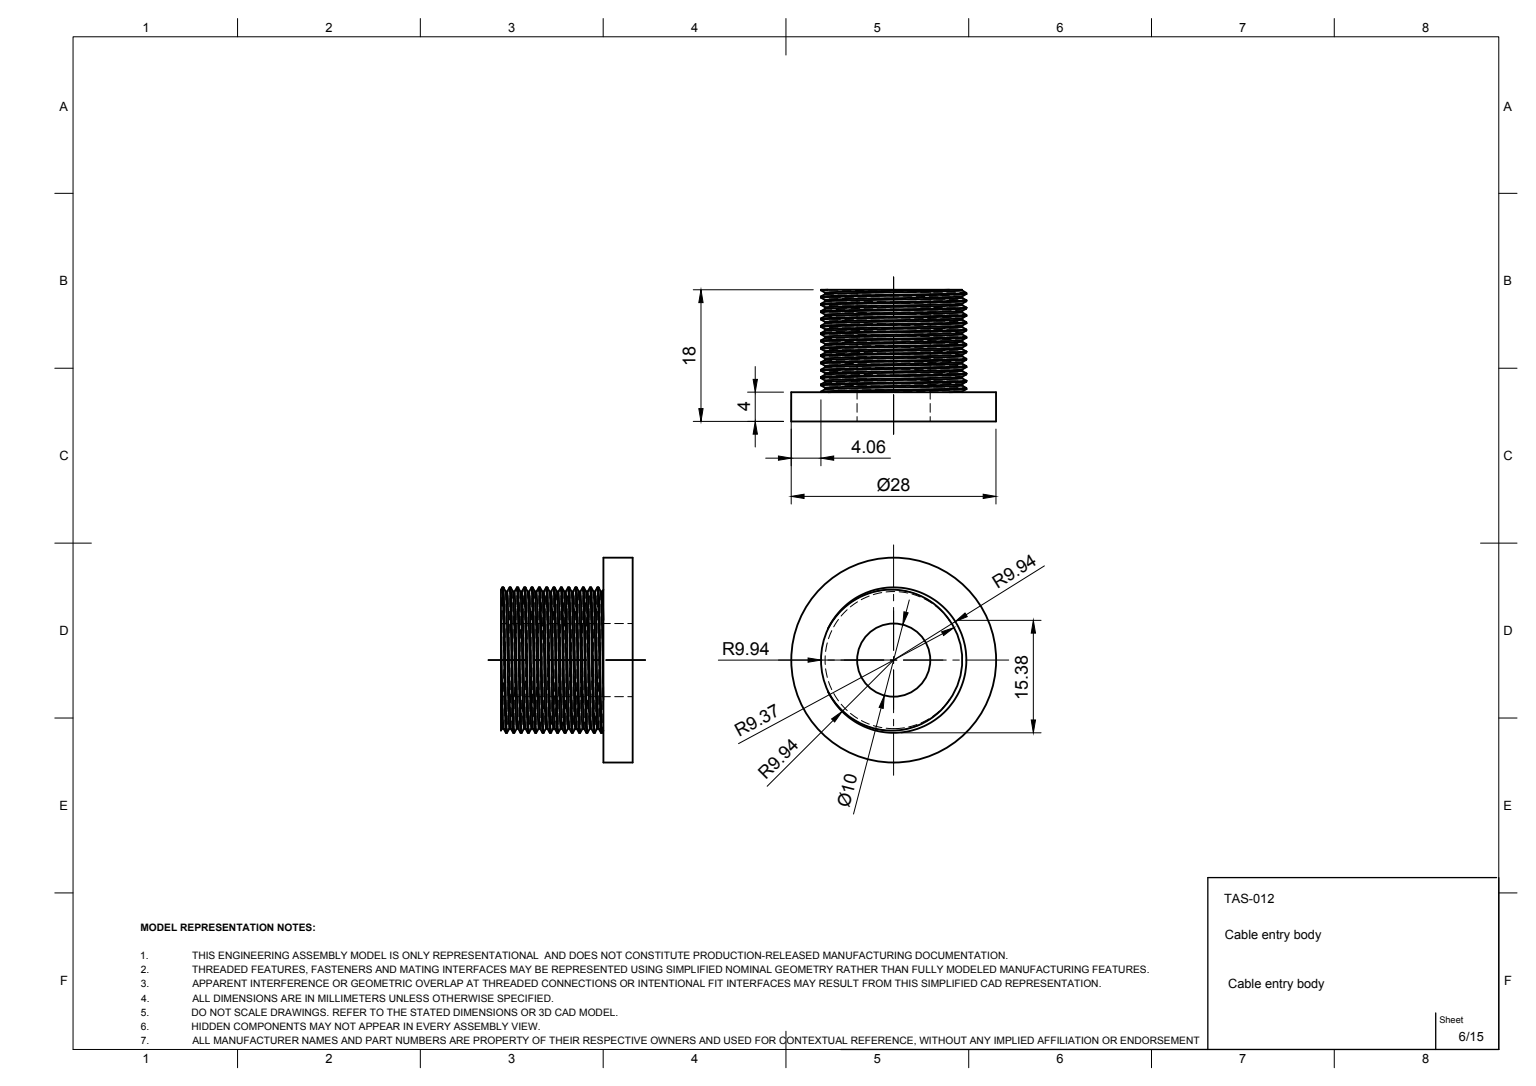
ISO-10303-21;
HEADER;
/* Generated by software containing ST-Developer
 * from STEP Tools, Inc. (www.steptools.com) 
 */

FILE_DESCRIPTION(
/* description */ (
'Independent welded steel electronics enclosure with removable sealed 
lid, internal mounting tray and two threaded cable entries. 300 x 220 
mm body. No ingress or electrical safety rating assigned.'),
/* implementation_level */ '2;1');

FILE_NAME(
/* name */ 'Cable entry body.step',
/* time_stamp */ '2026-11-14T09:13:27-08:00',
/* author */ (''),
/* organization */ (''),
/* preprocessor_version */ 'ST-DEVELOPER v20.2',
/* originating_system */ 'Autodesk Translation Framework v15.17.0.0',
/* authorisation */ '');

FILE_SCHEMA (('AUTOMOTIVE_DESIGN { 1 0 10303 214 3 1 1 }'));
ENDSEC;

DATA;
#10=MECHANICAL_DESIGN_GEOMETRIC_PRESENTATION_REPRESENTATION('',(#978),#94412);
#166=B_SPLINE_SURFACE_WITH_KNOTS('',3,3,((#89566,#89567,#89568,#89569,#89570,
#89571,#89572,#89573,#89574,#89575,#89576,#89577,#89578,#89579,#89580,#89581,
#89582,#89583,#89584,#89585,#89586,#89587,#89588,#89589,#89590,#89591,#89592,
#89593,#89594,#89595,#89596,#89597,#89598,#89599,#89600,#89601,#89602,#89603,
#89604,#89605,#89606,#89607,#89608,#89609,#89610,#89611,#89612,#89613,#89614,
#89615,#89616,#89617,#89618,#89619,#89620,#89621,#89622,#89623,#89624,#89625,
#89626,#89627,#89628,#89629,#89630,#89631,#89632,#89633,#89634,#89635,#89636,
#89637,#89638,#89639,#89640,#89641,#89642,#89643,#89644,#89645,#89646,#89647,
#89648,#89649,#89650,#89651,#89652,#89653,#89654,#89655,#89656,#89657,#89658,
#89659,#89660,#89661,#89662,#89663,#89664,#89665,#89666,#89667,#89668,#89669,
#89670,#89671,#89672,#89673,#89674,#89675,#89676,#89677,#89678,#89679,#89680,
#89681,#89682,#89683,#89684,#89685,#89686,#89687,#89688,#89689,#89690,#89691,
#89692,#89693,#89694,#89695,#89696,#89697,#89698,#89699,#89700,#89701,#89702,
#89703,#89704,#89705,#89706,#89707,#89708,#89709,#89710,#89711,#89712,#89713,
#89714,#89715,#89716,#89717,#89718,#89719,#89720,#89721,#89722,#89723,#89724,
#89725,#89726,#89727,#89728,#89729,#89730,#89731,#89732,#89733,#89734,#89735,
#89736,#89737,#89738,#89739,#89740,#89741,#89742,#89743,#89744,#89745,#89746,
#89747,#89748,#89749,#89750),(#89751,#89752,#89753,#89754,#89755,#89756,
#89757,#89758,#89759,#89760,#89761,#89762,#89763,#89764,#89765,#89766,#89767,
#89768,#89769,#89770,#89771,#89772,#89773,#89774,#89775,#89776,#89777,#89778,
#89779,#89780,#89781,#89782,#89783,#89784,#89785,#89786,#89787,#89788,#89789,
#89790,#89791,#89792,#89793,#89794,#89795,#89796,#89797,#89798,#89799,#89800,
#89801,#89802,#89803,#89804,#89805,#89806,#89807,#89808,#89809,#89810,#89811,
#89812,#89813,#89814,#89815,#89816,#89817,#89818,#89819,#89820,#89821,#89822,
#89823,#89824,#89825,#89826,#89827,#89828,#89829,#89830,#89831,#89832,#89833,
#89834,#89835,#89836,#89837,#89838,#89839,#89840,#89841,#89842,#89843,#89844,
#89845,#89846,#89847,#89848,#89849,#89850,#89851,#89852,#89853,#89854,#89855,
#89856,#89857,#89858,#89859,#89860,#89861,#89862,#89863,#89864,#89865,#89866,
#89867,#89868,#89869,#89870,#89871,#89872,#89873,#89874,#89875,#89876,#89877,
#89878,#89879,#89880,#89881,#89882,#89883,#89884,#89885,#89886,#89887,#89888,
#89889,#89890,#89891,#89892,#89893,#89894,#89895,#89896,#89897,#89898,#89899,
#89900,#89901,#89902,#89903,#89904,#89905,#89906,#89907,#89908,#89909,#89910,
#89911,#89912,#89913,#89914,#89915,#89916,#89917,#89918,#89919,#89920,#89921,
#89922,#89923,#89924,#89925,#89926,#89927,#89928,#89929,#89930,#89931,#89932,
#89933,#89934,#89935),(#89936,#89937,#89938,#89939,#89940,#89941,#89942,
#89943,#89944,#89945,#89946,#89947,#89948,#89949,#89950,#89951,#89952,#89953,
#89954,#89955,#89956,#89957,#89958,#89959,#89960,#89961,#89962,#89963,#89964,
#89965,#89966,#89967,#89968,#89969,#89970,#89971,#89972,#89973,#89974,#89975,
#89976,#89977,#89978,#89979,#89980,#89981,#89982,#89983,#89984,#89985,#89986,
#89987,#89988,#89989,#89990,#89991,#89992,#89993,#89994,#89995,#89996,#89997,
#89998,#89999,#90000,#90001,#90002,#90003,#90004,#90005,#90006,#90007,#90008,
#90009,#90010,#90011,#90012,#90013,#90014,#90015,#90016,#90017,#90018,#90019,
#90020,#90021,#90022,#90023,#90024,#90025,#90026,#90027,#90028,#90029,#90030,
#90031,#90032,#90033,#90034,#90035,#90036,#90037,#90038,#90039,#90040,#90041,
#90042,#90043,#90044,#90045,#90046,#90047,#90048,#90049,#90050,#90051,#90052,
#90053,#90054,#90055,#90056,#90057,#90058,#90059,#90060,#90061,#90062,#90063,
#90064,#90065,#90066,#90067,#90068,#90069,#90070,#90071,#90072,#90073,#90074,
#90075,#90076,#90077,#90078,#90079,#90080,#90081,#90082,#90083,#90084,#90085,
#90086,#90087,#90088,#90089,#90090,#90091,#90092,#90093,#90094,#90095,#90096,
#90097,#90098,#90099,#90100,#90101,#90102,#90103,#90104,#90105,#90106,#90107,
#90108,#90109,#90110,#90111,#90112,#90113,#90114,#90115,#90116,#90117,#90118,
#90119,#90120),(#90121,#90122,#90123,#90124,#90125,#90126,#90127,#90128,
#90129,#90130,#90131,#90132,#90133,#90134,#90135,#90136,#90137,#90138,#90139,
#90140,#90141,#90142,#90143,#90144,#90145,#90146,#90147,#90148,#90149,#90150,
#90151,#90152,#90153,#90154,#90155,#90156,#90157,#90158,#90159,#90160,#90161,
#90162,#90163,#90164,#90165,#90166,#90167,#90168,#90169,#90170,#90171,#90172,
#90173,#90174,#90175,#90176,#90177,#90178,#90179,#90180,#90181,#90182,#90183,
#90184,#90185,#90186,#90187,#90188,#90189,#90190,#90191,#90192,#90193,#90194,
#90195,#90196,#90197,#90198,#90199,#90200,#90201,#90202,#90203,#90204,#90205,
#90206,#90207,#90208,#90209,#90210,#90211,#90212,#90213,#90214,#90215,#90216,
#90217,#90218,#90219,#90220,#90221,#90222,#90223,#90224,#90225,#90226,#90227,
#90228,#90229,#90230,#90231,#90232,#90233,#90234,#90235,#90236,#90237,#90238,
#90239,#90240,#90241,#90242,#90243,#90244,#90245,#90246,#90247,#90248,#90249,
#90250,#90251,#90252,#90253,#90254,#90255,#90256,#90257,#90258,#90259,#90260,
#90261,#90262,#90263,#90264,#90265,#90266,#90267,#90268,#90269,#90270,#90271,
#90272,#90273,#90274,#90275,#90276,#90277,#90278,#90279,#90280,#90281,#90282,
#90283,#90284,#90285,#90286,#90287,#90288,#90289,#90290,#90291,#90292,#90293,
#90294,#90295,#90296,#90297,#90298,#90299,#90300,#90301,#90302,#90303,#90304,
#90305)),.UNSPECIFIED.,.F.,.F.,.F.,(4,4),(4,1,1,1,1,1,1,1,1,1,1,1,1,1,1,
1,1,1,1,1,1,1,1,1,1,1,1,1,1,1,1,1,1,1,1,1,1,1,1,1,1,1,1,1,1,1,1,1,1,1,1,
1,1,1,1,1,1,1,1,1,1,1,1,1,1,1,1,1,1,1,1,1,1,1,1,1,1,1,1,1,1,1,1,1,1,1,1,
1,1,1,1,1,1,1,1,1,1,1,1,1,1,1,1,1,1,1,1,1,1,1,1,1,1,1,1,1,1,1,1,1,1,1,1,
1,1,1,1,1,1,1,1,1,1,1,1,1,1,1,1,1,1,1,1,1,1,1,1,1,1,1,1,1,1,1,1,1,1,1,1,
1,1,1,1,1,1,1,1,1,1,1,1,1,1,1,1,1,1,1,1,1,1,1,4),(-0.000109569828534403,
0.0660914630517642),(8.30203615430833,8.79675414262435,9.29147213094037,
9.78619011925639,10.2809081075724,10.7756260958884,11.2703440842045,11.7650620725205,
12.2597800608365,12.7544980491525,13.2492160374685,13.7439340257846,14.2386520141006,
14.7333700024166,15.2280879907326,15.7228059790487,16.2175239673647,16.7122419556807,
17.2069599439967,17.7016779323128,18.1963959206288,18.6911139089448,19.1858318972608,
19.6805498855768,20.1752678738929,20.6699858622089,21.1647038505249,21.6594218388409,
22.1541398271569,22.648857815473,23.143575803789,23.638293792105,24.133011780421,
24.6277297687371,25.1224477570531,25.6171657453691,26.1118837336851,26.6066017220011,
27.1013197103172,27.5960376986332,28.0907556869492,28.5854736752652,29.0801916635813,
29.5749096518973,30.0696276402133,30.5643456285293,31.0590636168453,31.5537816051614,
32.0484995934774,32.5432175817934,33.0379355701094,33.5326535584255,34.0273715467415,
34.5220895350575,35.0168075233735,35.5115255116895,36.0062435000056,36.5009614883216,
36.9956794766376,37.4903974649536,37.9851154532697,38.4798334415857,38.9745514299017,
39.4692694182177,39.9639874065337,40.4587053948498,40.9534233831658,41.4481413714818,
41.9428593597978,42.4375773481139,42.9322953364299,43.4270133247459,43.9217313130619,
44.416449301378,44.911167289694,45.40588527801,45.900603266326,46.395321254642,
46.8900392429581,47.3847572312741,47.8794752195901,48.3741932079061,48.8689111962221,
49.3636291845382,49.8583471728542,50.3530651611702,50.8477831494862,51.3425011378023,
51.8372191261183,52.3319371144343,52.8266551027503,53.3213730910663,53.8160910793824,
54.3108090676984,54.8055270560144,55.3002450443304,55.7949630326465,56.2896810209625,
56.7843990092785,57.2791169975945,57.7738349859105,58.2685529742266,58.7632709625426,
59.2579889508586,59.7527069391746,60.2474249274907,60.7421429158067,61.2368609041227,
61.7315788924387,62.2262968807547,62.7210148690708,63.2157328573868,63.7104508457028,
64.2051688340188,64.6998868223349,65.1946048106509,65.6893227989669,66.1840407872829,
66.678758775599,67.173476763915,67.668194752231,68.162912740547,68.657630728863,
69.1523487171791,69.6470667054951,70.1417846938111,70.6365026821271,71.1312206704432,
71.6259386587592,72.1206566470752,72.6153746353912,73.1100926237072,73.6048106120233,
74.0995286003393,74.5942465886553,75.0889645769713,75.5836825652873,76.0784005536034,
76.5731185419194,77.0678365302354,77.5625545185514,78.0572725068675,78.5519904951835,
79.0467084834995,79.5414264718155,80.0361444601315,80.5308624484476,81.0255804367636,
81.5202984250796,82.0150164133956,82.5097344017117,83.0044523900277,83.4991703783437,
83.9938883666597,84.4886063549757,84.9833243432918,85.4780423316078,85.9727603199238,
86.4674783082398,86.9621962965559,87.4569142848719,87.9516322731879,88.4463502615039,
88.9410682498199,89.435786238136,89.930504226452,90.425222214768,90.919940203084,
91.4146581914001,91.9093761797161,92.4040941680321,92.8988121563481,93.3935301446641,
93.8882481329802,94.3829661212962,94.8776841096122,95.3724020979282,95.8671200862443,
96.3618380745603,96.8565560628763,97.3512740511923,97.8459920395083,98.3408195976529),
 .UNSPECIFIED.);
#167=B_SPLINE_SURFACE_WITH_KNOTS('',3,3,((#90545,#90546,#90547,#90548,#90549,
#90550,#90551,#90552,#90553,#90554,#90555,#90556,#90557,#90558,#90559,#90560,
#90561,#90562,#90563,#90564,#90565,#90566,#90567,#90568,#90569,#90570,#90571,
#90572,#90573,#90574,#90575,#90576,#90577,#90578,#90579,#90580,#90581,#90582,
#90583,#90584,#90585,#90586,#90587,#90588,#90589,#90590,#90591,#90592,#90593,
#90594,#90595,#90596,#90597,#90598,#90599,#90600,#90601,#90602,#90603,#90604,
#90605,#90606,#90607,#90608,#90609,#90610,#90611,#90612,#90613,#90614,#90615,
#90616,#90617,#90618,#90619,#90620,#90621,#90622,#90623,#90624,#90625,#90626,
#90627,#90628,#90629,#90630,#90631,#90632,#90633,#90634,#90635,#90636,#90637,
#90638,#90639,#90640,#90641,#90642,#90643,#90644,#90645,#90646,#90647,#90648,
#90649,#90650,#90651,#90652,#90653,#90654,#90655,#90656,#90657,#90658,#90659,
#90660,#90661,#90662,#90663,#90664,#90665,#90666,#90667,#90668,#90669,#90670,
#90671,#90672,#90673,#90674,#90675,#90676,#90677,#90678,#90679,#90680,#90681,
#90682,#90683,#90684,#90685,#90686,#90687,#90688,#90689,#90690,#90691,#90692,
#90693,#90694,#90695,#90696,#90697,#90698,#90699,#90700,#90701,#90702,#90703,
#90704,#90705,#90706,#90707,#90708,#90709,#90710,#90711,#90712,#90713,#90714,
#90715,#90716,#90717,#90718,#90719,#90720,#90721,#90722,#90723,#90724,#90725,
#90726,#90727,#90728,#90729),(#90730,#90731,#90732,#90733,#90734,#90735,
#90736,#90737,#90738,#90739,#90740,#90741,#90742,#90743,#90744,#90745,#90746,
#90747,#90748,#90749,#90750,#90751,#90752,#90753,#90754,#90755,#90756,#90757,
#90758,#90759,#90760,#90761,#90762,#90763,#90764,#90765,#90766,#90767,#90768,
#90769,#90770,#90771,#90772,#90773,#90774,#90775,#90776,#90777,#90778,#90779,
#90780,#90781,#90782,#90783,#90784,#90785,#90786,#90787,#90788,#90789,#90790,
#90791,#90792,#90793,#90794,#90795,#90796,#90797,#90798,#90799,#90800,#90801,
#90802,#90803,#90804,#90805,#90806,#90807,#90808,#90809,#90810,#90811,#90812,
#90813,#90814,#90815,#90816,#90817,#90818,#90819,#90820,#90821,#90822,#90823,
#90824,#90825,#90826,#90827,#90828,#90829,#90830,#90831,#90832,#90833,#90834,
#90835,#90836,#90837,#90838,#90839,#90840,#90841,#90842,#90843,#90844,#90845,
#90846,#90847,#90848,#90849,#90850,#90851,#90852,#90853,#90854,#90855,#90856,
#90857,#90858,#90859,#90860,#90861,#90862,#90863,#90864,#90865,#90866,#90867,
#90868,#90869,#90870,#90871,#90872,#90873,#90874,#90875,#90876,#90877,#90878,
#90879,#90880,#90881,#90882,#90883,#90884,#90885,#90886,#90887,#90888,#90889,
#90890,#90891,#90892,#90893,#90894,#90895,#90896,#90897,#90898,#90899,#90900,
#90901,#90902,#90903,#90904,#90905,#90906,#90907,#90908,#90909,#90910,#90911,
#90912,#90913,#90914),(#90915,#90916,#90917,#90918,#90919,#90920,#90921,
#90922,#90923,#90924,#90925,#90926,#90927,#90928,#90929,#90930,#90931,#90932,
#90933,#90934,#90935,#90936,#90937,#90938,#90939,#90940,#90941,#90942,#90943,
#90944,#90945,#90946,#90947,#90948,#90949,#90950,#90951,#90952,#90953,#90954,
#90955,#90956,#90957,#90958,#90959,#90960,#90961,#90962,#90963,#90964,#90965,
#90966,#90967,#90968,#90969,#90970,#90971,#90972,#90973,#90974,#90975,#90976,
#90977,#90978,#90979,#90980,#90981,#90982,#90983,#90984,#90985,#90986,#90987,
#90988,#90989,#90990,#90991,#90992,#90993,#90994,#90995,#90996,#90997,#90998,
#90999,#91000,#91001,#91002,#91003,#91004,#91005,#91006,#91007,#91008,#91009,
#91010,#91011,#91012,#91013,#91014,#91015,#91016,#91017,#91018,#91019,#91020,
#91021,#91022,#91023,#91024,#91025,#91026,#91027,#91028,#91029,#91030,#91031,
#91032,#91033,#91034,#91035,#91036,#91037,#91038,#91039,#91040,#91041,#91042,
#91043,#91044,#91045,#91046,#91047,#91048,#91049,#91050,#91051,#91052,#91053,
#91054,#91055,#91056,#91057,#91058,#91059,#91060,#91061,#91062,#91063,#91064,
#91065,#91066,#91067,#91068,#91069,#91070,#91071,#91072,#91073,#91074,#91075,
#91076,#91077,#91078,#91079,#91080,#91081,#91082,#91083,#91084,#91085,#91086,
#91087,#91088,#91089,#91090,#91091,#91092,#91093,#91094,#91095,#91096,#91097,
#91098,#91099),(#91100,#91101,#91102,#91103,#91104,#91105,#91106,#91107,
#91108,#91109,#91110,#91111,#91112,#91113,#91114,#91115,#91116,#91117,#91118,
#91119,#91120,#91121,#91122,#91123,#91124,#91125,#91126,#91127,#91128,#91129,
#91130,#91131,#91132,#91133,#91134,#91135,#91136,#91137,#91138,#91139,#91140,
#91141,#91142,#91143,#91144,#91145,#91146,#91147,#91148,#91149,#91150,#91151,
#91152,#91153,#91154,#91155,#91156,#91157,#91158,#91159,#91160,#91161,#91162,
#91163,#91164,#91165,#91166,#91167,#91168,#91169,#91170,#91171,#91172,#91173,
#91174,#91175,#91176,#91177,#91178,#91179,#91180,#91181,#91182,#91183,#91184,
#91185,#91186,#91187,#91188,#91189,#91190,#91191,#91192,#91193,#91194,#91195,
#91196,#91197,#91198,#91199,#91200,#91201,#91202,#91203,#91204,#91205,#91206,
#91207,#91208,#91209,#91210,#91211,#91212,#91213,#91214,#91215,#91216,#91217,
#91218,#91219,#91220,#91221,#91222,#91223,#91224,#91225,#91226,#91227,#91228,
#91229,#91230,#91231,#91232,#91233,#91234,#91235,#91236,#91237,#91238,#91239,
#91240,#91241,#91242,#91243,#91244,#91245,#91246,#91247,#91248,#91249,#91250,
#91251,#91252,#91253,#91254,#91255,#91256,#91257,#91258,#91259,#91260,#91261,
#91262,#91263,#91264,#91265,#91266,#91267,#91268,#91269,#91270,#91271,#91272,
#91273,#91274,#91275,#91276,#91277,#91278,#91279,#91280,#91281,#91282,#91283,
#91284)),.UNSPECIFIED.,.F.,.F.,.F.,(4,4),(4,1,1,1,1,1,1,1,1,1,1,1,1,1,1,
1,1,1,1,1,1,1,1,1,1,1,1,1,1,1,1,1,1,1,1,1,1,1,1,1,1,1,1,1,1,1,1,1,1,1,1,
1,1,1,1,1,1,1,1,1,1,1,1,1,1,1,1,1,1,1,1,1,1,1,1,1,1,1,1,1,1,1,1,1,1,1,1,
1,1,1,1,1,1,1,1,1,1,1,1,1,1,1,1,1,1,1,1,1,1,1,1,1,1,1,1,1,1,1,1,1,1,1,1,
1,1,1,1,1,1,1,1,1,1,1,1,1,1,1,1,1,1,1,1,1,1,1,1,1,1,1,1,1,1,1,1,1,1,1,1,
1,1,1,1,1,1,1,1,1,1,1,1,1,1,1,1,1,1,1,1,1,1,1,4),(-7.16819172715052E-5,
0.0661295621106345),(11.6149232889894,12.1097508361343,12.6044688244503,
13.0991868127663,13.5939048010823,14.0886227893984,14.5833407777144,15.0780587660304,
15.5727767543464,16.0674947426624,16.5622127309785,17.0569307192945,17.5516487076105,
18.0463666959265,18.5410846842426,19.0358026725586,19.5305206608746,20.0252386491906,
20.5199566375066,21.0146746258227,21.5093926141387,22.0041106024547,22.4988285907707,
22.9935465790868,23.4882645674028,23.9829825557188,24.4777005440348,24.9724185323508,
25.4671365206669,25.9618545089829,26.4565724972989,26.9512904856149,27.446008473931,
27.940726462247,28.435444450563,28.930162438879,29.424880427195,29.9195984155111,
30.4143164038271,30.9090343921431,31.4037523804591,31.8984703687752,32.3931883570912,
32.8879063454072,33.3826243337232,33.8773423220393,34.3720603103553,34.8667782986713,
35.3614962869873,35.8562142753033,36.3509322636194,36.8456502519354,37.3403682402514,
37.8350862285674,38.3298042168834,38.8245222051995,39.3192401935155,39.8139581818315,
40.3086761701475,40.8033941584636,41.2981121467796,41.7928301350956,42.2875481234116,
42.7822661117277,43.2769841000437,43.7717020883597,44.2664200766757,44.7611380649917,
45.2558560533078,45.7505740416238,46.2452920299398,46.7400100182558,47.2347280065719,
47.7294459948879,48.2241639832039,48.7188819715199,49.2135999598359,49.708317948152,
50.203035936468,50.697753924784,51.1924719131,51.6871899014161,52.1819078897321,
52.6766258780481,53.1713438663641,53.6660618546801,54.1607798429962,54.6554978313122,
55.1502158196282,55.6449338079442,56.1396517962603,56.6343697845763,57.1290877728923,
57.6238057612083,58.1185237495243,58.6132417378404,59.1079597261564,59.6026777144724,
60.0973957027884,60.5921136911045,61.0868316794205,61.5815496677365,62.0762676560525,
62.5709856443685,63.0657036326846,63.5604216210006,64.0551396093166,64.5498575976326,
65.0445755859486,65.5392935742647,66.0340115625807,66.5287295508967,67.0234475392127,
67.5181655275288,68.0128835158448,68.5076015041608,69.0023194924768,69.4970374807929,
69.9917554691089,70.4864734574249,70.9811914457409,71.4759094340569,71.970627422373,
72.465345410689,72.960063399005,73.454781387321,73.9494993756371,74.4442173639531,
74.9389353522691,75.4336533405851,75.9283713289011,76.4230893172172,76.9178073055332,
77.4125252938492,77.9072432821652,78.4019612704813,78.8966792587973,79.3913972471133,
79.8861152354293,80.3808332237453,80.8755512120614,81.3702692003774,81.8649871886934,
82.3597051770094,82.8544231653255,83.3491411536415,83.8438591419575,84.3385771302735,
84.8332951185895,85.3280131069056,85.8227310952216,86.3174490835376,86.8121670718536,
87.3068850601697,87.8016030484857,88.2963210368017,88.7910390251177,89.2857570134337,
89.7804750017498,90.2751929900658,90.7699109783818,91.2646289666978,91.7593469550139,
92.2540649433299,92.7487829316459,93.2435009199619,93.7382189082779,94.232936896594,
94.72765488491,95.222372873226,95.717090861542,96.2118088498581,96.7065268381741,
97.2012448264901,97.6959628148061,98.1906808031221,98.6853987914382,99.1801167797542,
99.6748347680702,100.169552756386,100.664270744702,101.158988733018,101.653706721334),
 .UNSPECIFIED.);
#820=B_SPLINE_CURVE_WITH_KNOTS('',3,(#79159,#79160,#79161,#79162,#79163,
#79164,#79165,#79166,#79167,#79168,#79169,#79170,#79171,#79172,#79173,#79174,
#79175,#79176,#79177,#79178,#79179,#79180,#79181,#79182,#79183,#79184,#79185,
#79186,#79187,#79188,#79189,#79190,#79191,#79192,#79193,#79194,#79195,#79196,
#79197,#79198,#79199,#79200,#79201,#79202,#79203,#79204,#79205,#79206,#79207,
#79208,#79209,#79210,#79211,#79212,#79213,#79214,#79215,#79216,#79217,#79218,
#79219,#79220,#79221,#79222,#79223,#79224,#79225,#79226,#79227,#79228,#79229,
#79230,#79231,#79232,#79233,#79234,#79235,#79236,#79237,#79238,#79239,#79240,
#79241,#79242,#79243,#79244,#79245,#79246,#79247,#79248,#79249,#79250,#79251,
#79252,#79253,#79254,#79255,#79256,#79257,#79258,#79259,#79260,#79261,#79262,
#79263,#79264,#79265,#79266,#79267,#79268,#79269,#79270,#79271,#79272,#79273,
#79274,#79275,#79276,#79277,#79278,#79279,#79280,#79281,#79282,#79283,#79284,
#79285,#79286,#79287,#79288,#79289,#79290,#79291,#79292,#79293,#79294,#79295,
#79296,#79297,#79298,#79299,#79300),.UNSPECIFIED.,.F.,.F.,(4,3,3,3,3,3,
3,3,3,3,3,3,3,3,3,3,3,3,3,3,3,3,3,3,3,3,3,3,3,3,3,3,3,3,3,3,3,3,3,3,3,3,
3,3,3,3,3,4),(10.3761157660455,10.4506267934108,10.5251285903801,10.5996351081557,
10.6741416414348,10.7486637991409,10.7756260958884,10.8504232250368,10.9252072529087,
10.9999831359438,11.074764867993,11.1495458255052,11.224342920955,11.2703440842045,
11.345139615213,11.4199219903501,11.494696171193,11.5694761383234,11.6442552982486,
11.719050557087,11.7650620725205,11.8398643668488,11.9146536010829,11.9894347157191,
12.064221679377,12.1390078597512,12.2138101295199,12.2597800608365,12.3345766451278,
12.409360096945,12.4841353745425,12.5589164609149,12.6336967509814,12.7084931494411,
12.7544980491525,12.8292980165575,12.9040848916852,12.9788636222862,13.0536481814959,
13.1284319498564,13.2032318119081,13.2492160374685,13.3240137948197,13.3987981794526,
13.4735800434188,13.5483567240136,13.6231416482335,13.6614849715988),
 .UNSPECIFIED.);
#821=B_SPLINE_CURVE_WITH_KNOTS('',3,(#79303,#79304,#79305,#79306,#79307,
#79308,#79309,#79310,#79311,#79312,#79313,#79314,#79315,#79316,#79317,#79318,
#79319,#79320,#79321,#79322,#79323,#79324,#79325,#79326,#79327,#79328,#79329,
#79330,#79331,#79332,#79333,#79334,#79335,#79336,#79337,#79338,#79339,#79340,
#79341,#79342,#79343,#79344,#79345,#79346,#79347,#79348,#79349,#79350,#79351,
#79352,#79353,#79354,#79355,#79356,#79357,#79358,#79359,#79360,#79361,#79362,
#79363,#79364,#79365,#79366,#79367,#79368,#79369,#79370,#79371,#79372,#79373,
#79374,#79375,#79376,#79377,#79378,#79379,#79380,#79381,#79382,#79383,#79384,
#79385,#79386,#79387,#79388,#79389,#79390),.UNSPECIFIED.,.F.,.F.,(4,3,3,
3,3,3,3,3,3,3,3,3,3,3,3,3,3,3,3,3,3,3,3,3,3,3,3,3,3,4),(11.6150328478182,
11.6902644851111,11.765490800086,11.8407152603781,11.915951572411,11.9911896602386,
12.0664446325848,12.1097508361343,12.1843206348914,12.2588742437492,12.3334173056347,
12.4079642286108,12.4825096216488,12.5570715231469,12.6044688244503,12.6793948372725,
12.7543093202956,12.8292168206913,12.9041309543681,12.9790445298975,13.0539736854477,
13.0991868127663,13.1739291377348,13.2486577313256,13.3233777185475,13.3981032598866,
13.4728279518355,13.5475690389764,13.5939048010823,13.6615138258512),
 .UNSPECIFIED.);
#822=B_SPLINE_CURVE_WITH_KNOTS('',3,(#79396,#79397,#79398,#79399,#79400,
#79401,#79402,#79403,#79404,#79405,#79406,#79407,#79408,#79409,#79410,#79411,
#79412,#79413,#79414,#79415,#79416,#79417,#79418,#79419,#79420,#79421,#79422,
#79423,#79424,#79425,#79426,#79427,#79428,#79429,#79430,#79431,#79432,#79433,
#79434,#79435,#79436,#79437,#79438,#79439,#79440,#79441,#79442,#79443,#79444,
#79445,#79446,#79447,#79448,#79449,#79450,#79451,#79452,#79453,#79454,#79455,
#79456,#79457,#79458,#79459,#79460,#79461,#79462,#79463,#79464,#79465,#79466,
#79467,#79468,#79469,#79470,#79471,#79472,#79473,#79474,#79475,#79476,#79477,
#79478,#79479,#79480,#79481,#79482,#79483,#79484,#79485,#79486,#79487,#79488,
#79489,#79490,#79491,#79492,#79493,#79494,#79495,#79496,#79497,#79498,#79499,
#79500,#79501,#79502,#79503,#79504,#79505,#79506,#79507,#79508,#79509,#79510,
#79511,#79512,#79513,#79514,#79515,#79516,#79517,#79518,#79519,#79520,#79521,
#79522,#79523,#79524,#79525,#79526,#79527,#79528,#79529,#79530,#79531,#79532,
#79533,#79534,#79535,#79536,#79537,#79538,#79539,#79540,#79541,#79542,#79543,
#79544,#79545,#79546,#79547,#79548,#79549,#79550,#79551,#79552,#79553,#79554,
#79555,#79556,#79557,#79558,#79559,#79560,#79561,#79562,#79563,#79564,#79565,
#79566,#79567,#79568,#79569,#79570,#79571,#79572,#79573,#79574,#79575,#79576,
#79577,#79578,#79579,#79580,#79581,#79582,#79583,#79584,#79585,#79586,#79587,
#79588,#79589,#79590,#79591,#79592,#79593,#79594,#79595,#79596,#79597),
 .UNSPECIFIED.,.F.,.F.,(4,2,2,2,2,2,2,2,2,2,2,2,2,2,2,2,2,2,2,2,2,2,2,2,
2,2,2,2,2,2,2,2,2,2,2,2,2,2,2,2,2,2,2,2,2,2,2,2,2,2,2,2,2,2,2,2,2,2,2,2,
2,2,2,2,2,2,2,2,2,2,2,2,2,2,2,2,2,2,2,2,2,2,2,2,2,2,2,2,2,2,2,2,2,2,2,2,
2,2,2,2,4),(-3.97109063192392,-3.9649584214025,-3.94125537962466,-3.91058322495257,
-3.89203316749827,-3.84035677009342,-3.74824131557227,-3.73197860427002,
-3.71922584434786,-3.7030726518714,-3.65804376908474,-3.52982073441756,
-3.50151446932462,-3.47782076935689,-3.4473215548278,-3.41239070554766,
-3.33572477575311,-3.28181642319089,-3.26520322651505,-3.25253604022651,
-3.23404990159059,-3.16534005368315,-3.07245755536263,-3.04222784660332,
-3.01852003999537,-2.99040223435899,-2.92206615278128,-2.82216886043237,
-2.80355774413339,-2.79088364704611,-2.77406349559966,-2.71944855650011,
-2.60247397040471,-2.57415598977363,-2.55046311454246,-2.51997956828078,
-2.4850754427358,-2.40855380420268,-2.35454076431744,-2.33788289742667,
-2.3252186833505,-2.30679093405412,-2.23683808586572,-2.14563298851787,
-2.11519033019849,-2.09146875015941,-2.0635047653402,-1.99725335964054,
-1.92544579474782,-1.88783821260595,-1.87222481097903,-1.85935818272856,
-1.83875150547172,-1.81194280557731,-1.73607218751607,-1.67481226399478,
-1.64659832981041,-1.62289804626951,-1.5922742192944,-1.57376850668018,
-1.52228771650205,-1.42937494715888,-1.41329236281721,-1.40056336817996,
-1.38425485370735,-1.33736129887648,-1.23960749036547,-1.19865388794307,
-1.17365645574888,-1.14883914487401,-1.10910255959279,-1.05646920957979,
-0.965000054988304,-0.949200763425442,-0.936504180056433,-0.919932085860634,
-0.869443816545504,-0.752738157034909,-0.722675470641795,-0.699000369934617,
-0.673666991491305,-0.664833626055923,-0.649423893463878,-0.601283018334735,
-0.502106716811277,-0.484581341103242,-0.47641641941256,-0.464785993756397,
-0.449891830642469,-0.436902619345004,-0.358101489383389,-0.286795121484024,
-0.257554411525978,-0.233892389125443,-0.211223048857578,-0.156660280482908,
-0.0839224513368464,-0.0354159956040736,-0.0191828792016435,-0.00973861638456724,
-0.000140069715062154),.UNSPECIFIED.);
#823=B_SPLINE_CURVE_WITH_KNOTS('',3,(#79598,#79599,#79600,#79601,#79602,
#79603,#79604,#79605,#79606,#79607,#79608,#79609,#79610,#79611,#79612,#79613,
#79614,#79615,#79616,#79617,#79618,#79619,#79620,#79621,#79622,#79623,#79624,
#79625,#79626,#79627,#79628,#79629,#79630,#79631,#79632,#79633,#79634,#79635,
#79636,#79637,#79638,#79639,#79640,#79641,#79642,#79643,#79644,#79645,#79646,
#79647,#79648,#79649,#79650,#79651,#79652,#79653,#79654,#79655,#79656,#79657,
#79658,#79659,#79660,#79661,#79662,#79663,#79664,#79665,#79666,#79667,#79668,
#79669,#79670,#79671,#79672,#79673,#79674,#79675,#79676,#79677,#79678,#79679,
#79680,#79681,#79682,#79683,#79684,#79685,#79686,#79687,#79688),
 .UNSPECIFIED.,.F.,.F.,(4,3,3,3,3,3,3,3,3,3,3,3,3,3,3,3,3,3,3,3,3,3,3,3,
3,3,3,3,3,3,4),(13.6614849715988,13.7362826754358,13.7439340257846,13.8187329504215,
13.8935187704987,13.9682964370049,14.0430799261714,14.1178626229009,14.1926614179982,
14.2386520141006,14.3134508885949,14.3882366586011,14.4630142752602,14.5377977152858,
14.6125803633574,14.6873791108762,14.7333700024166,14.8081687869976,14.882954465705,
14.9577319899606,15.0325153365808,15.1072978908342,15.1820965445166,15.2280879907326,
15.302789587196,15.3774777760568,15.4521578013161,15.5268433257792,15.6015287495532,
15.6762295160124,15.7079632678645),.UNSPECIFIED.);
#824=B_SPLINE_CURVE_WITH_KNOTS('',3,(#79690,#79691,#79692,#79693,#79694,
#79695,#79696,#79697,#79698,#79699,#79700,#79701,#79702,#79703,#79704,#79705,
#79706,#79707,#79708,#79709,#79710,#79711,#79712,#79713,#79714,#79715,#79716,
#79717,#79718,#79719,#79720,#79721,#79722,#79723,#79724,#79725,#79726,#79727,
#79728,#79729,#79730,#79731,#79732,#79733,#79734,#79735,#79736,#79737,#79738,
#79739,#79740,#79741,#79742,#79743,#79744,#79745,#79746,#79747,#79748,#79749,
#79750,#79751,#79752,#79753,#79754,#79755,#79756,#79757,#79758,#79759,#79760,
#79761,#79762,#79763,#79764,#79765,#79766,#79767,#79768,#79769,#79770,#79771,
#79772,#79773,#79774,#79775,#79776,#79777),.UNSPECIFIED.,.F.,.F.,(4,3,3,
3,3,3,3,3,3,3,3,3,3,3,3,3,3,3,3,3,3,3,3,3,3,3,3,3,3,4),(13.6615138258512,
13.7363191624509,13.8111159963363,13.8859184780869,13.9607196890201,14.0355373534483,
14.0886227893984,14.1634199053517,14.2382039199167,14.3129797895736,14.3877615082347,
14.4625424523753,14.5373395345686,14.5833407777144,14.6581363061753,14.7329186787134,
14.8076928569137,14.8824728213545,14.9572519785678,15.0320472346775,15.0780587660304,
15.1528610671284,15.2276503082195,15.302431429779,15.3772184004102,15.4520045877747,
15.5268068645131,15.5727767543464,15.650970727164,15.7079632679489),
 .UNSPECIFIED.);
#825=B_SPLINE_CURVE_WITH_KNOTS('',3,(#79778,#79779,#79780,#79781,#79782,
#79783,#79784,#79785,#79786,#79787,#79788,#79789),.UNSPECIFIED.,.F.,.F.,
(4,1,1,1,1,1,1,1,1,4),(15.7079632679489,16.0674947426624,16.5622127309785,
17.0569307192945,17.5516487076105,18.0463666959265,18.5410846842426,19.0358026725586,
19.5305206608746,19.9446639604968),.UNSPECIFIED.);
#826=B_SPLINE_CURVE_WITH_KNOTS('',3,(#79794,#79795,#79796,#79797,#79798,
#79799,#79800,#79801,#79802,#79803,#79804,#79805,#79806,#79807,#79808,#79809,
#79810,#79811,#79812,#79813,#79814,#79815,#79816,#79817,#79818,#79819,#79820,
#79821,#79822,#79823,#79824,#79825,#79826,#79827,#79828,#79829,#79830,#79831,
#79832,#79833,#79834,#79835,#79836,#79837,#79838,#79839,#79840,#79841,#79842,
#79843,#79844,#79845,#79846,#79847,#79848,#79849,#79850,#79851,#79852,#79853,
#79854,#79855,#79856,#79857,#79858,#79859,#79860,#79861,#79862,#79863,#79864,
#79865,#79866,#79867,#79868,#79869,#79870,#79871,#79872,#79873,#79874,#79875,
#79876,#79877,#79878,#79879,#79880,#79881,#79882,#79883,#79884,#79885,#79886,
#79887,#79888,#79889,#79890,#79891,#79892,#79893,#79894,#79895,#79896,#79897,
#79898,#79899,#79900,#79901,#79902,#79903,#79904,#79905,#79906,#79907,#79908,
#79909,#79910,#79911,#79912,#79913,#79914,#79915,#79916,#79917,#79918,#79919,
#79920,#79921,#79922,#79923,#79924,#79925,#79926,#79927,#79928,#79929,#79930,
#79931,#79932,#79933,#79934,#79935,#79936,#79937,#79938,#79939,#79940,#79941,
#79942,#79943,#79944,#79945,#79946,#79947,#79948,#79949,#79950,#79951,#79952,
#79953,#79954,#79955,#79956,#79957,#79958,#79959,#79960,#79961,#79962,#79963,
#79964,#79965,#79966,#79967,#79968,#79969,#79970,#79971,#79972,#79973,#79974,
#79975,#79976,#79977,#79978,#79979,#79980,#79981,#79982,#79983,#79984,#79985,
#79986,#79987,#79988,#79989,#79990,#79991,#79992,#79993,#79994,#79995,#79996,
#79997,#79998,#79999,#80000,#80001,#80002,#80003,#80004,#80005,#80006,#80007,
#80008,#80009,#80010,#80011,#80012,#80013,#80014,#80015,#80016,#80017,#80018,
#80019,#80020,#80021,#80022,#80023,#80024,#80025,#80026,#80027,#80028,#80029,
#80030,#80031,#80032,#80033,#80034,#80035,#80036,#80037,#80038,#80039,#80040,
#80041,#80042,#80043,#80044,#80045,#80046,#80047,#80048,#80049,#80050,#80051,
#80052,#80053,#80054,#80055,#80056,#80057,#80058,#80059,#80060,#80061,#80062,
#80063,#80064,#80065,#80066,#80067,#80068,#80069,#80070,#80071,#80072,#80073,
#80074,#80075,#80076,#80077,#80078,#80079,#80080,#80081,#80082,#80083,#80084,
#80085,#80086,#80087,#80088,#80089,#80090,#80091,#80092,#80093,#80094,#80095,
#80096,#80097,#80098,#80099,#80100,#80101),.UNSPECIFIED.,.F.,.F.,(4,2,2,
2,2,2,2,2,2,2,2,2,2,2,2,2,2,2,2,2,2,2,2,2,2,2,2,2,2,2,2,2,2,2,2,2,2,2,2,
2,2,2,2,2,2,2,2,2,2,2,2,2,2,2,2,2,2,2,2,2,2,2,2,2,2,2,2,2,2,2,2,2,2,2,2,
2,2,2,2,2,2,2,2,2,2,2,2,2,2,2,2,2,2,2,2,2,2,2,2,2,2,2,2,2,2,2,2,2,2,2,2,
2,2,2,2,2,2,2,2,2,2,2,2,2,2,2,2,2,2,2,2,2,2,2,2,2,2,2,2,2,2,2,2,2,2,2,2,
2,2,2,2,2,2,4),(-9.86013605182866,-9.85775592310744,-9.80120571927038,-9.78509274360098,
-9.76249470244743,-9.74934425532136,-9.73451575923864,-9.70134415794215,
-9.62845209064997,-9.55767673893976,-9.52939672097626,-9.50570105156311,
-9.47568485969833,-9.38097537979839,-9.33321054321053,-9.31169702354504,
-9.29405595272518,-9.28265001569269,-9.26623359882227,-9.21661344277033,
-9.13666290115609,-9.10114259414212,-9.07029916734766,-9.04658601691335,
-9.01852858927522,-8.89654998353862,-8.84560378324243,-8.8290011938466,
-8.81630761709997,-8.8005391354648,-8.70955394869662,-8.65661582770117,
-8.61674042232065,-8.59190236775481,-8.56692658301866,-8.52612083856455,
-8.42830549826841,-8.38123731803778,-8.3649147337912,-8.35218752366493,
-8.33612032199704,-8.24313778883039,-8.16742303449248,-8.13887189008925,
-8.11519192950506,-8.08500583940029,-7.98521965495371,-7.92449884912506,
-7.90501076512387,-7.8922684876077,-7.87604877900771,-7.83693885180086,
-7.7655751863258,-7.72118503160559,-7.68545871628982,-7.6612173431972,-7.63535576288555,
-7.58841906612945,-7.49441766873105,-7.47359980156074,-7.44683028829438,
-7.43298830831523,-7.41914254335625,-7.39235073028266,-7.28964779422958,
-7.25087949922825,-7.21818171589099,-7.19431121702325,-7.16732570321357,
-7.11144587243985,-7.02819044901947,-6.98844486983763,-6.97280647748618,
-6.95994613294143,-6.93939078254868,-6.88412961052176,-6.85306375000533,
-6.77649597594078,-6.74790554766224,-6.72422736167339,-6.69408941231124,
-6.59384716829753,-6.54927633205444,-6.52053385070342,-6.50636651372026,
-6.49448858324354,-6.47179765676272,-6.36363430158537,-6.32427069852211,
-6.29124106043262,-6.26733515011524,-6.24050357706787,-6.18597660025094,
-6.16949424205874,-6.09754507421765,-6.07916661576279,-6.06729844499258,
-6.0490075016292,-6.03634929855385,-6.01958334460289,-5.96547711678565,
-5.88919331281921,-5.84055104036619,-5.81445688424311,-5.79031754994828,
-5.75535671470574,-5.71242984849447,-5.64152711550889,-5.59920056388999,
-5.58285392158756,-5.5701300056767,-5.55084368472898,-5.53804144574276,
-5.45977517752814,-5.38672804378348,-5.35770365462632,-5.33403881488783,
-5.30440026965166,-5.27092874007404,-5.2016691711656,-5.19262313337488,
-5.13721349899873,-5.12033590631651,-5.10768281194952,-5.08952855945553,
-5.07778672957253,-5.05969028240922,-4.98987066092593,-4.96996673442988,
-4.91648815815063,-4.88953017159539,-4.86565349808146,-4.83289749484037,
-4.75387142711427,-4.67736449371335,-4.65855758971717,-4.64587098151835,
-4.62919627952934,-4.57711505794881,-4.45671660136064,-4.4285728621856,
-4.4048668683294,-4.37414531940268,-4.35554992977496,-4.30367308439143,
-4.28314416449104,-4.26293236475343,-4.21358916027192,-4.19482286021633,
-4.18213903445771,-4.16543487941048,-4.1128678875124,-3.99313738636478,
-3.97109063192392),.UNSPECIFIED.);
#827=B_SPLINE_CURVE_WITH_KNOTS('',3,(#80103,#80104,#80105,#80106,#80107,
#80108,#80109,#80110),.UNSPECIFIED.,.F.,.F.,(4,1,1,1,1,4),(19.9446639604968,
20.0252386491906,20.5199566375066,21.0146746258227,21.5093926141387,21.9911485575199),
 .UNSPECIFIED.);
#828=B_SPLINE_CURVE_WITH_KNOTS('',3,(#80111,#80112,#80113,#80114,#80115,
#80116,#80117,#80118,#80119,#80120,#80121,#80122,#80123,#80124,#80125,#80126,
#80127,#80128,#80129,#80130,#80131,#80132,#80133,#80134,#80135,#80136,#80137,
#80138,#80139,#80140,#80141,#80142,#80143,#80144,#80145,#80146,#80147,#80148,
#80149,#80150,#80151,#80152,#80153,#80154,#80155,#80156,#80157,#80158,#80159,
#80160,#80161,#80162,#80163,#80164,#80165,#80166,#80167,#80168,#80169,#80170,
#80171,#80172,#80173,#80174,#80175,#80176,#80177,#80178,#80179,#80180,#80181,
#80182,#80183,#80184,#80185,#80186,#80187,#80188,#80189,#80190,#80191,#80192,
#80193,#80194,#80195,#80196,#80197,#80198,#80199,#80200,#80201,#80202,#80203,
#80204,#80205,#80206,#80207,#80208,#80209,#80210,#80211,#80212,#80213,#80214,
#80215,#80216,#80217,#80218,#80219,#80220,#80221,#80222,#80223,#80224,#80225,
#80226,#80227,#80228,#80229,#80230,#80231,#80232,#80233,#80234,#80235,#80236,
#80237,#80238,#80239,#80240,#80241,#80242,#80243,#80244,#80245,#80246,#80247,
#80248,#80249,#80250,#80251,#80252,#80253,#80254,#80255,#80256,#80257,#80258,
#80259,#80260,#80261,#80262,#80263,#80264,#80265,#80266,#80267,#80268,#80269,
#80270,#80271,#80272,#80273,#80274,#80275,#80276,#80277,#80278,#80279,#80280,
#80281,#80282,#80283,#80284,#80285,#80286,#80287,#80288,#80289,#80290,#80291,
#80292,#80293,#80294,#80295,#80296,#80297,#80298,#80299,#80300,#80301,#80302,
#80303,#80304,#80305,#80306,#80307,#80308,#80309,#80310),.UNSPECIFIED.,
 .F.,.F.,(4,2,2,2,2,2,2,2,2,2,2,2,2,2,2,2,2,2,2,2,2,2,2,2,2,2,2,2,2,2,2,
2,2,2,2,2,2,2,2,2,2,2,2,2,2,2,2,2,2,2,2,2,2,2,2,2,2,2,2,2,2,2,2,2,2,2,2,
2,2,2,2,2,2,2,2,2,2,2,2,2,2,2,2,2,2,2,2,2,2,2,2,2,2,2,2,2,2,2,2,4),(-11.7781659429298,
-11.7695015011355,-11.7608648717293,-11.7446191234857,-11.6961485739992,
-11.6253310868354,-11.5693010683801,-11.546580909873,-11.5229169989328,
-11.4938896650299,-11.4207905883937,-11.3425572214838,-11.3297661630289,
-11.3149993089201,-11.3033988389499,-11.2945967762062,-11.27631395539,-11.1983463453215,
-11.13949459,-11.1168460665849,-11.1068983920934,-11.0813894076414,-11.0577201330965,
-11.0278361945305,-10.9092863261089,-10.8599661768067,-10.8434748824404,
-10.830769568392,-10.8117030092558,-10.757330661835,-10.6843363809635,-10.6501063763627,
-10.6200191075797,-10.5965648779771,-10.5680452639929,-10.4555779698413,
-10.3974659494186,-10.3804778821854,-10.3678152467337,-10.3494180968824,
-10.2636130824389,-10.1884160541029,-10.1575629366113,-10.1338495789973,
-10.1057997660604,-9.98369695884995,-9.93284204766808,-9.91624569593284,
-9.90355173584416,-9.88463638359643,-9.81037554518269,-9.7497025044728,
-9.7292453368533,-9.6965321207523,-9.6726603626042,-9.64568293025807,-9.58987219510691,
-9.50654307814477,-9.47869354785551,-9.45753575641754,-9.44459690261661,
-9.42923247726541,-9.39657756671605,-9.3238580101053,-9.2537602354624,-9.22552374854818,
-9.20182540347174,-9.17175387252392,-9.07754270399396,-9.00960384726125,
-8.99118342280821,-8.97851965180629,-8.96185630990279,-8.90783600130185,
-8.83133154849194,-8.79643098946603,-8.76594954274167,-8.74225692517295,
-8.71393769160619,-8.59699032178751,-8.54235438486408,-8.52553317220681,
-8.51285924140121,-8.49424976045908,-8.39900512355604,-8.3496835568728,
-8.31149720599506,-8.28690780339787,-8.26465669098099,-8.22564678861382,
-8.12025152888348,-8.07671557608262,-8.06069651088904,-8.04792037962756,
-8.03149393709917,-7.92656790738476,-7.86153813609482,-7.83367099818519,
-7.80993962364222,-7.80726529325742),.UNSPECIFIED.);
#829=B_SPLINE_CURVE_WITH_KNOTS('',3,(#80316,#80317,#80318,#80319,#80320,
#80321,#80322,#80323,#80324,#80325,#80326,#80327),.UNSPECIFIED.,.F.,.F.,
(4,1,1,1,1,1,1,1,1,4),(28.2743338823081,28.5854736752652,29.0801916635813,
29.5749096518973,30.0696276402133,30.5643456285293,31.0590636168453,31.5537816051614,
32.0484995934774,32.5110459440461),.UNSPECIFIED.);
#830=B_SPLINE_CURVE_WITH_KNOTS('',3,(#80328,#80329,#80330,#80331,#80332,
#80333,#80334,#80335,#80336,#80337,#80338,#80339,#80340,#80341,#80342,#80343,
#80344,#80345,#80346,#80347,#80348,#80349,#80350,#80351,#80352,#80353,#80354,
#80355,#80356,#80357,#80358,#80359,#80360,#80361,#80362,#80363,#80364,#80365,
#80366,#80367,#80368,#80369,#80370,#80371,#80372,#80373,#80374,#80375,#80376,
#80377,#80378,#80379,#80380,#80381,#80382,#80383,#80384,#80385,#80386,#80387,
#80388,#80389,#80390,#80391,#80392,#80393,#80394,#80395,#80396,#80397,#80398,
#80399,#80400,#80401,#80402,#80403,#80404,#80405,#80406,#80407,#80408,#80409,
#80410,#80411,#80412,#80413,#80414,#80415,#80416,#80417,#80418,#80419,#80420,
#80421,#80422,#80423,#80424,#80425,#80426,#80427,#80428,#80429,#80430,#80431,
#80432,#80433,#80434,#80435),.UNSPECIFIED.,.F.,.F.,(4,2,2,2,2,2,2,2,2,2,
2,2,2,2,2,2,2,2,2,2,2,2,2,2,2,2,2,2,2,2,2,2,2,2,2,2,2,2,2,2,2,2,2,2,2,2,
2,2,2,2,2,2,2,4),(-11.778252564853,-11.6406709475873,-11.6235349277419,
-11.6112523485181,-11.598568535928,-11.5798024599838,-11.5304636051125,
-11.5206877207964,-11.5075055668975,-11.445472516879,-11.4136118290732,
-11.3858150712362,-11.3629328315184,-11.3338397533264,-11.2579743756513,
-11.1949532381769,-11.1702611569884,-11.152796955343,-11.152515566578,-11.1520536549756,
-11.1513315226703,-11.150268370153,-11.1496141462943,-11.1369542046494,
-11.1202217431636,-11.0691368366197,-10.9907289590674,-10.9554812177169,
-10.924796590793,-10.9010927554962,-10.8729225884066,-10.7530181607851,
-10.7005758873345,-10.6838791394854,-10.6711945775082,-10.6555200921164,
-10.5636129805667,-10.4860973636492,-10.4574659762096,-10.4361630462076,
-10.4073916427012,-10.3366881833582,-10.2569399767523,-10.2293878667224,
-10.2154146117674,-10.2034293258265,-10.1800043676687,-10.0728753989478,
-10.0336200014843,-10.0006505217454,-9.97675121384317,-9.94989254594728,
-9.89513072885096,-9.86013605182866),.UNSPECIFIED.);
#831=B_SPLINE_CURVE_WITH_KNOTS('',3,(#80436,#80437,#80438,#80439,#80440,
#80441,#80442,#80443,#80444,#80445,#80446,#80447,#80448,#80449,#80450,#80451,
#80452,#80453,#80454,#80455,#80456,#80457,#80458,#80459,#80460,#80461,#80462,
#80463,#80464,#80465,#80466,#80467,#80468,#80469,#80470,#80471,#80472,#80473,
#80474,#80475,#80476,#80477,#80478,#80479,#80480,#80481,#80482,#80483,#80484,
#80485,#80486,#80487,#80488,#80489,#80490,#80491,#80492,#80493,#80494,#80495,
#80496,#80497,#80498,#80499,#80500,#80501,#80502,#80503,#80504,#80505,#80506,
#80507,#80508,#80509,#80510,#80511,#80512,#80513,#80514,#80515,#80516,#80517,
#80518,#80519,#80520,#80521,#80522,#80523,#80524,#80525,#80526,#80527,#80528,
#80529,#80530,#80531,#80532,#80533,#80534,#80535,#80536,#80537,#80538,#80539,
#80540,#80541,#80542,#80543,#80544,#80545,#80546,#80547,#80548,#80549,#80550,
#80551,#80552,#80553,#80554,#80555,#80556,#80557,#80558,#80559,#80560,#80561,
#80562,#80563,#80564,#80565,#80566,#80567,#80568,#80569,#80570,#80571,#80572,
#80573,#80574,#80575,#80576,#80577,#80578,#80579,#80580,#80581,#80582,#80583,
#80584,#80585,#80586,#80587,#80588,#80589,#80590,#80591,#80592,#80593,#80594,
#80595,#80596,#80597,#80598,#80599,#80600,#80601,#80602,#80603,#80604,#80605,
#80606,#80607,#80608,#80609,#80610,#80611,#80612,#80613,#80614,#80615,#80616,
#80617,#80618,#80619,#80620,#80621,#80622,#80623,#80624,#80625,#80626,#80627,
#80628,#80629,#80630,#80631,#80632,#80633,#80634,#80635,#80636,#80637,#80638,
#80639,#80640,#80641,#80642,#80643,#80644,#80645,#80646,#80647,#80648,#80649,
#80650,#80651,#80652,#80653,#80654,#80655,#80656,#80657,#80658,#80659,#80660,
#80661,#80662,#80663,#80664,#80665,#80666,#80667,#80668,#80669,#80670,#80671,
#80672,#80673,#80674,#80675,#80676,#80677,#80678,#80679,#80680,#80681,#80682,
#80683,#80684,#80685,#80686,#80687,#80688,#80689,#80690,#80691,#80692,#80693,
#80694,#80695,#80696,#80697,#80698,#80699,#80700,#80701,#80702,#80703,#80704,
#80705,#80706,#80707,#80708,#80709,#80710,#80711,#80712,#80713,#80714,#80715,
#80716,#80717,#80718,#80719,#80720,#80721,#80722,#80723,#80724,#80725,#80726,
#80727,#80728,#80729,#80730,#80731,#80732,#80733,#80734,#80735),
 .UNSPECIFIED.,.F.,.F.,(4,2,2,2,2,2,2,2,2,2,2,2,2,2,2,2,2,2,2,2,2,2,2,2,
2,2,2,2,2,2,2,2,2,2,2,2,2,2,2,2,2,2,2,2,2,2,2,2,2,2,2,2,2,2,2,2,2,2,2,2,
2,2,2,2,2,2,2,2,2,2,2,2,2,2,2,2,2,2,2,2,2,2,2,2,2,2,2,2,2,2,2,2,2,2,2,2,
2,2,2,2,2,2,2,2,2,2,2,2,2,2,2,2,2,2,2,2,2,2,2,2,2,2,2,2,2,2,2,2,2,2,2,2,
2,2,2,2,2,2,2,2,2,2,2,2,2,2,2,2,2,4),(-7.80726529325742,-7.77935749609294,
-7.67305087886337,-7.61532396084259,-7.59835246544215,-7.58568871944003,
-7.56727066738562,-7.47118503282339,-7.42209034280295,-7.38401311193093,
-7.35943952478874,-7.33717305143281,-7.29804852312495,-7.19964982003832,
-7.15047690409958,-7.13399591078041,-7.12128917107599,-7.10220677162885,
-7.04762646706141,-7.01303062849308,-6.96101782570722,-6.94239188993943,
-6.91163719378434,-6.88792947523917,-6.85980982007647,-6.73896706821418,
-6.68720740777731,-6.67055278508652,-6.65786440302101,-6.63903011343649,
-6.56284146877764,-6.48357197730743,-6.45081089598387,-6.42693388028032,
-6.39997866352125,-6.34652087598751,-6.32989519195407,-6.25758324449705,
-6.23131673594426,-6.21100128453345,-6.19817022235686,-6.18241309711473,
-6.14686954960281,-6.11611080039932,-6.04600090885001,-6.02380754583908,
-5.98930233089118,-5.96522178535301,-5.93897523237577,-5.88918110525131,
-5.80898148854834,-5.75967792345171,-5.74327726051686,-5.73187018921226,
-5.71420974715616,-5.6926632020871,-5.64475803048892,-5.55036136288458,
-5.52031075793103,-5.49661326915974,-5.46835998403671,-5.39800749783332,
-5.32522198340407,-5.29281571825591,-5.27749425283985,-5.26454117835684,
-5.24328084015127,-5.21523579186608,-5.13040125871549,-5.0759326908419,
-5.0491080994601,-5.02520070541903,-4.99215618326773,-4.95276549104083,
-4.84434110764955,-4.82183199912996,-4.80998016703858,-4.79576089979521,
-4.76669207336761,-4.6887629815646,-4.65102056503018,-4.60678762499012,
-4.58130911634682,-4.55685806621619,-4.51963156128297,-4.49466563782946,
-4.40554657926642,-4.36686138093599,-4.3510076779813,-4.33949694543313,
-4.32066136354435,-4.29707312666952,-4.23980418042955,-4.1963896853928,
-4.14646511054971,-4.12020136732982,-4.09612672528735,-4.06166971512036,
-4.0395240005844,-3.9696941780766,-3.92927284834963,-3.89911281573639,-3.8847234296745,
-3.87132508166856,-3.84718798128298,-3.723868174573,-3.67950966880563,-3.65401301968522,
-3.62957324258816,-3.59242578765454,-3.56754300871115,-3.47909488615639,
-3.44000695207153,-3.42395354489741,-3.41130481685074,-3.39166051011915,
-3.3295062352493,-3.23111223937331,-3.20106004713098,-3.17738496280548,
-3.14872381429807,-3.07048034386312,-2.97957200166355,-2.96382341457031,
-2.95113180129177,-2.93450944732577,-2.88325837040146,-2.76170931335911,
-2.73362826711275,-2.70991711376523,-2.67910727891974,-2.64364459968794,
-2.56402503823103,-2.51397747236937,-2.49754039088955,-2.48613588695837,
-2.46852001598447,-2.44704958953221,-2.3994666130595,-2.30436443440703,
-2.27439122337597,-2.2506977762483,-2.22238404925131,-2.15106455046269,
-2.05533442705832,-2.03644540328393,-2.02375314844008,-2.00713760892109,
-1.95599150686342,-1.91824501396425),.UNSPECIFIED.);
#832=B_SPLINE_CURVE_WITH_KNOTS('',3,(#80741,#80742,#80743,#80744,#80745,
#80746,#80747,#80748,#80749,#80750,#80751,#80752,#80753,#80754,#80755,#80756,
#80757,#80758,#80759,#80760,#80761,#80762,#80763,#80764,#80765,#80766,#80767,
#80768,#80769,#80770,#80771,#80772,#80773,#80774,#80775,#80776,#80777,#80778,
#80779,#80780,#80781,#80782,#80783,#80784,#80785,#80786,#80787,#80788,#80789,
#80790,#80791,#80792,#80793,#80794,#80795,#80796,#80797,#80798,#80799,#80800,
#80801,#80802,#80803,#80804,#80805,#80806,#80807,#80808,#80809,#80810,#80811,
#80812,#80813,#80814,#80815,#80816,#80817,#80818,#80819,#80820,#80821,#80822,
#80823,#80824,#80825,#80826,#80827,#80828,#80829,#80830,#80831,#80832,#80833,
#80834,#80835,#80836,#80837,#80838,#80839,#80840,#80841,#80842,#80843,#80844,
#80845,#80846,#80847,#80848,#80849,#80850,#80851,#80852,#80853,#80854,#80855,
#80856,#80857,#80858,#80859,#80860,#80861,#80862,#80863,#80864,#80865,#80866,
#80867,#80868,#80869,#80870,#80871,#80872,#80873,#80874,#80875,#80876,#80877,
#80878,#80879,#80880,#80881,#80882,#80883,#80884,#80885,#80886,#80887,#80888,
#80889,#80890,#80891,#80892,#80893,#80894,#80895,#80896,#80897,#80898,#80899,
#80900,#80901,#80902,#80903,#80904,#80905,#80906,#80907,#80908,#80909,#80910,
#80911,#80912,#80913,#80914,#80915,#80916,#80917,#80918,#80919,#80920,#80921,
#80922,#80923,#80924,#80925,#80926,#80927,#80928,#80929,#80930,#80931,#80932,
#80933,#80934),.UNSPECIFIED.,.F.,.F.,(4,2,2,2,2,2,2,2,2,2,2,2,2,2,2,2,2,
2,2,2,2,2,2,2,2,2,2,2,2,2,2,2,2,2,2,2,2,2,2,2,2,2,2,2,2,2,2,2,2,2,2,2,2,
2,2,2,2,2,2,2,2,2,2,2,2,2,2,2,2,2,2,2,2,2,2,2,2,2,2,2,2,2,2,2,2,2,2,2,2,
2,2,2,2,2,2,2,4),(-3.97117590885512,-3.94669210599682,-3.91832163603527,
-3.89463165039578,-3.86421585636958,-3.8294276465923,-3.7535305641743,-3.70095786973156,
-3.68480102203414,-3.67206237742609,-3.65581860712673,-3.60972342272422,
-3.48546404062927,-3.45625278551107,-3.43259021326658,-3.40314936400795,
-3.37001008928841,-3.30231304465889,-3.25471306968969,-3.22710654390848,
-3.21312430909366,-3.19941166328336,-3.17340453068049,-3.09590210320283,
-3.02140843908474,-2.99233187439596,-2.96866796824151,-2.93908586509719,
-2.85571691487168,-2.77465612436432,-2.75627897603085,-2.74361703761271,
-2.72661210030565,-2.66810690159166,-2.55612981204258,-2.52758977816173,
-2.50413606401613,-2.47407252071042,-2.38836528380176,-2.3118553058605,
-2.29304889556372,-2.28036241622853,-2.26368760924573,-2.21160285508002,
-2.09121087589847,-2.06306707946917,-2.03936130748535,-2.00864042433467,
-1.99004556608244,-1.93817082040966,-1.91785217331093,-1.89587697902556,
-1.84473820161903,-1.82916976320421,-1.81649459529526,-1.7996884101607,
-1.74533279986831,-1.62801440519616,-1.59971318465083,-1.576019203503,-1.54551343126094,
-1.45913347520987,-1.38469760991913,-1.365779818563,-1.35308564020557,-1.33649089694924,
-1.28566093199827,-1.16352397162026,-1.13547607916695,-1.11176242983227,
-1.08090624861425,-1.00568594923737,-0.919885438748811,-0.901498384786369,
-0.888836175204954,-0.871839799565827,-0.8135330797845,-0.701310851708188,
-0.672781243510081,-0.649327404532392,-0.62189163869072,-0.589287260920047,
-0.524022535056337,-0.457700442076925,-0.438593440647315,-0.426817530209833,
-0.411870657074917,-0.393914572892701,-0.375874474294829,-0.306470523602214,
-0.286747545038346,-0.232123890928064,-0.205281683836191,-0.182245325000184,
-0.158840728001359,-0.126585532836681,-0.000142354813690746),
 .UNSPECIFIED.);
#833=B_SPLINE_CURVE_WITH_KNOTS('',3,(#80935,#80936,#80937,#80938,#80939,
#80940,#80941,#80942,#80943),.UNSPECIFIED.,.F.,.F.,(4,1,1,1,1,1,4),(32.5110459440461,
32.5432175817934,33.0379355701094,33.5326535584255,34.0273715467415,34.5220895350575,
34.5575191894876),.UNSPECIFIED.);
#834=B_SPLINE_CURVE_WITH_KNOTS('',3,(#80945,#80946,#80947,#80948,#80949,
#80950,#80951,#80952,#80953,#80954,#80955,#80956,#80957,#80958,#80959,#80960,
#80961,#80962,#80963,#80964,#80965,#80966,#80967,#80968,#80969,#80970,#80971,
#80972,#80973,#80974,#80975,#80976,#80977,#80978,#80979,#80980,#80981,#80982,
#80983,#80984,#80985,#80986,#80987,#80988,#80989,#80990,#80991,#80992,#80993,
#80994,#80995,#80996,#80997,#80998,#80999,#81000,#81001,#81002,#81003,#81004,
#81005,#81006,#81007,#81008,#81009,#81010,#81011,#81012,#81013,#81014,#81015,
#81016,#81017,#81018,#81019,#81020,#81021,#81022,#81023,#81024,#81025,#81026,
#81027,#81028,#81029,#81030,#81031,#81032,#81033,#81034,#81035,#81036,#81037,
#81038,#81039,#81040,#81041,#81042,#81043,#81044,#81045,#81046,#81047,#81048,
#81049,#81050,#81051,#81052,#81053,#81054),.UNSPECIFIED.,.F.,.F.,(4,2,2,
2,2,2,2,2,2,2,2,2,2,2,2,2,2,2,2,2,2,2,2,2,2,2,2,2,2,2,2,2,2,2,2,2,2,2,2,
2,2,2,2,2,2,2,2,2,2,2,2,2,2,2,4),(-1.91824501396425,-1.8342962072515,-1.8062233370852,
-1.78251154726549,-1.75169024170491,-1.64528869417893,-1.59185174083218,
-1.572850276496,-1.5601497685894,-1.5436131796231,-1.49364886915071,-1.39509152131626,
-1.35654326121122,-1.33435343049951,-1.3096967027995,-1.27105115822649,
-1.24456381956939,-1.14148313179044,-1.11499221548568,-1.1011975431422,
-1.0873036587019,-1.06022641471589,-0.98116527554644,-0.909790542086502,
-0.88076198567875,-0.857097422887064,-0.827463893622975,-0.794000655713836,
-0.724779681140215,-0.716059543688041,-0.660156861263222,-0.64332592836881,
-0.630670960003319,-0.629780525361832,-0.628733844006517,-0.62803050250851,
-0.627587692028264,-0.627323204165017,-0.609917659297998,-0.585254988701595,
-0.522393448448096,-0.446313546842396,-0.417219738677862,-0.394335955943159,
-0.36653663262421,-0.334674406927403,-0.272634956591863,-0.259378025635748,
-0.23422814172291,-0.196144838492948,-0.179462759142269,-0.166799940165386,
-0.153984094128512,-0.135253108926845,-0.000139984804832171),
 .UNSPECIFIED.);
#835=B_SPLINE_CURVE_WITH_KNOTS('',3,(#81055,#81056,#81057,#81058,#81059,
#81060,#81061,#81062,#81063,#81064,#81065,#81066),.UNSPECIFIED.,.F.,.F.,
(4,1,1,1,1,1,1,1,1,4),(34.5575191894876,34.8667782986713,35.3614962869873,
35.8562142753033,36.3509322636194,36.8456502519354,37.3403682402514,37.8350862285674,
38.3298042168834,38.7942318298859),.UNSPECIFIED.);
#836=B_SPLINE_CURVE_WITH_KNOTS('',3,(#81071,#81072,#81073,#81074,#81075,
#81076,#81077,#81078,#81079,#81080,#81081,#81082,#81083,#81084,#81085,#81086,
#81087,#81088,#81089,#81090,#81091,#81092,#81093,#81094,#81095,#81096,#81097,
#81098,#81099,#81100,#81101,#81102,#81103,#81104,#81105,#81106,#81107,#81108,
#81109,#81110,#81111,#81112,#81113,#81114,#81115,#81116,#81117,#81118,#81119,
#81120,#81121,#81122,#81123,#81124,#81125,#81126,#81127,#81128,#81129,#81130,
#81131,#81132,#81133,#81134,#81135,#81136,#81137,#81138,#81139,#81140,#81141,
#81142,#81143,#81144,#81145,#81146,#81147,#81148,#81149,#81150,#81151,#81152,
#81153,#81154,#81155,#81156,#81157,#81158,#81159,#81160,#81161,#81162,#81163,
#81164,#81165,#81166,#81167,#81168,#81169,#81170,#81171,#81172,#81173,#81174,
#81175,#81176,#81177,#81178,#81179,#81180,#81181,#81182,#81183,#81184,#81185,
#81186,#81187,#81188,#81189,#81190,#81191,#81192,#81193,#81194,#81195,#81196,
#81197,#81198,#81199,#81200,#81201,#81202,#81203,#81204,#81205,#81206,#81207,
#81208,#81209,#81210,#81211,#81212,#81213,#81214,#81215,#81216,#81217,#81218,
#81219,#81220,#81221,#81222,#81223,#81224,#81225,#81226,#81227,#81228,#81229,
#81230,#81231,#81232,#81233,#81234,#81235,#81236,#81237,#81238,#81239,#81240,
#81241,#81242,#81243,#81244,#81245,#81246,#81247,#81248,#81249,#81250,#81251,
#81252,#81253,#81254,#81255,#81256,#81257,#81258,#81259,#81260,#81261,#81262,
#81263,#81264,#81265,#81266,#81267,#81268,#81269,#81270,#81271,#81272,#81273,
#81274,#81275,#81276,#81277,#81278,#81279,#81280,#81281,#81282,#81283,#81284,
#81285,#81286,#81287,#81288,#81289,#81290,#81291,#81292,#81293,#81294,#81295,
#81296,#81297,#81298,#81299,#81300,#81301,#81302,#81303,#81304,#81305,#81306,
#81307,#81308,#81309,#81310,#81311,#81312,#81313,#81314,#81315,#81316,#81317,
#81318,#81319,#81320,#81321,#81322,#81323,#81324,#81325,#81326,#81327,#81328,
#81329,#81330,#81331,#81332,#81333,#81334,#81335,#81336,#81337,#81338,#81339,
#81340,#81341,#81342,#81343,#81344,#81345,#81346,#81347,#81348,#81349,#81350,
#81351,#81352,#81353,#81354,#81355,#81356,#81357,#81358,#81359,#81360,#81361,
#81362,#81363,#81364,#81365,#81366,#81367,#81368),.UNSPECIFIED.,.F.,.F.,
(4,2,2,2,2,2,2,2,2,2,2,2,2,2,2,2,2,2,2,2,2,2,2,2,2,2,2,2,2,2,2,2,2,2,2,
2,2,2,2,2,2,2,2,2,2,2,2,2,2,2,2,2,2,2,2,2,2,2,2,2,2,2,2,2,2,2,2,2,2,2,2,
2,2,2,2,2,2,2,2,2,2,2,2,2,2,2,2,2,2,2,2,2,2,2,2,2,2,2,2,2,2,2,2,2,2,2,2,
2,2,2,2,2,2,2,2,2,2,2,2,2,2,2,2,2,2,2,2,2,2,2,2,2,2,2,2,2,2,2,2,2,2,2,2,
2,2,2,2,2,4),(-9.86033244913055,-9.77739253699707,-9.72608805652884,-9.70946221456373,
-9.69677094322151,-9.67789630566169,-9.58370404394948,-9.53411900141677,
-9.4958060569039,-9.47119783710931,-9.44896361531342,-9.41008279524055,
-9.31161175459176,-9.26210699274753,-9.24560223454247,-9.2328980318875,
-9.21384994916835,-9.15973800623508,-9.0865412548556,-9.05227082661466,
-9.02215941597697,-8.99870349725517,-8.97020186124062,-8.91993015267223,
-8.83613964537186,-8.80822929074451,-8.78703944730677,-8.77409598781925,
-8.75874466618789,-8.72616719264965,-8.71460591101003,-8.64361178224165,
-8.58131395590594,-8.55368052872497,-8.52992100104272,-8.49898199278193,
-8.41371278870625,-8.36129776720617,-8.33872740203133,-8.32047261013326,
-8.30781587696831,-8.29102083704401,-8.23690113026724,-8.22576947493894,
-8.15689905032915,-8.12350961599345,-8.09391980192682,-8.07025570510155,
-8.04118613511597,-7.96727658597128,-7.91431314121214,-7.87005969786478,
-7.85397490925657,-7.84121039815357,-7.82486478496651,-7.73961184116769,
-7.66314229947051,-7.63230474640208,-7.60859179350799,-7.58052989993121,
-7.45862679723594,-7.40762576420864,-7.39101949292255,-7.37832618291459,
-7.36256119343595,-7.27146810243856,-7.21858318283746,-7.17873180614436,
-7.15389716371441,-7.12891735908514,-7.08808541847225,-6.99027954696925,
-6.94324135847825,-6.92692105665543,-6.91419341668011,-6.89812340003582,
-6.80515230070911,-6.75368581940515,-6.73518324516962,-6.70456260377428,
-6.6808620763586,-6.65264484757364,-6.53363498250119,-6.48053465728852,
-6.463798708702,-6.45111745010716,-6.4354809092715,-6.34385213485923,-6.27122998973946,
-6.2407010657508,-6.21700532389978,-6.1887201022444,-6.07105406488286,-6.01695397039558,
-6.00016133534451,-5.98748472432999,-5.96883638058315,-5.88932349350522,
-5.85688907718263,-5.7996625413613,-5.77186850167902,-5.74835431386524,
-5.71726481319648,-5.64013499651377,-5.5561899478352,-5.53983783589433,
-5.52707224812301,-5.51099234058698,-5.46679473976078,-5.40816786213515,
-5.39720969879808,-5.33637019363306,-5.30845410012555,-5.28472697569694,
-5.25367452506697,-5.23477430860724,-5.18153367420624,-5.09224079483206,
-5.07600190110426,-5.06325217333186,-5.04707826682177,-5.00181284160679,
-4.87419332313879,-4.84578181499333,-4.82209415948423,-4.79173118246769,
-4.7570330918028,-4.68161596568595,-4.62656862638144,-4.6096571361798,-4.59700524646752,
-4.57889121193606,-4.56718649646222,-4.54917257720713,-4.47996380352212,
-4.46032468063247,-4.40545256047621,-4.37858099181817,-4.35468437146394,
-4.3217420755776,-4.30106674047401,-4.23928386116105,-4.22927950101439,
-4.16785287070975,-4.14845555875556,-4.13572163212356,-4.11944533935889,
-4.07295488621113,-3.97117590885512),.UNSPECIFIED.);
#837=B_SPLINE_CURVE_WITH_KNOTS('',3,(#81370,#81371,#81372,#81373,#81374,
#81375,#81376,#81377,#81378),.UNSPECIFIED.,.F.,.F.,(4,1,1,1,1,1,4),(38.7942318298859,
38.8245222051995,39.3192401935155,39.8139581818315,40.3086761701475,40.8033941584636,
40.8407044966672),.UNSPECIFIED.);
#838=B_SPLINE_CURVE_WITH_KNOTS('',3,(#81379,#81380,#81381,#81382,#81383,
#81384,#81385,#81386,#81387,#81388,#81389,#81390,#81391,#81392,#81393,#81394,
#81395,#81396,#81397,#81398,#81399,#81400,#81401,#81402,#81403,#81404,#81405,
#81406,#81407,#81408,#81409,#81410,#81411,#81412,#81413,#81414,#81415,#81416,
#81417,#81418,#81419,#81420,#81421,#81422,#81423,#81424,#81425,#81426,#81427,
#81428,#81429,#81430,#81431,#81432,#81433,#81434,#81435,#81436,#81437,#81438,
#81439,#81440,#81441,#81442,#81443,#81444,#81445,#81446,#81447,#81448,#81449,
#81450,#81451,#81452,#81453,#81454,#81455,#81456,#81457,#81458,#81459,#81460,
#81461,#81462,#81463,#81464,#81465,#81466,#81467,#81468,#81469,#81470,#81471,
#81472,#81473,#81474,#81475,#81476,#81477,#81478,#81479,#81480,#81481,#81482,
#81483,#81484,#81485,#81486,#81487,#81488,#81489,#81490,#81491,#81492,#81493,
#81494,#81495,#81496,#81497,#81498,#81499,#81500,#81501,#81502,#81503,#81504,
#81505,#81506,#81507,#81508,#81509,#81510,#81511,#81512,#81513,#81514,#81515,
#81516,#81517,#81518,#81519,#81520,#81521,#81522,#81523,#81524,#81525,#81526,
#81527,#81528,#81529,#81530,#81531,#81532,#81533,#81534,#81535,#81536,#81537,
#81538,#81539,#81540,#81541,#81542,#81543,#81544,#81545,#81546,#81547,#81548,
#81549,#81550,#81551,#81552,#81553,#81554,#81555,#81556,#81557,#81558,#81559,
#81560,#81561,#81562,#81563,#81564,#81565,#81566,#81567,#81568,#81569,#81570,
#81571,#81572,#81573,#81574,#81575,#81576,#81577,#81578,#81579,#81580,#81581,
#81582,#81583,#81584),.UNSPECIFIED.,.F.,.F.,(4,2,2,2,2,2,2,2,2,2,2,2,2,
2,2,2,2,2,2,2,2,2,2,2,2,2,2,2,2,2,2,2,2,2,2,2,2,2,2,2,2,2,2,2,2,2,2,2,2,
2,2,2,2,2,2,2,2,2,2,2,2,2,2,2,2,2,2,2,2,2,2,2,2,2,2,2,2,2,2,2,2,2,2,2,2,
2,2,2,2,2,2,2,2,2,2,2,2,2,2,2,2,2,4),(-11.7781831743828,-11.6260661591714,
-11.6017687512626,-11.5793373662868,-11.5539682497423,-11.5104874491002,
-11.4117913943339,-11.3821460219622,-11.365635591246,-11.3568105796511,
-11.3448291022619,-11.3284934608432,-11.2832616135781,-11.2097913377315,
-11.1693775682343,-11.1378568324822,-11.1343972580855,-11.1114130120227,
-11.0846875885037,-11.0310599347158,-11.0142787233368,-10.9415863014961,
-10.9152604997613,-10.8949131518813,-10.8820784311998,-10.8663378351426,
-10.8303263626715,-10.7390074721489,-10.7137762171665,-10.6762987149449,
-10.6518120688465,-10.6294573281325,-10.5896720157373,-10.4914848761713,
-10.4431744763155,-10.4267566561111,-10.4140423728019,-10.3948660301994,
-10.3303755979629,-10.2640571819278,-10.2312187377213,-10.2019574387005,
-10.1782955211556,-10.1489069072841,-10.025056066204,-9.97904025569186,
-9.96280326709271,-9.9500638566959,-9.93389977234738,-9.84134158836594,
-9.78977879127754,-9.77125454352334,-9.74061054432852,-9.71690924558964,
-9.68871022344481,-9.56202468271073,-9.51544944811176,-9.49916648734847,
-9.48643380623231,-9.47032222349466,-9.37754625099469,-9.32603165477186,
-9.30751829735652,-9.27688610265486,-9.25318533589026,-9.22497743715288,
-9.16377067687952,-9.08784253829277,-9.06102515672551,-9.04041388539968,
-9.02754667261904,-9.0119354141544,-8.97443421784928,-8.90261099926778,
-8.83628479849076,-8.80831510907377,-8.78459403637256,-8.75415933515382,
-8.66289066274043,-8.59341019005958,-8.57477704409865,-8.56328836775181,
-8.54730785134841,-8.5062499668104,-8.43507091744583,-8.39124270955568,
-8.35580860507305,-8.33160692971632,-8.30566037143869,-8.25810507985645,
-8.21190747541639,-8.15402958371029,-8.13031948200305,-8.11141517262278,
-8.09989680431939,-8.08408519176954,-8.04553184658872,-7.97394355569426,
-7.90868877073898,-7.88080345692803,-7.85707400606071,-7.8265184254936,
-7.80724139219308),.UNSPECIFIED.);
#839=B_SPLINE_CURVE_WITH_KNOTS('',3,(#81590,#81591,#81592,#81593,#81594,
#81595,#81596,#81597,#81598,#81599,#81600,#81601,#81602),.UNSPECIFIED.,
 .F.,.F.,(4,1,1,1,1,1,1,1,1,1,4),(47.1238898038468,47.3847572312741,47.8794752195901,
48.3741932079061,48.8689111962221,49.3636291845382,49.8583471728542,50.3530651611702,
50.8477831494862,51.3425011378023,51.3606186663471),.UNSPECIFIED.);
#840=B_SPLINE_CURVE_WITH_KNOTS('',3,(#81603,#81604,#81605,#81606,#81607,
#81608,#81609,#81610,#81611,#81612,#81613,#81614,#81615,#81616,#81617,#81618,
#81619,#81620,#81621,#81622,#81623,#81624,#81625,#81626,#81627,#81628,#81629,
#81630,#81631,#81632,#81633,#81634,#81635,#81636,#81637,#81638,#81639,#81640,
#81641,#81642,#81643,#81644,#81645,#81646,#81647,#81648,#81649,#81650,#81651,
#81652,#81653,#81654,#81655,#81656,#81657,#81658,#81659,#81660,#81661,#81662,
#81663,#81664,#81665,#81666,#81667,#81668,#81669,#81670,#81671,#81672,#81673,
#81674,#81675,#81676,#81677,#81678,#81679,#81680,#81681,#81682,#81683,#81684,
#81685,#81686,#81687,#81688,#81689,#81690,#81691,#81692,#81693,#81694,#81695,
#81696,#81697,#81698,#81699,#81700,#81701,#81702),.UNSPECIFIED.,.F.,.F.,
(4,2,2,2,2,2,2,2,2,2,2,2,2,2,2,2,2,2,2,2,2,2,2,2,2,2,2,2,2,2,2,2,2,2,2,
2,2,2,2,2,2,2,2,2,2,2,2,2,2,4),(-11.7784366611071,-11.7628329720818,-11.7438991398111,
-11.6731931297632,-11.5857198879355,-11.5712330140719,-11.5596933549217,
-11.5477413454121,-11.5245409275816,-11.429055081479,-11.3974403810343,
-11.3770429577357,-11.3465365156196,-11.3239349171576,-11.2987398156749,
-11.2552837584844,-11.157740113712,-11.1282150063576,-11.1117428477294,
-11.0996706976597,-11.0868939480905,-11.0704638980195,-10.9731801343212,
-10.9019065435147,-10.8735957935129,-10.8499022671194,-10.8199255897818,
-10.724853489267,-10.6772553015051,-10.6557812424994,-10.6381633068063,
-10.6267587391384,-10.6103235151704,-10.5603129861121,-10.4806667080049,
-10.4451996306652,-10.4143872066649,-10.3906759963909,-10.362597003124,
-10.2410084683321,-10.1897840972919,-10.1731634678615,-10.1604717404985,
-10.1415899762254,-10.0660389719386,-9.98146986987404,-9.95066607423389,
-9.92695529116087,-9.89887002508965,-9.86033244913055),.UNSPECIFIED.);
#841=B_SPLINE_CURVE_WITH_KNOTS('',3,(#81703,#81704,#81705,#81706,#81707,
#81708,#81709,#81710,#81711,#81712,#81713,#81714,#81715,#81716,#81717,#81718,
#81719,#81720,#81721,#81722,#81723,#81724,#81725,#81726,#81727,#81728,#81729,
#81730,#81731,#81732,#81733,#81734,#81735,#81736,#81737,#81738,#81739,#81740,
#81741,#81742,#81743,#81744,#81745,#81746,#81747,#81748,#81749,#81750,#81751,
#81752,#81753,#81754,#81755,#81756,#81757,#81758,#81759,#81760,#81761,#81762,
#81763,#81764,#81765,#81766,#81767,#81768,#81769,#81770,#81771,#81772,#81773,
#81774,#81775,#81776,#81777,#81778,#81779,#81780,#81781,#81782,#81783,#81784,
#81785,#81786,#81787,#81788,#81789,#81790,#81791,#81792,#81793,#81794,#81795,
#81796,#81797,#81798,#81799,#81800,#81801,#81802,#81803,#81804,#81805,#81806,
#81807,#81808,#81809,#81810,#81811,#81812,#81813,#81814,#81815,#81816,#81817,
#81818,#81819,#81820,#81821,#81822,#81823,#81824,#81825,#81826,#81827,#81828,
#81829,#81830,#81831,#81832,#81833,#81834,#81835,#81836,#81837,#81838,#81839,
#81840,#81841,#81842,#81843,#81844,#81845,#81846,#81847,#81848,#81849,#81850,
#81851,#81852,#81853,#81854,#81855,#81856,#81857,#81858,#81859,#81860,#81861,
#81862,#81863,#81864,#81865,#81866,#81867,#81868,#81869,#81870,#81871,#81872,
#81873,#81874,#81875,#81876,#81877,#81878,#81879,#81880,#81881,#81882,#81883,
#81884,#81885,#81886,#81887,#81888,#81889,#81890,#81891,#81892,#81893,#81894,
#81895,#81896,#81897,#81898,#81899,#81900,#81901,#81902,#81903,#81904,#81905,
#81906,#81907,#81908,#81909,#81910,#81911,#81912,#81913,#81914,#81915,#81916,
#81917,#81918,#81919,#81920,#81921,#81922,#81923,#81924,#81925,#81926,#81927,
#81928,#81929,#81930,#81931,#81932,#81933,#81934,#81935,#81936,#81937,#81938,
#81939,#81940,#81941,#81942,#81943,#81944,#81945,#81946,#81947,#81948,#81949,
#81950,#81951,#81952,#81953,#81954,#81955,#81956,#81957,#81958,#81959,#81960,
#81961,#81962,#81963,#81964,#81965,#81966,#81967,#81968,#81969,#81970,#81971,
#81972,#81973,#81974,#81975,#81976,#81977,#81978,#81979,#81980,#81981,#81982,
#81983,#81984,#81985,#81986,#81987,#81988,#81989,#81990,#81991,#81992,#81993,
#81994),.UNSPECIFIED.,.F.,.F.,(4,2,2,2,2,2,2,2,2,2,2,2,2,2,2,2,2,2,2,2,
2,2,2,2,2,2,2,2,2,2,2,2,2,2,2,2,2,2,2,2,2,2,2,2,2,2,2,2,2,2,2,2,2,2,2,2,
2,2,2,2,2,2,2,2,2,2,2,2,2,2,2,2,2,2,2,2,2,2,2,2,2,2,2,2,2,2,2,2,2,2,2,2,
2,2,2,2,2,2,2,2,2,2,2,2,2,2,2,2,2,2,2,2,2,2,2,2,2,2,2,2,2,2,2,2,2,2,2,2,
2,2,2,2,2,2,2,2,2,2,2,2,2,2,2,2,2,4),(-7.80724139219308,-7.71981411584434,
-7.66238540670509,-7.64542715140195,-7.63276260216355,-7.61432806879973,
-7.51902370635884,-7.46954082116731,-7.43127702730007,-7.40667626901852,
-7.38443574036619,-7.34550564743403,-7.24705048558355,-7.19761483203255,
-7.18111515690178,-7.16841058865532,-7.14935567740324,-7.09514549910357,
-7.06013174301192,-7.00811444826017,-6.98948750202281,-6.95873170878801,
-6.93502392881301,-6.90690505996573,-6.78604788650302,-6.73429865586456,
-6.71764468902357,-6.7049562462725,-6.68612105310803,-6.60994322166724,
-6.52663647899754,-6.49554504837585,-6.4718157252893,-6.44392648958552,
-6.38310357438839,-6.30610461156731,-6.28709356693267,-6.26185675755588,
-6.248274504511,-6.23413839171721,-6.20558963652288,-6.08739629825127,-6.06691649875384,
-6.03417942648747,-6.01030504049926,-5.9833386803844,-5.92762805862817,
-5.9085270784957,-5.88912162087633,-5.8114649031761,-5.79277306680576,-5.78009411540398,
-5.76333503166283,-5.70982622853529,-5.59289502256792,-5.56414726593092,
-5.54284402610689,-5.51418991434288,-5.43611253566099,-5.34507201881703,
-5.32930315830641,-5.31660970274705,-5.30000788713656,-5.24906994341387,
-5.12708537128809,-5.09902902657562,-5.07531612920752,-5.04447208400203,
-5.02576378834927,-4.97338409018216,-4.88079830608383,-4.86525974655114,
-4.85258707442919,-4.83574942302132,-4.78080134286866,-4.66426854438349,
-4.63592963200015,-4.61223831586623,-4.58178290849773,-4.54692666753449,
-4.47066198081675,-4.41655177900153,-4.39977664938611,-4.38711922061191,
-4.36884058323063,-4.34622863933131,-4.29362138147143,-4.20868051162857,
-4.17772831554607,-4.153968166327,-4.12634409390635,-4.06414485520939,-3.99316939908279,
-3.9512880072954,-3.9350046218929,-3.9222721619858,-3.90288743283804,-3.82514334413091,
-3.79455919053801,-3.73524112807164,-3.70744511817718,-3.68393208073028,
-3.65284815981533,-3.57575833230207,-3.49175970537597,-3.47541175515693,
-3.46264712666091,-3.44656482193475,-3.40233582021728,-3.34944051758646,
-3.27544666702614,-3.24637554499574,-3.22271196292625,-3.1931250345579,
-3.0666442707149,-3.02358198437376,-3.00743616719612,-2.99468229505708,
-2.97507273668637,-2.9619614306192,-2.92136634805748,-2.81027466971957,
-2.7817001388985,-2.75824833629441,-2.7282273842617,-2.64473239184088,-2.56664748201972,
-2.54747680819553,-2.53476292974152,-2.51834114956905,-2.46997835697277,
-2.37177799286476,-2.33203424036561,-2.30968496589827,-2.28519289835624,
-2.24767871416892,-2.22240866395265,-2.13076386697722,-2.09522623310789,
-2.07946916398594,-2.06663819593896,-2.0463229812227,-2.0200569220251,-1.94774618660062,
-1.93112068746492,-1.91819499630147),.UNSPECIFIED.);
#842=B_SPLINE_CURVE_WITH_KNOTS('',3,(#82000,#82001,#82002,#82003,#82004,
#82005,#82006,#82007,#82008,#82009,#82010,#82011,#82012,#82013,#82014,#82015,
#82016,#82017,#82018,#82019,#82020,#82021,#82022,#82023,#82024,#82025,#82026,
#82027,#82028,#82029,#82030,#82031,#82032,#82033,#82034,#82035,#82036,#82037,
#82038,#82039,#82040,#82041,#82042,#82043,#82044,#82045,#82046,#82047,#82048,
#82049,#82050,#82051,#82052,#82053,#82054,#82055,#82056,#82057,#82058,#82059,
#82060,#82061,#82062,#82063,#82064,#82065,#82066,#82067,#82068,#82069,#82070,
#82071,#82072,#82073,#82074,#82075,#82076,#82077,#82078,#82079,#82080,#82081,
#82082,#82083,#82084,#82085,#82086,#82087,#82088,#82089,#82090,#82091,#82092,
#82093,#82094,#82095,#82096,#82097,#82098,#82099,#82100,#82101,#82102,#82103,
#82104,#82105,#82106,#82107,#82108,#82109,#82110,#82111,#82112,#82113,#82114,
#82115,#82116,#82117,#82118,#82119,#82120,#82121,#82122,#82123,#82124,#82125,
#82126,#82127,#82128,#82129,#82130,#82131,#82132,#82133,#82134,#82135,#82136,
#82137,#82138,#82139,#82140,#82141,#82142,#82143,#82144,#82145,#82146,#82147,
#82148,#82149,#82150,#82151,#82152,#82153,#82154,#82155,#82156,#82157,#82158,
#82159,#82160,#82161,#82162,#82163,#82164,#82165,#82166,#82167,#82168,#82169,
#82170,#82171,#82172,#82173,#82174,#82175,#82176,#82177,#82178,#82179,#82180,
#82181,#82182,#82183,#82184,#82185,#82186,#82187,#82188,#82189,#82190,#82191,
#82192,#82193,#82194,#82195,#82196,#82197,#82198,#82199,#82200,#82201,#82202,
#82203,#82204,#82205,#82206,#82207,#82208,#82209,#82210,#82211,#82212,#82213,
#82214,#82215,#82216,#82217,#82218,#82219,#82220,#82221,#82222,#82223,#82224,
#82225,#82226,#82227,#82228,#82229,#82230,#82231,#82232,#82233,#82234,#82235,
#82236,#82237,#82238,#82239,#82240,#82241,#82242,#82243,#82244,#82245,#82246,
#82247,#82248,#82249,#82250,#82251,#82252,#82253,#82254,#82255,#82256,#82257,
#82258,#82259,#82260,#82261),.UNSPECIFIED.,.F.,.F.,(4,2,2,2,2,2,2,2,2,2,
2,2,2,2,2,2,2,2,2,2,2,2,2,2,2,2,2,2,2,2,2,2,2,2,2,2,2,2,2,2,2,2,2,2,2,2,
2,2,2,2,2,2,2,2,2,2,2,2,2,2,2,2,2,2,2,2,2,2,2,2,2,2,2,2,2,2,2,2,2,2,2,2,
2,2,2,2,2,2,2,2,2,2,2,2,2,2,2,2,2,2,2,2,2,2,2,2,2,2,2,2,2,2,2,2,2,2,2,2,
2,2,2,2,2,2,2,2,2,2,2,2,4),(-3.97106902784548,-3.92763702759207,-3.88658726948169,
-3.86157564296453,-3.83677143377912,-3.79712325142066,-3.74468343813467,
-3.71930870986453,-3.67855003444377,-3.64596163986994,-3.63121485673307,
-3.61802438814193,-3.59516984522404,-3.57878598034135,-3.52057697670576,
-3.47447712698077,-3.42716169972195,-3.40124808422559,-3.3770314632448,
-3.34148628585702,-3.29655584204512,-3.22516500407385,-3.18603234543882,
-3.16989907684228,-3.15714308560228,-3.13751237530974,-3.07548303671522,
-2.97699289886706,-2.94692082160117,-2.92324532436927,-2.89460137822684,
-2.81677771574109,-2.72646537129329,-2.71028098076275,-2.69753885782243,
-2.68131928490212,-2.63551235245105,-2.51274633614994,-2.48287398686597,
-2.45920466084796,-2.43039101748281,-2.34751381213038,-2.26309873669759,
-2.2467721866917,-2.23401058227639,-2.21791067086075,-2.17348570310189,
-2.1200220147858,-2.04674442946513,-2.0177048269426,-1.99404069618889,-1.96441975132728,
-1.93097753686296,-1.86185582314895,-1.85352372285057,-1.79693737035706,
-1.78016703054182,-1.76750929180927,-1.74922452449514,-1.68025602220506,
-1.58712567071024,-1.55692645471647,-1.53322060704891,-1.50508041606367,
-1.4364223163488,-1.36405595990008,-1.32992978739223,-1.31433086946165,
-1.3014604671143,-1.28082355616448,-1.2539582281551,-1.17770366320611,-1.11698099230666,
-1.08875463234774,-1.06505534980239,-1.03444869698213,-1.01595871852822,
-0.964547150835598,-0.871350335210757,-0.855331785850333,-0.842610685524731,
-0.841971808595246,-0.841598533267113,-0.841016873017116,-0.840476030622721,
-0.839967576677204,-0.839484904299374,-0.839022702077622,-0.838576597640662,
-0.838142908864513,-0.837718465167538,-0.837300475579303,-0.836886428710489,
-0.83647401478626,-0.83606106307723,-0.835645490086229,-0.835225255142268,
-0.8347983209602,-0.834362617250619,-0.833916005886004,-0.83345624637869,
-0.83298096054626,-0.832487595370593,-0.831973383073842,-0.831435297421812,
-0.830870005246937,-0.830273812123175,-0.829642601008122,-0.828971762612169,
-0.811325756352297,-0.778014452110565,-0.656225603591129,-0.627005057000953,
-0.60526296837011,-0.578223232538482,-0.513942971878402,-0.408329105522501,
-0.392024514695536,-0.37945768711879,-0.372205583438089,-0.368508017567174,
-0.364538771885888,-0.35870535677802,-0.336516659750203,-0.28582242840502,
-0.19456591449315,-0.164613128014372,-0.140941586881161,-0.118416890036587,
-0.0893764328265369,-0.000139981276188635),.UNSPECIFIED.);
#843=B_SPLINE_CURVE_WITH_KNOTS('',3,(#82262,#82263,#82264,#82265,#82266,
#82267,#82268,#82269),.UNSPECIFIED.,.F.,.F.,(4,1,1,1,1,4),(51.3606186663471,
51.8372191261183,52.3319371144343,52.8266551027503,53.3213730910663,53.4070751110264),
 .UNSPECIFIED.);
#844=B_SPLINE_CURVE_WITH_KNOTS('',3,(#82271,#82272,#82273,#82274,#82275,
#82276,#82277,#82278,#82279,#82280,#82281,#82282,#82283,#82284,#82285,#82286,
#82287,#82288,#82289,#82290,#82291,#82292,#82293,#82294,#82295,#82296,#82297,
#82298,#82299,#82300,#82301,#82302,#82303,#82304,#82305,#82306,#82307,#82308,
#82309,#82310,#82311,#82312,#82313,#82314,#82315,#82316,#82317,#82318,#82319,
#82320,#82321,#82322,#82323,#82324,#82325,#82326,#82327,#82328,#82329,#82330,
#82331,#82332,#82333,#82334,#82335,#82336,#82337,#82338,#82339,#82340,#82341,
#82342,#82343,#82344,#82345,#82346,#82347,#82348,#82349,#82350,#82351,#82352,
#82353,#82354,#82355,#82356,#82357,#82358,#82359,#82360,#82361,#82362,#82363,
#82364,#82365,#82366,#82367,#82368,#82369,#82370,#82371,#82372,#82373,#82374,
#82375,#82376),.UNSPECIFIED.,.F.,.F.,(4,2,2,2,2,2,2,2,2,2,2,2,2,2,2,2,2,
2,2,2,2,2,2,2,2,2,2,2,2,2,2,2,2,2,2,2,2,2,2,2,2,2,2,2,2,2,2,2,2,2,2,2,4),
(-1.91819499630147,-1.87766457283462,-1.85070973980333,-1.82683283538219,
-1.79407155318896,-1.71482950507396,-1.63860667925558,-1.61977518415059,
-1.6070870775522,-1.59043063343498,-1.53863980797281,-1.41784389016388,
-1.38972214811814,-1.36601476848303,-1.33526346641363,-1.31664055887158,
-1.26464110781738,-1.23166413753118,-1.22234416155914,-1.17083002724642,
-1.15404420940821,-1.1413872571699,-1.12312171934314,-1.10053258824019,
-1.0480302443296,-0.96291390268036,-0.931969030139395,-0.908209396563523,
-0.880580497888131,-0.818328981072665,-0.747343504341567,-0.740218637105036,
-0.70416063323493,-0.688422966350614,-0.675998044370477,-0.662701351071325,
-0.642577968887252,-0.600420092881105,-0.493624541301765,-0.464976406255507,
-0.443133510839089,-0.420702987473508,-0.368555841706777,-0.279372293480822,
-0.24073541960509,-0.224897825626572,-0.212422821125956,-0.199161181862277,
-0.179138713400343,-0.100949134524616,-0.0341860253130483,-0.0155898498183682,
-0.000147296708047949),.UNSPECIFIED.);
#845=B_SPLINE_CURVE_WITH_KNOTS('',3,(#82377,#82378,#82379,#82380,#82381,
#82382,#82383,#82384,#82385,#82386,#82387,#82388,#82389),.UNSPECIFIED.,
 .F.,.F.,(4,1,1,1,1,1,1,1,1,1,4),(53.4070751110264,53.6660618546801,54.1607798429962,
54.6554978313122,55.1502158196282,55.6449338079442,56.1396517962603,56.6343697845763,
57.1290877728923,57.6238057612083,57.6438045939519),.UNSPECIFIED.);
#846=B_SPLINE_CURVE_WITH_KNOTS('',3,(#82394,#82395,#82396,#82397,#82398,
#82399,#82400,#82401,#82402,#82403,#82404,#82405,#82406,#82407,#82408,#82409,
#82410,#82411,#82412,#82413,#82414,#82415,#82416,#82417,#82418,#82419,#82420,
#82421,#82422,#82423,#82424,#82425,#82426,#82427,#82428,#82429,#82430,#82431,
#82432,#82433,#82434,#82435,#82436,#82437,#82438,#82439,#82440,#82441,#82442,
#82443,#82444,#82445,#82446,#82447,#82448,#82449,#82450,#82451,#82452,#82453,
#82454,#82455,#82456,#82457,#82458,#82459,#82460,#82461,#82462,#82463,#82464,
#82465,#82466,#82467,#82468,#82469,#82470,#82471,#82472,#82473,#82474,#82475,
#82476,#82477,#82478,#82479,#82480,#82481,#82482,#82483,#82484,#82485,#82486,
#82487,#82488,#82489,#82490,#82491,#82492,#82493,#82494,#82495,#82496,#82497,
#82498,#82499,#82500,#82501,#82502,#82503,#82504,#82505,#82506,#82507,#82508,
#82509,#82510,#82511,#82512,#82513,#82514,#82515,#82516,#82517,#82518,#82519,
#82520,#82521,#82522,#82523,#82524,#82525,#82526,#82527,#82528,#82529,#82530,
#82531,#82532,#82533,#82534,#82535,#82536,#82537,#82538,#82539,#82540,#82541,
#82542,#82543,#82544,#82545,#82546,#82547,#82548,#82549,#82550,#82551,#82552,
#82553,#82554,#82555,#82556,#82557,#82558,#82559,#82560,#82561,#82562,#82563,
#82564,#82565,#82566,#82567,#82568,#82569,#82570,#82571,#82572,#82573,#82574,
#82575,#82576,#82577,#82578,#82579,#82580,#82581,#82582,#82583,#82584,#82585,
#82586,#82587,#82588,#82589,#82590,#82591,#82592,#82593,#82594,#82595,#82596,
#82597,#82598,#82599,#82600,#82601,#82602,#82603,#82604,#82605,#82606,#82607,
#82608,#82609,#82610,#82611,#82612,#82613,#82614,#82615,#82616,#82617,#82618,
#82619,#82620,#82621,#82622,#82623,#82624,#82625,#82626,#82627,#82628,#82629,
#82630,#82631,#82632,#82633,#82634,#82635,#82636,#82637,#82638,#82639,#82640,
#82641,#82642,#82643,#82644,#82645,#82646,#82647,#82648,#82649,#82650,#82651,
#82652,#82653,#82654,#82655,#82656,#82657,#82658,#82659,#82660,#82661,#82662,
#82663,#82664,#82665,#82666,#82667,#82668,#82669,#82670,#82671,#82672,#82673,
#82674,#82675,#82676,#82677,#82678,#82679,#82680,#82681,#82682,#82683,#82684,
#82685),.UNSPECIFIED.,.F.,.F.,(4,2,2,2,2,2,2,2,2,2,2,2,2,2,2,2,2,2,2,2,
2,2,2,2,2,2,2,2,2,2,2,2,2,2,2,2,2,2,2,2,2,2,2,2,2,2,2,2,2,2,2,2,2,2,2,2,
2,2,2,2,2,2,2,2,2,2,2,2,2,2,2,2,2,2,2,2,2,2,2,2,2,2,2,2,2,2,2,2,2,2,2,2,
2,2,2,2,2,2,2,2,2,2,2,2,2,2,2,2,2,2,2,2,2,2,2,2,2,2,2,2,2,2,2,2,2,2,2,2,
2,2,2,2,2,2,2,2,2,2,2,2,2,2,2,2,2,4),(-9.86015336115856,-9.85112107665557,
-9.73234097774461,-9.67907491002362,-9.66232973585665,-9.64964966553001,
-9.63093939286098,-9.55346161428105,-9.46848977915582,-9.43844076773081,
-9.41498789206796,-9.38643655715724,-9.2747466562768,-9.21601068168618,
-9.19899630765461,-9.18633504712259,-9.16796991697759,-9.11662958873329,
-9.04061738726003,-9.00580818792979,-8.97538018470112,-8.95168998360197,
-8.92332970768221,-8.80723506060394,-8.75194962552062,-8.73509428103419,
-8.7224227714209,-8.70385735242706,-8.62502559433194,-8.54105198095022,
-8.51102185785259,-8.48756957904827,-8.45900234775354,-8.3477111488377,
-8.3072202899935,-8.28012563495795,-8.26622884022644,-8.25243701797931,
-8.22596286234655,-8.12286278334457,-8.09637382329746,-8.05772678593365,
-8.03306987492616,-8.01088026991953,-7.97233364650726,-7.87377414164528,
-7.82380622701391,-7.80726935678347,-7.79456889389346,-7.77556793543447,
-7.72280811588031,-7.6863040883554,-7.63424773593838,-7.59477525556185,
-7.56999679569308,-7.54790772441784,-7.51012282186554,-7.40273633132772,
-7.35891725706706,-7.34287192003409,-7.33010040689837,-7.31370626843554,
-7.2282247323264,-7.22215939427984,-7.170348323014,-7.13098885485114,-7.10622698907692,
-7.0811671137208,-7.03979329316824,-7.00574600627153,-6.93141886167929,
-6.90484124158917,-6.88435831391051,-6.87150695686912,-6.85583337717617,
-6.82117650596712,-6.72870682155704,-6.70334030097632,-6.66573504471784,
-6.64122963123573,-6.61889390092359,-6.57925290940474,-6.48101497679801,
-6.43251820348115,-6.41608627558843,-6.40337347458836,-6.38421758849865,
-6.31915745810591,-6.25316707945606,-6.23169953994733,-6.19793527587825,
-6.17394561104494,-6.147424039819,-6.0954754239936,-6.0546002044583,-5.99766332840923,
-5.97414202140216,-5.9553443672419,-5.9438378775019,-5.92796091797475,-5.88921018058492,
-5.80738331403327,-5.751789343871,-5.72419275012434,-5.702808400446,-5.67277371661147,
-5.58763036529654,-5.5103155132909,-5.49158776523044,-5.47890645502993,
-5.46217389855026,-5.409127062288,-5.29005024509407,-5.26183725705596,-5.23813683574541,
-5.20751153712327,-5.18900449860782,-5.13751794380597,-5.04462723108378,
-5.02853972464975,-5.01581007563393,-4.99950581333244,-4.95266601441447,
-4.85493067453439,-4.81393048047088,-4.78892608679856,-4.76411500771177,
-4.72442103281901,-4.67188119314957,-4.57984323469745,-4.56420311164501,
-4.55152179124098,-4.53479024155588,-4.48175935887976,-4.36266193486768,
-4.33445019780762,-4.31074982326731,-4.28012318965012,-4.26161487334029,
-4.21012252237014,-4.1172562378652,-4.10116362116595,-4.0884333873929,-4.0721338186792,
-4.02535174248445,-3.97106902784548),.UNSPECIFIED.);
#847=B_SPLINE_CURVE_WITH_KNOTS('',3,(#82687,#82688,#82689,#82690,#82691,
#82692,#82693,#82694),.UNSPECIFIED.,.F.,.F.,(4,1,1,1,1,4),(57.6438045939519,
58.1185237495243,58.6132417378404,59.1079597261564,59.6026777144724,59.690260418206),
 .UNSPECIFIED.);
#848=B_SPLINE_CURVE_WITH_KNOTS('',3,(#82695,#82696,#82697,#82698,#82699,
#82700,#82701,#82702,#82703,#82704,#82705,#82706,#82707,#82708,#82709,#82710,
#82711,#82712,#82713,#82714,#82715,#82716,#82717,#82718,#82719,#82720,#82721,
#82722,#82723,#82724,#82725,#82726,#82727,#82728,#82729,#82730,#82731,#82732,
#82733,#82734,#82735,#82736,#82737,#82738,#82739,#82740,#82741,#82742,#82743,
#82744,#82745,#82746,#82747,#82748,#82749,#82750,#82751,#82752,#82753,#82754,
#82755,#82756,#82757,#82758,#82759,#82760,#82761,#82762,#82763,#82764,#82765,
#82766,#82767,#82768,#82769,#82770,#82771,#82772,#82773,#82774,#82775,#82776,
#82777,#82778,#82779,#82780,#82781,#82782,#82783,#82784,#82785,#82786,#82787,
#82788,#82789,#82790,#82791,#82792,#82793,#82794,#82795,#82796,#82797,#82798,
#82799,#82800,#82801,#82802,#82803,#82804,#82805,#82806,#82807,#82808,#82809,
#82810,#82811,#82812,#82813,#82814,#82815,#82816,#82817,#82818,#82819,#82820,
#82821,#82822,#82823,#82824,#82825,#82826,#82827,#82828,#82829,#82830,#82831,
#82832,#82833,#82834,#82835,#82836,#82837,#82838,#82839,#82840,#82841,#82842,
#82843,#82844,#82845,#82846,#82847,#82848,#82849,#82850,#82851,#82852,#82853,
#82854,#82855,#82856,#82857,#82858,#82859,#82860,#82861,#82862,#82863,#82864,
#82865,#82866,#82867,#82868,#82869,#82870,#82871,#82872,#82873,#82874,#82875,
#82876,#82877,#82878,#82879,#82880,#82881,#82882,#82883,#82884,#82885,#82886,
#82887,#82888,#82889,#82890,#82891,#82892,#82893,#82894,#82895,#82896,#82897,
#82898,#82899,#82900,#82901,#82902,#82903,#82904,#82905,#82906,#82907,#82908,
#82909,#82910,#82911,#82912,#82913,#82914,#82915,#82916,#82917,#82918,#82919,
#82920,#82921,#82922,#82923,#82924,#82925,#82926,#82927,#82928,#82929,#82930,
#82931,#82932,#82933,#82934,#82935,#82936,#82937,#82938),.UNSPECIFIED.,
 .F.,.F.,(4,2,2,2,2,2,2,2,2,2,2,2,2,2,2,2,2,2,2,2,2,2,2,2,2,2,2,2,2,2,2,
2,2,2,2,2,2,2,2,2,2,2,2,2,2,2,2,2,2,2,2,2,2,2,2,2,2,2,2,2,2,2,2,2,2,2,2,
2,2,2,2,2,2,2,2,2,2,2,2,2,2,2,2,2,2,2,2,2,2,2,2,2,2,2,2,2,2,2,2,2,2,2,2,
2,2,2,2,2,2,2,2,2,2,2,2,2,2,2,2,2,2,4),(-11.7782433813122,-11.671195119626,
-11.6473056010272,-11.6246665597352,-11.598752315003,-11.5514323970964,
-11.5051023112653,-11.4470576971769,-11.4233144249748,-11.4167649936174,
-11.412514330664,-11.408934675872,-11.4013304508867,-11.3888355709107,-11.3698816668961,
-11.2712794337868,-11.2029058896194,-11.1753604768282,-11.1537618919276,
-11.1248693547153,-11.0009641587299,-10.9682950672716,-10.9508432664319,
-10.9501945134906,-10.9495829148123,-10.9490041309768,-10.9484542778668,
-10.9479298614948,-10.9474277204746,-10.946944974927,-10.9464789807197,
-10.9460272879692,-10.9455876028475,-10.9451577517098,-10.9447356465859,
-10.9443192509673,-10.9439065447685,-10.9434954871308,-10.9430839754008,
-10.9426697982165,-10.942250579915,-10.9293947922388,-10.9137394347937,
-10.876819551278,-10.8455121371138,-10.7764745552988,-10.7430501617321,
-10.7134397120378,-10.6897756517681,-10.6607260850306,-10.550848274455,
-10.5103612654862,-10.4972729434807,-10.4776873479655,-10.4649358198072,
-10.4487756267148,-10.4096435430698,-10.3214283543408,-10.2965750221025,
-10.2594557512361,-10.2350202376197,-10.2126083449402,-10.1723981475647,
-10.0688810548932,-10.0256192830561,-10.0096257475398,-9.99684474971968,
-9.98038599542834,-9.8835911299728,-9.82680570880455,-9.79262003133798,
-9.76857950739939,-9.7422188362255,-9.69154298124339,-9.60225585210072,
-9.56134555490115,-9.54558388244023,-9.53275390079849,-9.5124474570374,
-9.45661100564261,-9.38619139679131,-9.36394538057102,-9.329386850422,-9.30529951752727,
-9.27907138823502,-9.22941808939449,-9.18566307231222,-9.12834348619326,
-9.10474506181329,-9.08590380981178,-9.07439252219019,-9.05854250537307,
-9.01986837505997,-8.94831148201065,-8.88320511691128,-8.85533163827514,
-8.83160077915512,-8.80102750444044,-8.69458410696588,-8.63695913221868,
-8.61999204731709,-8.60732795400351,-8.5889041838377,-8.49284378594965,
-8.44374158551736,-8.40566064934577,-8.38108641082387,-8.35579106529998,
-8.31281680921966,-8.21339842953975,-8.17076238758113,-8.15482828655533,
-8.1420355796061,-8.12550048789552,-8.04370013019104,-7.96980156264351,
-7.936648225396,-7.91272887766949,-7.88595269996078,-7.83189839505448,-7.81526137055862,
-7.8073037175468),.UNSPECIFIED.);
#849=B_SPLINE_CURVE_WITH_KNOTS('',3,(#82944,#82945,#82946,#82947,#82948,
#82949,#82950,#82951,#82952,#82953,#82954,#82955,#82956,#82957,#82958,#82959,
#82960,#82961,#82962,#82963,#82964,#82965,#82966,#82967,#82968,#82969,#82970,
#82971,#82972,#82973,#82974,#82975,#82976,#82977,#82978,#82979,#82980,#82981,
#82982,#82983,#82984,#82985,#82986,#82987,#82988,#82989,#82990,#82991,#82992,
#82993,#82994,#82995,#82996,#82997,#82998,#82999,#83000,#83001,#83002,#83003,
#83004,#83005,#83006,#83007,#83008,#83009,#83010,#83011,#83012,#83013,#83014,
#83015,#83016,#83017,#83018,#83019,#83020,#83021,#83022,#83023,#83024,#83025,
#83026,#83027,#83028,#83029,#83030,#83031,#83032,#83033,#83034,#83035,#83036,
#83037,#83038,#83039,#83040,#83041,#83042,#83043,#83044,#83045,#83046,#83047,
#83048,#83049,#83050,#83051,#83052,#83053,#83054,#83055,#83056,#83057,#83058,
#83059,#83060,#83061,#83062,#83063,#83064,#83065,#83066,#83067,#83068,#83069,
#83070,#83071,#83072,#83073,#83074,#83075,#83076,#83077,#83078,#83079,#83080,
#83081,#83082,#83083,#83084,#83085,#83086,#83087,#83088,#83089,#83090,#83091,
#83092,#83093,#83094,#83095,#83096,#83097,#83098,#83099,#83100,#83101,#83102,
#83103,#83104,#83105,#83106,#83107,#83108,#83109,#83110,#83111,#83112,#83113,
#83114,#83115,#83116,#83117,#83118,#83119,#83120,#83121,#83122,#83123,#83124,
#83125,#83126,#83127,#83128,#83129,#83130,#83131,#83132,#83133,#83134,#83135,
#83136,#83137,#83138,#83139,#83140,#83141,#83142,#83143,#83144,#83145,#83146,
#83147,#83148,#83149),.UNSPECIFIED.,.F.,.F.,(4,2,2,2,2,2,2,2,2,2,2,2,2,
2,2,2,2,2,2,2,2,2,2,2,2,2,2,2,2,2,2,2,2,2,2,2,2,2,2,2,2,2,2,2,2,2,2,2,2,
2,2,2,2,2,2,2,2,2,2,2,2,2,2,2,2,2,2,2,2,2,2,2,2,2,2,2,2,2,2,2,2,2,2,2,2,
2,2,2,2,2,2,2,2,2,2,2,2,2,2,2,2,2,4),(-3.97106360210015,-3.93154941246759,
-3.91534326741906,-3.90259826317977,-3.88639738128753,-3.84081185867932,
-3.71951182690687,-3.68931028839893,-3.66560431106409,-3.63746587323261,
-3.56883288056332,-3.49647260530372,-3.46232003672252,-3.44671727956274,
-3.4338479046664,-3.41321909845903,-3.38636894111882,-3.31021733843855,
-3.24969937392289,-3.22136309713559,-3.19767141447138,-3.16721203280993,
-3.13234915561305,-3.05604983167387,-3.00194770542473,-2.98518978414246,
-2.97253136466594,-2.95423098475025,-2.93158130477272,-2.87880094740292,
-2.7941439040794,-2.76318007271603,-2.73941878842122,-2.71180168845739,
-2.6496813948042,-2.57872010813792,-2.53681247685938,-2.52049133638009,
-2.50776412338351,-2.48843866028749,-2.47559908004031,-2.39722618196737,
-2.3243639623351,-2.29535416049886,-2.27168940342283,-2.24203587860026,
-2.22441494897889,-2.19927707050256,-2.1087441126888,-2.07134810063568,
-2.05573238847377,-2.04286631347507,-2.02226430252417,-1.99546437139115,
-1.9196533220304,-1.85833069935911,-1.83011171892852,-1.80641172640206,
-1.77579456936414,-1.7572950110357,-1.70584144049654,-1.6128177573806,-1.59675964194115,
-1.58403364622509,-1.56770317870616,-1.52053350097482,-1.42268634605136,
-1.38196842104908,-1.35700580281315,-1.33215568560653,-1.29219779257155,
-1.23907726405921,-1.14832949305187,-1.13259936320152,-1.11990966706137,
-1.10326930029612,-1.05173452906981,-0.936637390580611,-0.906425310718271,
-0.882744613850218,-0.854215098157555,-0.778946988843379,-0.684767816069046,
-0.668980502577175,-0.656285143818308,-0.644039947635034,-0.627019610541083,
-0.59575401550241,-0.479312122330603,-0.447076554926775,-0.423615884180066,
-0.399483243967795,-0.372125365902695,-0.34827155072839,-0.267531186387864,
-0.218913608109173,-0.202548666952636,-0.191138962330041,-0.178542598726127,
-0.160457842190778,-0.125671030034368,-0.025411561791965,-0.000144225401985139),
 .UNSPECIFIED.);
#850=B_SPLINE_CURVE_WITH_KNOTS('',3,(#83150,#83151,#83152,#83153,#83154,
#83155,#83156,#83157,#83158,#83159,#83160,#83161,#83162,#83163,#83164,#83165,
#83166,#83167,#83168,#83169,#83170,#83171,#83172,#83173,#83174,#83175,#83176,
#83177,#83178,#83179,#83180,#83181,#83182,#83183,#83184,#83185,#83186,#83187,
#83188,#83189,#83190,#83191,#83192,#83193,#83194,#83195,#83196,#83197,#83198,
#83199,#83200,#83201,#83202,#83203,#83204,#83205,#83206,#83207,#83208,#83209,
#83210,#83211,#83212,#83213,#83214,#83215,#83216,#83217,#83218,#83219,#83220,
#83221,#83222,#83223,#83224,#83225,#83226,#83227,#83228,#83229,#83230,#83231,
#83232,#83233,#83234,#83235,#83236,#83237,#83238,#83239,#83240,#83241,#83242,
#83243,#83244,#83245,#83246,#83247,#83248,#83249,#83250,#83251,#83252,#83253,
#83254,#83255,#83256,#83257,#83258,#83259,#83260,#83261,#83262,#83263,#83264,
#83265,#83266,#83267,#83268,#83269,#83270,#83271,#83272,#83273,#83274,#83275,
#83276,#83277,#83278,#83279,#83280,#83281,#83282,#83283),.UNSPECIFIED.,
 .F.,.F.,(4,2,2,2,2,2,2,2,2,2,2,2,2,2,2,2,2,2,2,2,2,2,2,2,2,2,2,2,2,2,2,
2,2,2,2,2,2,2,2,2,2,2,2,2,2,2,2,2,2,2,2,2,2,2,2,2,2,2,2,2,2,2,2,2,2,2,4),
(-11.7782575909705,-11.7575540749702,-11.7369611070762,-11.7099771235911,
-11.6568567564943,-11.5552551067953,-11.5282812880275,-11.516182296382,
-11.5034219449728,-11.4871032548703,-11.4023154228092,-11.3197716048351,
-11.2964182480323,-11.2787602779056,-11.2535336455908,-11.212763532941,
-11.1112177793469,-11.0812833824136,-11.0776916759057,-11.0756434608909,
-11.073407044803,-11.071605746434,-11.0701524098604,-11.0689762136385,-11.0680206179461,
-11.0672409400877,-11.0666020329901,-11.0660762717131,-11.0656419014181,
-11.0652817257151,-11.0649820852044,-11.0647320703852,-11.0645229180375,
-11.0637768884411,-11.0630779539183,-11.0624209159605,-11.0618010465555,
-11.0533233711773,-11.0406372792275,-11.0249428765762,-10.9303725641988,
-10.8792717018237,-10.8608525571439,-10.8303232403025,-10.8066283466347,
-10.7783454237913,-10.6606599979269,-10.6065800181202,-10.5897890331692,
-10.5771128407755,-10.5584639193114,-10.4804095028337,-10.3930812579989,
-10.3640423659618,-10.3403784154605,-10.3107571883045,-10.1896140519374,
-10.1418789080586,-10.1255045955927,-10.1127846910637,-10.0967756194634,
-10.0035404674789,-9.95213954384135,-9.93365204672542,-9.90304812855436,
-9.87934913223944,-9.86015336115856),.UNSPECIFIED.);
#851=B_SPLINE_CURVE_WITH_KNOTS('',3,(#83284,#83285,#83286,#83287,#83288,
#83289,#83290,#83291,#83292,#83293,#83294,#83295,#83296,#83297,#83298,#83299,
#83300,#83301,#83302,#83303,#83304,#83305,#83306,#83307,#83308,#83309,#83310,
#83311,#83312,#83313,#83314,#83315,#83316,#83317,#83318,#83319,#83320,#83321,
#83322,#83323,#83324,#83325,#83326,#83327,#83328,#83329,#83330,#83331,#83332,
#83333,#83334,#83335,#83336,#83337,#83338,#83339,#83340,#83341,#83342,#83343,
#83344,#83345,#83346,#83347,#83348,#83349,#83350,#83351,#83352,#83353,#83354,
#83355,#83356,#83357,#83358,#83359,#83360,#83361,#83362,#83363,#83364,#83365,
#83366,#83367,#83368,#83369,#83370,#83371,#83372,#83373,#83374,#83375,#83376,
#83377,#83378,#83379,#83380,#83381,#83382,#83383,#83384,#83385,#83386,#83387,
#83388,#83389,#83390,#83391,#83392,#83393,#83394,#83395,#83396,#83397,#83398,
#83399,#83400,#83401,#83402,#83403,#83404,#83405,#83406,#83407,#83408,#83409,
#83410,#83411,#83412,#83413,#83414,#83415,#83416,#83417,#83418,#83419,#83420,
#83421,#83422,#83423,#83424,#83425,#83426,#83427,#83428,#83429,#83430,#83431,
#83432,#83433,#83434,#83435,#83436,#83437,#83438,#83439,#83440,#83441,#83442,
#83443,#83444,#83445,#83446,#83447,#83448,#83449,#83450,#83451,#83452,#83453,
#83454,#83455,#83456,#83457,#83458,#83459,#83460,#83461,#83462,#83463,#83464,
#83465,#83466,#83467,#83468,#83469,#83470,#83471,#83472,#83473,#83474,#83475,
#83476,#83477,#83478,#83479,#83480,#83481,#83482,#83483,#83484,#83485,#83486,
#83487,#83488,#83489,#83490,#83491,#83492,#83493,#83494,#83495,#83496,#83497,
#83498,#83499,#83500,#83501,#83502,#83503,#83504,#83505,#83506,#83507,#83508,
#83509,#83510,#83511,#83512,#83513,#83514,#83515,#83516,#83517,#83518,#83519,
#83520,#83521,#83522,#83523,#83524,#83525,#83526,#83527,#83528,#83529,#83530,
#83531,#83532,#83533,#83534,#83535,#83536,#83537,#83538,#83539,#83540,#83541,
#83542,#83543,#83544,#83545,#83546,#83547,#83548,#83549,#83550,#83551,#83552,
#83553,#83554,#83555,#83556,#83557,#83558,#83559,#83560,#83561,#83562,#83563,
#83564,#83565,#83566,#83567,#83568,#83569,#83570,#83571,#83572,#83573,#83574,
#83575),.UNSPECIFIED.,.F.,.F.,(4,2,2,2,2,2,2,2,2,2,2,2,2,2,2,2,2,2,2,2,
2,2,2,2,2,2,2,2,2,2,2,2,2,2,2,2,2,2,2,2,2,2,2,2,2,2,2,2,2,2,2,2,2,2,2,2,
2,2,2,2,2,2,2,2,2,2,2,2,2,2,2,2,2,2,2,2,2,2,2,2,2,2,2,2,2,2,2,2,2,2,2,2,
2,2,2,2,2,2,2,2,2,2,2,2,2,2,2,2,2,2,2,2,2,2,2,2,2,2,2,2,2,2,2,2,2,2,2,2,
2,2,2,2,2,2,2,2,2,2,2,2,2,2,2,2,2,4),(-7.8073037175468,-7.74292118198365,
-7.72449205042442,-7.71260130911684,-7.69428604059757,-7.68162690632006,
-7.66488060267763,-7.61367995023372,-7.59095399533706,-7.52745080722082,
-7.50644536633783,-7.47315903063662,-7.44922483001077,-7.42250653484181,
-7.36894106007636,-7.34884172523891,-7.27858411274764,-7.26042892551343,
-7.24866073428695,-7.23047799738935,-7.21782404205162,-7.20097033190753,
-7.14531212426787,-7.07022069676661,-7.03558484160617,-7.00525851864319,
-6.98157288953722,-6.95313368063236,-6.82423245389675,-6.7800873275622,
-6.76401234746762,-6.75124615385068,-6.73488860646261,-6.64579612220412,
-6.59260484784879,-6.55261484140024,-6.52775983008803,-6.50280191517561,
-6.4621168874173,-6.36425471880772,-6.31704451025778,-6.30071072326953,
-6.28798505209198,-6.27193033623732,-6.17889231185864,-6.12744299971697,
-6.10894438036917,-6.07832812733441,-6.0546279934244,-6.02640789041755,
-5.9648222721677,-5.88921276289147,-5.85155812821751,-5.83593747359763,
-5.82307248216422,-5.80248010435335,-5.7756983179467,-5.70001064467656,
-5.63853809686397,-5.61031499222469,-5.58661499050462,-5.55600259843744,
-5.53750752466101,-5.48607402915805,-5.39296460190005,-5.37692548423314,
-5.36420168938903,-5.34785376741974,-5.30046325973471,-5.20254393802874,
-5.16201099553745,-5.13707554200837,-5.11219868402656,-5.0720616089203,
-5.01854408903397,-4.93091528972588,-4.91241031564853,-4.89974197024353,
-4.88283908428359,-4.82660225763457,-4.71828360346469,-4.68784014166486,
-4.66411818976943,-4.63615403090008,-4.56990446544818,-4.49809651958925,
-4.46048584326041,-4.44487184088536,-4.43200512455116,-4.411398905625,-4.38459121790057,
-4.30872876916115,-4.24745901609728,-4.21924384248143,-4.19554328001026,
-4.16492013479057,-4.14641518012815,-4.09493811802865,-4.00200708452449,
-3.9859280708723,-3.97319935991522,-3.95688717489712,-3.90994985184454,
-3.81218014182191,-3.77126329230043,-3.74627101771131,-3.72144820066655,
-3.68167629419756,-3.62896589164102,-3.53876932865768,-3.52250366458213,
-3.5097504086274,-3.49359941899154,-3.44859693966417,-3.32031140685774,
-3.29201449886223,-3.26831995178768,-3.23780768369129,-3.16531250903986,
-3.07345863005895,-3.05784470727535,-3.04516560990965,-3.02840673795051,
-2.97490384846812,-2.85796307568887,-2.82921547333254,-2.80791202717228,
-2.77925723658052,-2.70116875374401,-2.61014015700233,-2.5943707035695,
-2.58167708720648,-2.56507556253835,-2.51414391047934,-2.39214873923174,
-2.36409266784384,-2.34037950757043,-2.30953442163685,-2.23440519405854,
-2.14857693793214,-2.13014579159411,-2.1174813608415,-2.10052024235325,
-2.04302775384782,-1.9364103796757,-1.91819812389623),.UNSPECIFIED.);
#852=B_SPLINE_CURVE_WITH_KNOTS('',3,(#83580,#83581,#83582,#83583,#83584,
#83585,#83586,#83587,#83588,#83589,#83590,#83591,#83592,#83593,#83594,#83595,
#83596,#83597,#83598,#83599,#83600,#83601,#83602,#83603,#83604,#83605,#83606,
#83607,#83608,#83609,#83610,#83611,#83612,#83613,#83614,#83615,#83616,#83617,
#83618,#83619,#83620,#83621,#83622,#83623,#83624,#83625,#83626,#83627,#83628,
#83629,#83630,#83631,#83632,#83633,#83634,#83635,#83636,#83637,#83638,#83639,
#83640,#83641,#83642,#83643,#83644,#83645,#83646,#83647,#83648,#83649,#83650,
#83651,#83652,#83653,#83654,#83655,#83656,#83657,#83658,#83659,#83660,#83661,
#83662,#83663,#83664,#83665,#83666,#83667,#83668,#83669,#83670,#83671,#83672,
#83673,#83674,#83675,#83676,#83677,#83678,#83679,#83680,#83681,#83682,#83683,
#83684,#83685,#83686,#83687,#83688,#83689,#83690,#83691,#83692,#83693,#83694,
#83695,#83696,#83697,#83698,#83699,#83700,#83701,#83702,#83703,#83704,#83705,
#83706,#83707,#83708,#83709,#83710,#83711,#83712,#83713,#83714,#83715,#83716,
#83717,#83718,#83719,#83720,#83721,#83722,#83723,#83724,#83725,#83726,#83727,
#83728,#83729,#83730,#83731,#83732,#83733,#83734,#83735,#83736,#83737,#83738,
#83739,#83740,#83741,#83742,#83743,#83744,#83745,#83746,#83747,#83748,#83749,
#83750,#83751,#83752,#83753,#83754,#83755,#83756,#83757,#83758,#83759,#83760,
#83761,#83762,#83763,#83764,#83765,#83766,#83767,#83768,#83769,#83770,#83771,
#83772,#83773,#83774,#83775,#83776,#83777,#83778,#83779,#83780,#83781,#83782,
#83783,#83784,#83785,#83786,#83787,#83788,#83789,#83790,#83791,#83792,#83793,
#83794,#83795,#83796,#83797,#83798,#83799,#83800,#83801,#83802,#83803,#83804,
#83805,#83806,#83807,#83808,#83809,#83810,#83811,#83812,#83813,#83814,#83815,
#83816,#83817,#83818,#83819,#83820,#83821,#83822,#83823,#83824,#83825,#83826,
#83827,#83828,#83829,#83830,#83831,#83832,#83833,#83834,#83835,#83836,#83837,
#83838,#83839,#83840,#83841,#83842,#83843,#83844,#83845,#83846,#83847,#83848,
#83849,#83850,#83851,#83852,#83853,#83854,#83855,#83856,#83857,#83858,#83859,
#83860,#83861,#83862,#83863,#83864,#83865,#83866,#83867,#83868,#83869,#83870,
#83871),.UNSPECIFIED.,.F.,.F.,(4,2,2,2,2,2,2,2,2,2,2,2,2,2,2,2,2,2,2,2,
2,2,2,2,2,2,2,2,2,2,2,2,2,2,2,2,2,2,2,2,2,2,2,2,2,2,2,2,2,2,2,2,2,2,2,2,
2,2,2,2,2,2,2,2,2,2,2,2,2,2,2,2,2,2,2,2,2,2,2,2,2,2,2,2,2,2,2,2,2,2,2,2,
2,2,2,2,2,2,2,2,2,2,2,2,2,2,2,2,2,2,2,2,2,2,2,2,2,2,2,2,2,2,2,2,2,2,2,2,
2,2,2,2,2,2,2,2,2,2,2,2,2,2,2,2,2,4),(-9.86012475374465,-9.81805694591507,
-9.76638317281649,-9.7478337986043,-9.71716245642267,-9.69345967754844,
-9.66528061631865,-9.54555410367724,-9.49298378056098,-9.47627951278026,
-9.46359582714404,-9.44792917678455,-9.35599498939593,-9.27848877374205,
-9.2498581365546,-9.22618212653158,-9.19609412078237,-9.09756635372558,
-9.03560090988958,-9.01597708359595,-9.00333063785702,-8.98726567364478,
-8.94583519820819,-8.85912738720152,-8.83446527295588,-8.797528558207,-8.77311903712428,
-8.74757353706966,-8.70287391096224,-8.60587561757498,-8.56362781215548,
-8.54773149448201,-8.5349311880803,-8.51488175645492,-8.41798442006454,
-8.34957371320675,-8.32145076090209,-8.29774339591059,-8.26752068805409,
-8.17457810077457,-8.10400393729673,-8.08639603827367,-8.07499209212843,
-8.05854877960523,-8.00836498502534,-7.92885360126043,-7.89341029095786,
-7.86261175139507,-7.83890147756646,-7.81081295402954,-7.6894002479943,
-7.63805055333626,-7.62142192899553,-7.6087310591234,-7.58986068890172,
-7.49565365602257,-7.43545002996782,-7.40226368727481,-7.3783407408959,
-7.35157920361877,-7.29764869517202,-7.28097034323694,-7.2085273413631,
-7.18224031306595,-7.1619138010534,-7.14908145427972,-7.13333004864614,
-7.09800147018681,-7.00618995472378,-6.98090040037943,-6.94336774212854,
-6.9188729496194,-6.89652639576043,-6.85680356230483,-6.75859380374859,
-6.71020258763505,-6.69377859603814,-6.68106493058263,-6.66189746374913,
-6.59716168654103,-6.53098402851683,-6.49817641346088,-6.46893341864697,
-6.44527117415028,-6.41586328678028,-6.31097887003897,-6.26806098370764,
-6.23997186839252,-6.22591030662268,-6.21397617601239,-6.19089758677078,
-6.08328545867654,-6.04397954033149,-6.01098207459441,-5.98707990649186,
-5.96023430116837,-5.90558409960236,-5.88914154606991,-5.81713829752032,
-5.78112854424425,-5.76538747743229,-5.75255264710922,-5.73220558493534,
-5.70588056727411,-5.63319361589111,-5.61641489390075,-5.56278034871493,
-5.53605385922234,-5.51212180327659,-5.47885455286815,-5.41720906178363,
-5.32477741280231,-5.30583278021585,-5.29313653306905,-5.27656039918392,
-5.22601295040308,-5.10939772673686,-5.07932617848319,-5.05565063942082,
-5.02700611151578,-4.94916988681424,-4.85843366697098,-4.84243004761189,
-4.82971068321558,-4.81333104316248,-4.76552781880852,-4.64449837592189,
-4.61486517093543,-4.59120076920861,-4.56217230790328,-4.54511589829703,
-4.52119248885457,-4.43996218829928,-4.39195915984871,-4.37562787348718,
-4.3642154411799,-4.34646832220976,-4.3350999553969,-4.30221744949254,-4.20427050082486,
-4.16381437130908,-4.13889058125131,-4.1140030748158,-4.07379210163428,
-4.02010945622261,-3.97106360210015),.UNSPECIFIED.);
#853=B_SPLINE_CURVE_WITH_KNOTS('',3,(#83873,#83874,#83875,#83876,#83877,
#83878,#83879,#83880,#83881,#83882,#83883,#83884,#83885,#83886,#83887,#83888,
#83889,#83890,#83891,#83892,#83893,#83894,#83895,#83896,#83897,#83898,#83899,
#83900,#83901,#83902,#83903,#83904,#83905,#83906,#83907,#83908,#83909,#83910,
#83911,#83912,#83913,#83914,#83915,#83916,#83917,#83918,#83919,#83920,#83921,
#83922,#83923,#83924,#83925,#83926,#83927,#83928,#83929,#83930,#83931,#83932,
#83933,#83934,#83935,#83936,#83937,#83938,#83939,#83940,#83941,#83942,#83943,
#83944,#83945,#83946,#83947,#83948,#83949,#83950,#83951,#83952,#83953,#83954,
#83955,#83956,#83957,#83958,#83959,#83960,#83961,#83962,#83963,#83964,#83965,
#83966,#83967,#83968,#83969,#83970,#83971,#83972,#83973,#83974,#83975,#83976,
#83977,#83978,#83979,#83980,#83981,#83982,#83983,#83984,#83985,#83986,#83987,
#83988,#83989,#83990,#83991,#83992,#83993,#83994,#83995,#83996,#83997,#83998,
#83999,#84000,#84001,#84002,#84003,#84004,#84005,#84006,#84007,#84008,#84009,
#84010,#84011,#84012,#84013,#84014,#84015,#84016,#84017,#84018),
 .UNSPECIFIED.,.F.,.F.,(4,2,2,2,2,2,2,2,2,2,2,2,2,2,2,2,2,2,2,2,2,2,2,2,
2,2,2,2,2,2,2,2,2,2,2,2,2,2,2,2,2,2,2,2,2,2,2,2,2,2,2,2,2,2,2,2,2,2,2,2,
2,2,2,2,2,2,2,2,2,2,2,2,4),(-1.91819812389623,-1.9058490804987,-1.88211911746911,
-1.8542374965745,-1.78903080278789,-1.71745145019472,-1.67885684990661,
-1.66303268597609,-1.65151661409857,-1.632632900303,-1.60895940878541,-1.55126479817968,
-1.50557186200159,-1.45752823120374,-1.43151501950158,-1.40734235008991,
-1.37212664127907,-1.32871571446535,-1.22425509209492,-1.20433294426275,
-1.19154660427064,-1.17558047072642,-1.13260917932051,-1.03102427025317,
-0.989537169418201,-0.964460755422503,-0.939713715787689,-0.900453552421356,
-0.848856656785603,-0.756458768016186,-0.740252681795145,-0.727507654282451,
-0.719301269264677,-0.71873817849579,-0.718145823758188,-0.717520203283071,
-0.716856944383347,-0.716151248054843,-0.715397830381653,-0.7151825000816,
-0.714925079174424,-0.714616512330017,-0.714245513008139,-0.713797931162959,
-0.713255927242603,-0.712596898445036,-0.711792097955374,-0.710804894237682,
-0.709588649502659,-0.708084278206175,-0.706217712918539,-0.705744296785534,
-0.704892428077784,-0.703365751696435,-0.70065560504686,-0.672629558219046,
-0.587941888667891,-0.534793224722198,-0.507542293239183,-0.489843497568673,
-0.4673732733938,-0.438828689271821,-0.389528553450192,-0.294195689020745,
-0.275606447982955,-0.262933621783939,-0.250609911718129,-0.218573040534112,
-0.146182347082779,-0.0746323275261985,-0.0468036259155507,-0.0233663524740781,
-0.000143848792500651),.UNSPECIFIED.);
#854=B_SPLINE_CURVE_WITH_KNOTS('',3,(#84019,#84020,#84021,#84022,#84023,
#84024,#84025,#84026,#84027,#84028,#84029,#84030,#84031,#84032,#84033,#84034,
#84035,#84036,#84037,#84038,#84039,#84040,#84041,#84042,#84043,#84044,#84045,
#84046,#84047,#84048,#84049,#84050,#84051,#84052,#84053,#84054,#84055,#84056,
#84057,#84058,#84059,#84060,#84061,#84062,#84063,#84064,#84065,#84066,#84067,
#84068,#84069,#84070,#84071,#84072,#84073,#84074,#84075,#84076,#84077,#84078,
#84079,#84080,#84081,#84082,#84083,#84084,#84085,#84086,#84087,#84088,#84089,
#84090,#84091,#84092,#84093,#84094,#84095,#84096,#84097,#84098,#84099,#84100,
#84101,#84102,#84103,#84104,#84105,#84106,#84107,#84108,#84109,#84110,#84111,
#84112,#84113,#84114,#84115,#84116,#84117,#84118,#84119,#84120,#84121,#84122,
#84123,#84124,#84125,#84126,#84127,#84128,#84129,#84130,#84131,#84132,#84133,
#84134,#84135,#84136,#84137,#84138,#84139,#84140,#84141,#84142,#84143,#84144,
#84145,#84146,#84147,#84148,#84149,#84150,#84151,#84152,#84153,#84154,#84155,
#84156,#84157,#84158,#84159,#84160,#84161,#84162,#84163,#84164,#84165,#84166,
#84167,#84168,#84169,#84170,#84171,#84172,#84173,#84174,#84175,#84176,#84177,
#84178,#84179,#84180,#84181,#84182,#84183,#84184,#84185,#84186,#84187,#84188,
#84189,#84190,#84191,#84192,#84193,#84194,#84195,#84196,#84197,#84198,#84199,
#84200,#84201,#84202,#84203,#84204,#84205,#84206,#84207,#84208,#84209,#84210,
#84211,#84212,#84213,#84214,#84215,#84216,#84217,#84218,#84219,#84220,#84221,
#84222),.UNSPECIFIED.,.F.,.F.,(4,2,2,2,2,2,2,2,2,2,2,2,2,2,2,2,2,2,2,2,
2,2,2,2,2,2,2,2,2,2,2,2,2,2,2,2,2,2,2,2,2,2,2,2,2,2,2,2,2,2,2,2,2,2,2,2,
2,2,2,2,2,2,2,2,2,2,2,2,2,2,2,2,2,2,2,2,2,2,2,2,2,2,2,2,2,2,2,2,2,2,2,2,
2,2,2,2,2,2,2,2,2,4),(-11.7783190292283,-11.7492162270637,-11.6675692593062,
-11.6250943656212,-11.6048886037439,-11.5915631425151,-11.5791772908065,
-11.5635179196079,-11.525627476028,-11.4538809289882,-11.3879040295678,
-11.3609520810337,-11.3392014628929,-11.3107537491765,-11.2008946537563,
-11.1602437590013,-11.14051677233,-11.1273575764358,-11.1232389866094,-11.1104767599408,
-11.0941474555619,-11.0097935177337,-10.9268645008013,-10.8980490731557,
-10.8743792632854,-10.8445075675873,-10.7258181191681,-10.6765803703627,
-10.660094455377,-10.6473879660322,-10.6283118597966,-10.5738190323731,
-10.5009125332178,-10.4666990779374,-10.4366211984448,-10.4131665256044,
-10.3846372850365,-10.2723753449478,-10.2140939986964,-10.1970981782366,
-10.1844354813104,-10.1660464241347,-10.0850851367844,-10.0039359258322,
-9.97350105142926,-9.94980993292345,-9.92145352610052,-9.80525892818735,
-9.75004641150789,-9.73319446332854,-9.72052233655845,-9.70195142450754,
-9.62316445555718,-9.53811863693912,-9.50846790629941,-9.48480253204695,
-9.45578853103084,-9.38288293308005,-9.30453061291114,-9.29169887196127,
-9.27238150622478,-9.25965469807577,-9.24332753729619,-9.19800023294773,
-9.11456874202166,-9.06388283604925,-9.03752038408268,-9.01347958822037,
-8.98482051548703,-8.93972627840673,-8.93224317711163,-8.85712997391759,
-8.83043356948044,-8.80988686941316,-8.79702747752518,-8.7813845630056,
-8.74433414612589,-8.65359593667067,-8.62843334346072,-8.61080096401444,
-8.581134549036,-8.5574690611916,-8.52846982546471,-8.41722914928883,-8.3592803577413,
-8.34229878682887,-8.32963526726845,-8.31122863279196,-8.2233421871445,
-8.16985239876153,-8.1508972069372,-8.11978528243707,-8.09605412315632,
-8.06817744717281,-8.00405001307945,-7.9295594695943,-7.90295688921793,
-7.88246048809213,-7.86960732914023,-7.85393996722258,-7.81713156719808,
-7.80730129127322),.UNSPECIFIED.);
#855=B_SPLINE_CURVE_WITH_KNOTS('',3,(#84228,#84229,#84230,#84231,#84232,
#84233,#84234,#84235,#84236,#84237,#84238,#84239,#84240,#84241,#84242,#84243,
#84244,#84245,#84246,#84247,#84248,#84249,#84250,#84251,#84252,#84253,#84254,
#84255,#84256,#84257,#84258,#84259,#84260,#84261,#84262,#84263,#84264,#84265,
#84266,#84267,#84268,#84269,#84270,#84271,#84272,#84273,#84274,#84275,#84276,
#84277,#84278,#84279,#84280,#84281,#84282,#84283,#84284,#84285,#84286,#84287,
#84288,#84289,#84290,#84291,#84292,#84293,#84294,#84295,#84296,#84297,#84298,
#84299,#84300,#84301,#84302,#84303,#84304,#84305,#84306,#84307,#84308,#84309,
#84310,#84311,#84312,#84313,#84314,#84315,#84316,#84317,#84318,#84319,#84320,
#84321,#84322,#84323,#84324,#84325,#84326,#84327,#84328,#84329,#84330,#84331,
#84332,#84333,#84334,#84335,#84336,#84337,#84338,#84339,#84340,#84341,#84342,
#84343,#84344,#84345,#84346,#84347,#84348,#84349,#84350,#84351,#84352,#84353,
#84354,#84355,#84356,#84357,#84358,#84359,#84360,#84361,#84362,#84363,#84364,
#84365,#84366,#84367,#84368,#84369,#84370,#84371,#84372,#84373,#84374,#84375,
#84376,#84377,#84378,#84379,#84380,#84381,#84382,#84383,#84384,#84385,#84386,
#84387,#84388,#84389,#84390,#84391,#84392,#84393,#84394,#84395,#84396,#84397,
#84398,#84399,#84400,#84401,#84402,#84403,#84404,#84405,#84406,#84407,#84408,
#84409,#84410,#84411,#84412,#84413,#84414,#84415,#84416,#84417,#84418,#84419,
#84420,#84421,#84422,#84423,#84424,#84425,#84426,#84427,#84428,#84429,#84430,
#84431,#84432,#84433,#84434,#84435),.UNSPECIFIED.,.F.,.F.,(4,2,2,2,2,2,
2,2,2,2,2,2,2,2,2,2,2,2,2,2,2,2,2,2,2,2,2,2,2,2,2,2,2,2,2,2,2,2,2,2,2,2,
2,2,2,2,2,2,2,2,2,2,2,2,2,2,2,2,2,2,2,2,2,2,2,2,2,2,2,2,2,2,2,2,2,2,2,2,
2,2,2,2,2,2,2,2,2,2,2,2,2,2,2,2,2,2,2,2,2,2,2,2,2,4),(-3.97107570014323,
-3.95473179825932,-3.93020570680576,-3.89245600578724,-3.86693551442944,
-3.77312373637299,-3.73891431794088,-3.72373572613475,-3.71073286783546,
-3.68911897534789,-3.66039358571638,-3.5700233681002,-3.5202329848614,-3.49398699035555,
-3.46990632381394,-3.435399829625,-3.41320515749296,-3.34308808260247,-3.31458177455716,
-3.27658819463,-3.26091007323842,-3.24805997714065,-3.22758670622655,-3.20102707365061,
-3.12681642009985,-3.11318670439561,-3.05874838764347,-3.0319273757567,
-3.00801922012637,-2.97496708060967,-2.93556261129145,-2.82700389684559,
-2.80458806588298,-2.79274951820068,-2.77850296973325,-2.74926141772127,
-2.6715669437198,-2.6012429510694,-2.57252089631481,-2.55121669997346,-2.52253624128907,
-2.4437933480278,-2.35348830357128,-2.33772156953117,-2.32502823325172,
-2.30842407283542,-2.25745220623051,-2.13551300270738,-2.10745377660231,
-2.08374091170392,-2.05290041843001,-1.97974715544867,-1.89197199852887,
-1.87352118462463,-1.86085578434366,-1.8439104376255,-1.78676740370546,
-1.67968103479866,-1.64915145851153,-1.62542377696657,-1.59752035123772,
-1.53204166259927,-1.46040373978181,-1.4220408298139,-1.40628173318693,
-1.39345118573078,-1.3731398189934,-1.34688094275814,-1.27461648875262,
-1.25800982781872,-1.20449761438769,-1.17753565025881,-1.15366022090385,
-1.12091370672339,-1.10042492291373,-1.03959272848015,-0.965578501506255,
-0.94667038583358,-0.933976851013923,-0.917375117779512,-0.866439678260105,
-0.744449990918004,-0.716393696059684,-0.692680660979183,-0.665114002403756,
-0.652555049898491,-0.609840083087632,-0.538690221656287,-0.495670496848202,
-0.479810627250529,-0.471533796712322,-0.459537431588819,-0.429186928283623,
-0.40372805506196,-0.305148315625417,-0.266691316274866,-0.244513739481454,
-0.222150760767069,-0.197667044314299,-0.108830485409659,-0.0392328373056414,
-0.0201720577622807,-0.00991112195934663,-0.000147043797163775),
 .UNSPECIFIED.);
#856=B_SPLINE_CURVE_WITH_KNOTS('',3,(#84436,#84437,#84438,#84439,#84440,
#84441,#84442,#84443,#84444,#84445,#84446,#84447,#84448,#84449,#84450,#84451,
#84452,#84453,#84454,#84455,#84456,#84457,#84458,#84459,#84460,#84461,#84462,
#84463,#84464,#84465,#84466,#84467,#84468,#84469,#84470,#84471,#84472,#84473,
#84474,#84475,#84476,#84477,#84478,#84479,#84480,#84481,#84482,#84483,#84484,
#84485,#84486,#84487,#84488,#84489,#84490,#84491,#84492,#84493,#84494,#84495,
#84496,#84497,#84498,#84499,#84500,#84501,#84502,#84503,#84504,#84505,#84506,
#84507,#84508,#84509,#84510,#84511,#84512,#84513,#84514,#84515,#84516,#84517,
#84518,#84519,#84520,#84521,#84522,#84523,#84524,#84525,#84526,#84527,#84528,
#84529,#84530,#84531,#84532,#84533,#84534,#84535,#84536,#84537,#84538,#84539,
#84540,#84541,#84542,#84543,#84544,#84545),.UNSPECIFIED.,.F.,.F.,(4,2,2,
2,2,2,2,2,2,2,2,2,2,2,2,2,2,2,2,2,2,2,2,2,2,2,2,2,2,2,2,2,2,2,2,2,2,2,2,
2,2,2,2,2,2,2,2,2,2,2,2,2,2,2,4),(-11.7781571887288,-11.7684257903246,-11.7554890562485,
-11.6940865751676,-11.6184770809455,-11.5900780734401,-11.567636756316,
-11.5439447904632,-11.5139922544665,-11.4186973918007,-11.3712036358175,
-11.349754490077,-11.3335855379709,-11.3300998060477,-11.3175519573378,
-11.2987524687992,-11.2329152060424,-11.1673992444472,-11.1347387363269,
-11.1112175349723,-11.0882967914464,-11.0617153499735,-11.0092792105663,
-10.9690171151081,-10.9121529858805,-10.8886466206752,-10.869857523657,
-10.8583521437458,-10.8424703702003,-10.8037065509359,-10.7749688230159,
-10.7058418005106,-10.6723987048533,-10.6427772116743,-10.6191131712757,
-10.5900743152024,-10.5145386260965,-10.5015478941132,-10.4473075308457,
-10.4243447954512,-10.4058650551817,-10.3931983270468,-10.3765805758244,
-10.3226581850168,-10.2460126486708,-10.2110859833837,-10.1805892538587,
-10.1568959033466,-10.128588281631,-10.0003736155827,-9.95534136766762,
-9.93918797693893,-9.92643540149527,-9.91017329198182,-9.86012475374465),
 .UNSPECIFIED.);
#857=B_SPLINE_CURVE_WITH_KNOTS('',3,(#84546,#84547,#84548,#84549,#84550,
#84551,#84552,#84553,#84554,#84555,#84556,#84557,#84558,#84559,#84560,#84561,
#84562,#84563,#84564,#84565,#84566,#84567,#84568,#84569,#84570,#84571,#84572,
#84573,#84574,#84575,#84576,#84577,#84578,#84579,#84580,#84581,#84582,#84583,
#84584,#84585,#84586,#84587,#84588,#84589,#84590,#84591,#84592,#84593,#84594,
#84595,#84596,#84597,#84598,#84599,#84600,#84601,#84602,#84603,#84604,#84605,
#84606,#84607,#84608,#84609,#84610,#84611,#84612,#84613,#84614,#84615,#84616,
#84617,#84618,#84619,#84620,#84621,#84622,#84623,#84624,#84625,#84626,#84627,
#84628,#84629,#84630,#84631,#84632,#84633,#84634,#84635,#84636,#84637,#84638,
#84639,#84640,#84641,#84642,#84643,#84644,#84645,#84646,#84647,#84648,#84649,
#84650,#84651,#84652,#84653,#84654,#84655,#84656,#84657,#84658,#84659,#84660,
#84661,#84662,#84663,#84664,#84665,#84666,#84667,#84668,#84669,#84670,#84671,
#84672,#84673,#84674,#84675,#84676,#84677,#84678,#84679,#84680,#84681,#84682,
#84683,#84684,#84685,#84686,#84687,#84688,#84689,#84690,#84691,#84692,#84693,
#84694,#84695,#84696,#84697,#84698,#84699,#84700,#84701,#84702,#84703,#84704,
#84705,#84706,#84707,#84708,#84709,#84710,#84711,#84712,#84713,#84714,#84715,
#84716,#84717,#84718,#84719,#84720,#84721,#84722,#84723,#84724,#84725,#84726,
#84727,#84728,#84729,#84730,#84731,#84732,#84733,#84734,#84735,#84736,#84737,
#84738,#84739,#84740,#84741,#84742,#84743,#84744,#84745,#84746,#84747,#84748,
#84749,#84750,#84751,#84752,#84753,#84754,#84755,#84756,#84757,#84758,#84759,
#84760,#84761,#84762,#84763,#84764,#84765,#84766,#84767,#84768,#84769,#84770,
#84771,#84772,#84773,#84774,#84775,#84776,#84777,#84778,#84779,#84780,#84781,
#84782,#84783,#84784,#84785,#84786,#84787,#84788,#84789,#84790,#84791,#84792,
#84793,#84794,#84795,#84796,#84797,#84798,#84799,#84800,#84801,#84802,#84803,
#84804,#84805,#84806,#84807,#84808,#84809,#84810,#84811,#84812,#84813,#84814,
#84815,#84816,#84817,#84818,#84819,#84820,#84821,#84822,#84823,#84824,#84825,
#84826,#84827,#84828,#84829,#84830,#84831,#84832,#84833,#84834,#84835,#84836,
#84837,#84838,#84839,#84840,#84841),.UNSPECIFIED.,.F.,.F.,(4,2,2,2,2,2,
2,2,2,2,2,2,2,2,2,2,2,2,2,2,2,2,2,2,2,2,2,2,2,2,2,2,2,2,2,2,2,2,2,2,2,2,
2,2,2,2,2,2,2,2,2,2,2,2,2,2,2,2,2,2,2,2,2,2,2,2,2,2,2,2,2,2,2,2,2,2,2,2,
2,2,2,2,2,2,2,2,2,2,2,2,2,2,2,2,2,2,2,2,2,2,2,2,2,2,2,2,2,2,2,2,2,2,2,2,
2,2,2,2,2,2,2,2,2,2,2,2,2,2,2,2,2,2,2,2,2,2,2,2,2,2,2,2,2,2,2,2,2,4),(-7.80730129127322,
-7.72626070803151,-7.7010822693862,-7.68344262614194,-7.65376820880232,
-7.63010261009414,-7.60111076828799,-7.48968140974421,-7.43188466833877,
-7.41490973134245,-7.40224583193526,-7.38383101509938,-7.28772569745943,
-7.23863452479943,-7.20055861038576,-7.17598471389478,-7.15371732777224,
-7.1145893216891,-7.01618875752558,-6.98220030310816,-6.95799161114217,
-6.94458131688635,-6.93020955348779,-6.90016498701403,-6.78420541842453,
-6.76372608325726,-6.73098929393947,-6.70711456424249,-6.68014729356618,
-6.6244319247151,-6.54099330071706,-6.51312896722129,-6.49196324499553,
-6.47902305637814,-6.46366139852171,-6.43102404018116,-6.3921140042867,
-6.3828728016361,-6.30179277408867,-6.26829252794629,-6.24433370615216,
-6.21770519992345,-6.16488740897721,-6.14781873464011,-6.07445189168421,
-6.04802116493502,-6.02761715835029,-6.01477537602664,-5.99906261136243,
-5.96089838110735,-5.88921372726034,-5.87222516816054,-5.82413357039492,
-5.79601889169422,-5.77231047110769,-5.74154799098932,-5.72291497052435,
-5.67087114022673,-5.63446608085268,-5.58157199415807,-5.56257499411121,
-5.54987477891329,-5.533334978487,-5.48332472992724,-5.38475873854658,-5.34624272353777,
-5.32405710250212,-5.29939539128026,-5.26071639208904,-5.23419256346272,
-5.13073009081111,-5.10454072761013,-5.09079717233722,-5.0768488704392,
-5.0494467043246,-5.00821659146785,-4.8983025910283,-4.86968351672077,-4.84623348659058,
-4.81626545227133,-4.7355749325088,-4.65241000009572,-4.63600142053206,
-4.6232278169302,-4.60719412831721,-4.56350114418109,-4.45700660607494,
-4.41867979288013,-4.39651931476581,-4.37182872781416,-4.33295255148146,
-4.28217884332469,-4.19043276846567,-4.17146627557357,-4.15876841884557,
-4.14220758361283,-4.0918874399943,-3.99326890603292,-3.95497042562246,
-3.93281373032131,-3.90811878823828,-3.86921273373862,-3.81837530397846,
-3.72385475547863,-3.70793706089702,-3.69522766568379,-3.67876860681528,
-3.62990008463346,-3.53157225065714,-3.49221893819145,-3.46992183369893,
-3.44537909090425,-3.40751491414312,-3.38187216716478,-3.28697109242537,
-3.25457842163597,-3.23925935398732,-3.22630551638532,-3.20503953442129,
-3.17698367024549,-3.09206456882485,-3.03767070147343,-3.01085483748964,
-2.98694536507005,-2.95388153121467,-2.91445600178413,-2.80569186649304,
-2.78341806290467,-2.7715995416598,-2.75731036407457,-2.72779742144896,
-2.68121261314395,-2.58403220313755,-2.55393779383181,-2.53026137975239,
-2.501635595418,-2.42425151436333,-2.33196494646441,-2.31638248565394,-2.3037060794182,
-2.28691440657283,-2.23282568172364,-2.11515125868408,-2.08686739980335,
-2.06317206648552,-2.03264264600147,-1.96001370979526,-1.91821254494555),
 .UNSPECIFIED.);
#858=B_SPLINE_CURVE_WITH_KNOTS('',3,(#84846,#84847,#84848,#84849,#84850,
#84851,#84852,#84853,#84854,#84855,#84856,#84857,#84858,#84859,#84860,#84861,
#84862,#84863,#84864,#84865,#84866,#84867,#84868,#84869,#84870,#84871,#84872,
#84873,#84874,#84875,#84876,#84877,#84878,#84879,#84880,#84881,#84882,#84883,
#84884,#84885,#84886,#84887,#84888,#84889,#84890,#84891,#84892,#84893,#84894,
#84895,#84896,#84897,#84898,#84899,#84900,#84901,#84902,#84903,#84904,#84905,
#84906,#84907,#84908,#84909,#84910,#84911,#84912,#84913,#84914,#84915,#84916,
#84917,#84918,#84919,#84920,#84921,#84922,#84923,#84924,#84925,#84926,#84927,
#84928,#84929,#84930,#84931,#84932,#84933,#84934,#84935,#84936,#84937,#84938,
#84939,#84940,#84941,#84942,#84943,#84944,#84945,#84946,#84947,#84948,#84949,
#84950,#84951,#84952,#84953,#84954,#84955,#84956,#84957,#84958,#84959,#84960,
#84961,#84962,#84963,#84964,#84965,#84966,#84967,#84968,#84969,#84970,#84971,
#84972,#84973,#84974,#84975,#84976,#84977,#84978,#84979,#84980,#84981,#84982,
#84983,#84984,#84985,#84986,#84987,#84988,#84989,#84990,#84991,#84992,#84993,
#84994,#84995,#84996,#84997,#84998,#84999,#85000,#85001,#85002,#85003,#85004,
#85005,#85006,#85007,#85008,#85009,#85010,#85011,#85012,#85013,#85014,#85015,
#85016,#85017,#85018,#85019,#85020,#85021,#85022,#85023,#85024,#85025,#85026,
#85027,#85028,#85029,#85030,#85031,#85032,#85033,#85034,#85035,#85036,#85037,
#85038,#85039,#85040,#85041,#85042,#85043,#85044,#85045,#85046,#85047,#85048,
#85049,#85050,#85051,#85052,#85053,#85054,#85055,#85056,#85057,#85058,#85059,
#85060,#85061,#85062,#85063,#85064,#85065,#85066,#85067,#85068,#85069,#85070,
#85071,#85072,#85073,#85074,#85075,#85076,#85077,#85078,#85079,#85080,#85081,
#85082,#85083,#85084,#85085,#85086,#85087,#85088,#85089,#85090,#85091,#85092,
#85093,#85094,#85095,#85096,#85097,#85098,#85099,#85100,#85101,#85102,#85103,
#85104,#85105,#85106,#85107,#85108,#85109,#85110,#85111,#85112,#85113,#85114,
#85115,#85116,#85117,#85118,#85119,#85120,#85121,#85122,#85123,#85124,#85125,
#85126,#85127,#85128,#85129,#85130,#85131,#85132,#85133,#85134,#85135,#85136,
#85137,#85138,#85139,#85140,#85141,#85142,#85143,#85144,#85145),
 .UNSPECIFIED.,.F.,.F.,(4,2,2,2,2,2,2,2,2,2,2,2,2,2,2,2,2,2,2,2,2,2,2,2,
2,2,2,2,2,2,2,2,2,2,2,2,2,2,2,2,2,2,2,2,2,2,2,2,2,2,2,2,2,2,2,2,2,2,2,2,
2,2,2,2,2,2,2,2,2,2,2,2,2,2,2,2,2,2,2,2,2,2,2,2,2,2,2,2,2,2,2,2,2,2,2,2,
2,2,2,2,2,2,2,2,2,2,2,2,2,2,2,2,2,2,2,2,2,2,2,2,2,2,2,2,2,2,2,2,2,2,2,2,
2,2,2,2,2,2,2,2,2,2,2,2,2,2,2,2,2,4),(-9.8600466769179,-9.84206584295104,
-9.79430053056243,-9.77278706780202,-9.75514611306556,-9.74374035233858,
-9.72732434117913,-9.67770771118887,-9.59775640398324,-9.5622363248628,
-9.53139320116547,-9.50768043446348,-9.47962362525768,-9.35764431995831,
-9.30670089523282,-9.29009870977196,-9.27740533364911,-9.26163699141251,
-9.1706516862146,-9.09252639283127,-9.06387052371785,-9.04019569192078,
-9.01013840244186,-8.91243686329657,-8.84726702784952,-8.82876592470117,
-8.81609803268091,-8.79949637671837,-8.74632813309397,-8.73373247455104,
-8.66489886320464,-8.63151756204156,-8.60193276709316,-8.57826917693296,
-8.54919598653495,-8.47445370961755,-8.382795493253,-8.36466988482914,-8.35201795540257,
-8.33511703818709,-8.28095016071714,-8.20492567263585,-8.1701142663127,
-8.13968501214976,-8.1159948466224,-8.08763574886608,-7.95968375768151,
-7.91456398152732,-7.89840293084959,-7.88565151964558,-7.86939832085296,
-7.77721892949442,-7.72556684497607,-7.70702233864676,-7.67635623416614,
-7.65265361993511,-7.62447047066011,-7.56248924296279,-7.48709766992981,
-7.46035999964738,-7.43979135923156,-7.42692949892786,-7.4112978538634,
-7.37357186022674,-7.2833181460758,-7.25821413681925,-7.24060880799932,
-7.21097249982408,-7.1873080957152,-7.15828261302411,-7.08521608330629,
-7.03157243862825,-6.98708575100017,-6.97098029202599,-6.95821961452808,
-6.94189975247792,-6.85702473987766,-6.85210149800976,-6.799249349395,-6.75941316163392,
-6.73458112984575,-6.70959952742261,-6.66875298260193,-6.57095507150738,
-6.52393579735874,-6.50761723821256,-6.49488964383261,-6.47556007015856,
-6.4185636006122,-6.34764494607684,-6.32531467145704,-6.29067099213656,
-6.26657284584925,-6.24037397369317,-6.19094286150453,-6.14691162042031,
-6.089548533163,-6.06594136975729,-6.04709518216505,-6.03451899219249,-6.01824476240093,
-5.97111573519495,-5.88917195261918,-5.83889056476543,-5.81258073154367,
-5.78852284640933,-5.75419725231639,-5.73218081449458,-5.66310093541642,
-5.65472823129876,-5.59811080858734,-5.58134289117328,-5.56868497150465,
-5.55039702061101,-5.48146309781162,-5.38829079710632,-5.35809650215912,
-5.334390859045,-5.30624678933474,-5.2375340976441,-5.16515432719394,-5.13108510646865,
-5.11549448602193,-5.1026217984588,-5.081967154605,-5.05506865657269,-4.97858870805779,
-4.91773408247829,-4.88964365055376,-4.86593346613737,-4.83513744712718,
-4.76040354563755,-4.67441673901827,-4.65581324173366,-4.64313956778014,
-4.62631353331931,-4.57158857672458,-4.454759122508,-4.42643406752544,-4.40274161142435,
-4.37226730420765,-4.27753378678927,-4.21180739773302,-4.19267462735229,
-4.17996384509378,-4.16351678919367,-4.11481223648704,-4.01652416287867,
-3.97704559273293,-3.97107570014323),.UNSPECIFIED.);
#859=B_SPLINE_CURVE_WITH_KNOTS('',3,(#85147,#85148,#85149,#85150,#85151,
#85152,#85153,#85154,#85155,#85156,#85157,#85158,#85159,#85160,#85161,#85162,
#85163,#85164,#85165,#85166,#85167,#85168,#85169,#85170,#85171,#85172,#85173,
#85174,#85175,#85176,#85177,#85178,#85179,#85180,#85181,#85182,#85183,#85184,
#85185,#85186,#85187,#85188,#85189,#85190,#85191,#85192,#85193,#85194,#85195,
#85196,#85197,#85198,#85199,#85200,#85201,#85202,#85203,#85204,#85205,#85206,
#85207,#85208,#85209,#85210,#85211,#85212,#85213,#85214,#85215,#85216,#85217,
#85218,#85219,#85220,#85221,#85222,#85223,#85224,#85225,#85226,#85227,#85228,
#85229,#85230,#85231,#85232,#85233,#85234,#85235,#85236,#85237,#85238,#85239,
#85240,#85241,#85242,#85243,#85244,#85245,#85246,#85247,#85248),
 .UNSPECIFIED.,.F.,.F.,(4,2,2,2,2,2,2,2,2,2,2,2,2,2,2,2,2,2,2,2,2,2,2,2,
2,2,2,2,2,2,2,2,2,2,2,2,2,2,2,2,2,2,2,2,2,2,2,2,2,2,4),(-1.91821254494555,
-1.86839903619994,-1.85276133308806,-1.84008019964067,-1.82334605577424,
-1.77027108258705,-1.6512336036067,-1.62301874449097,-1.59931853966615,
-1.56869598641094,-1.55019143328576,-1.49871569663207,-1.40578377547403,
-1.389705496664,-1.37697703585121,-1.36066464945206,-1.3137224669229,-1.21595229946101,
-1.17504082588153,-1.15004962676499,-1.12522652147238,-1.08545077294208,
-1.03273142049454,-0.941827689680017,-0.925862908919356,-0.913148172761548,
-0.89673304559461,-0.848459661708831,-0.75028302974387,-0.710468741360725,
-0.688109987795645,-0.665657646085728,-0.641409806040928,-0.606317324509801,
-0.5287690856591,-0.476739578401613,-0.460004654608429,-0.448135954610373,
-0.437461668385129,-0.40482392682485,-0.349255322368366,-0.322063337722082,
-0.260137630910478,-0.231948035731113,-0.208246000535885,-0.185278800870477,
-0.154617101514796,-0.0828852558936575,-0.0228474886777043,-0.00990135018824966,
-0.000147253532549841),.UNSPECIFIED.);
#860=B_SPLINE_CURVE_WITH_KNOTS('',3,(#85249,#85250,#85251,#85252,#85253,
#85254,#85255,#85256,#85257,#85258,#85259,#85260,#85261,#85262,#85263,#85264,
#85265,#85266,#85267,#85268,#85269,#85270,#85271,#85272,#85273,#85274,#85275,
#85276,#85277,#85278,#85279,#85280,#85281,#85282,#85283,#85284,#85285,#85286,
#85287,#85288,#85289,#85290,#85291,#85292,#85293,#85294,#85295,#85296,#85297,
#85298,#85299,#85300,#85301,#85302,#85303,#85304,#85305,#85306,#85307,#85308,
#85309,#85310,#85311,#85312,#85313,#85314,#85315,#85316,#85317,#85318,#85319,
#85320,#85321,#85322,#85323,#85324,#85325,#85326,#85327,#85328,#85329,#85330,
#85331,#85332,#85333,#85334,#85335,#85336,#85337,#85338,#85339,#85340,#85341,
#85342,#85343,#85344,#85345,#85346,#85347,#85348,#85349,#85350,#85351,#85352,
#85353,#85354,#85355,#85356,#85357,#85358,#85359,#85360,#85361,#85362,#85363,
#85364,#85365,#85366,#85367,#85368,#85369,#85370,#85371,#85372,#85373,#85374,
#85375,#85376,#85377,#85378,#85379,#85380,#85381,#85382,#85383,#85384,#85385,
#85386,#85387,#85388,#85389,#85390,#85391,#85392,#85393,#85394,#85395,#85396,
#85397,#85398,#85399,#85400,#85401,#85402,#85403,#85404,#85405,#85406,#85407,
#85408,#85409,#85410,#85411,#85412,#85413,#85414,#85415,#85416,#85417,#85418,
#85419,#85420,#85421,#85422,#85423,#85424,#85425,#85426,#85427,#85428,#85429,
#85430,#85431,#85432),.UNSPECIFIED.,.F.,.F.,(4,3,3,3,3,3,3,3,3,3,3,3,3,
3,3,3,3,3,3,3,3,3,3,3,3,3,3,3,3,3,3,3,3,3,3,3,3,3,3,3,3,3,3,3,3,3,3,3,3,
3,3,3,3,3,3,3,3,3,3,3,3,4),(84.8230016469244,84.8332951185895,84.9080939578295,
84.9828796919349,85.0576572721575,85.1324406751991,85.2072232860376,85.2820219961831,
85.3280131069056,85.4028119461453,85.4775976802505,85.5523752604729,85.6271586635142,
85.7019412743525,85.7767399844978,85.8227310952216,85.8975299344615,85.972315668567,
86.0470932487896,86.1218766518312,86.1966592626696,86.271457972815,86.3174490835376,
86.3922479227778,86.4670336568836,86.5418112371066,86.6165946401485,86.6913772509873,
86.766175961133,86.8121670718536,86.886965911092,86.9617516451959,87.036529225417,
87.111312628457,87.186095239294,87.2608939494379,87.3068850601697,87.3816838994136,
87.4564696335229,87.5312472137495,87.606030616795,87.6808132276374,87.7556119377866,
87.8016030484857,87.8764018877177,87.9511876218152,88.0259652020298,88.1007486050634,
88.1755312158941,88.2503299260317,88.2963210368017,88.3711198760534,88.4459056101707,
88.5206831904052,88.5954665934584,88.6702492043086,88.7450479144654,88.7910390251177,
88.8658384445578,88.9406237466334,89.0154044721172,89.0597207272658),
 .UNSPECIFIED.);
#861=B_SPLINE_CURVE_WITH_KNOTS('',3,(#85438,#85439,#85440,#85441,#85442,
#85443,#85444,#85445,#85446,#85447,#85448,#85449),.UNSPECIFIED.,.F.,.F.,
(4,1,1,1,1,1,1,1,1,4),(91.106186954104,91.4146581914001,91.9093761797161,
92.4040941680321,92.8988121563481,93.3935301446641,93.8882481329802,94.3829661212962,
94.8776841096122,95.3428995923426),.UNSPECIFIED.);
#862=B_SPLINE_CURVE_WITH_KNOTS('',3,(#85450,#85451,#85452,#85453,#85454,
#85455,#85456,#85457,#85458,#85459,#85460,#85461,#85462,#85463,#85464,#85465,
#85466,#85467,#85468,#85469,#85470,#85471,#85472,#85473,#85474,#85475,#85476,
#85477,#85478,#85479,#85480,#85481,#85482,#85483,#85484,#85485,#85486,#85487,
#85488,#85489,#85490,#85491,#85492,#85493,#85494,#85495,#85496,#85497,#85498,
#85499,#85500,#85501,#85502,#85503,#85504,#85505,#85506,#85507,#85508,#85509,
#85510,#85511,#85512,#85513,#85514,#85515,#85516,#85517,#85518,#85519,#85520,
#85521,#85522,#85523,#85524,#85525,#85526,#85527,#85528,#85529,#85530,#85531,
#85532,#85533,#85534,#85535,#85536,#85537,#85538,#85539,#85540,#85541,#85542,
#85543,#85544,#85545,#85546,#85547,#85548,#85549,#85550,#85551),
 .UNSPECIFIED.,.F.,.F.,(4,2,2,2,2,2,2,2,2,2,2,2,2,2,2,2,2,2,2,2,2,2,2,2,
2,2,2,2,2,2,2,2,2,2,2,2,2,2,2,2,2,2,2,2,2,2,2,2,2,2,4),(-11.7781008861112,
-11.6373344995044,-11.6204440228226,-11.6082405011693,-11.5955300900881,
-11.5764003055972,-11.521236726541,-11.448850777203,-11.4147410879726,-11.3853834696144,
-11.3650025297003,-11.3380786473167,-11.2870480504116,-11.1997437417241,
-11.1713879083436,-11.1552922460493,-11.1423547247261,-11.1294614398261,
-11.1077194521551,-10.9981785551021,-10.9586748743302,-10.9255678000331,
-10.901653876741,-10.8748578918298,-10.8226435275272,-10.7359207671394,
-10.6954923810874,-10.679781165207,-10.6669393575842,-10.6465333506768,
-10.5875984842728,-10.5771417319825,-10.5153295996795,-10.4946488797552,
-10.4617012485059,-10.4378046521462,-10.4109367477416,-10.356091672179,
-10.3188209767005,-10.2622824118571,-10.2461714752425,-10.223575498489,
-10.2104255409795,-10.1955967608558,-10.1624218729707,-10.0895319682909,
-10.0187614880707,-9.99048216776105,-9.96678687148919,-9.93677087038606,
-9.8600466769179),.UNSPECIFIED.);
#863=B_SPLINE_CURVE_WITH_KNOTS('',3,(#85553,#85554,#85555,#85556,#85557,
#85558,#85559,#85560,#85561,#85562,#85563,#85564,#85565,#85566,#85567,#85568,
#85569,#85570,#85571,#85572,#85573,#85574,#85575,#85576,#85577,#85578,#85579,
#85580,#85581,#85582,#85583,#85584,#85585,#85586,#85587,#85588,#85589,#85590,
#85591,#85592,#85593,#85594,#85595,#85596,#85597,#85598,#85599,#85600,#85601,
#85602,#85603,#85604,#85605,#85606,#85607,#85608,#85609,#85610,#85611,#85612,
#85613,#85614,#85615,#85616,#85617,#85618,#85619,#85620,#85621,#85622,#85623,
#85624,#85625,#85626,#85627,#85628,#85629,#85630,#85631,#85632,#85633,#85634,
#85635,#85636,#85637,#85638,#85639,#85640),.UNSPECIFIED.,.F.,.F.,(4,3,3,
3,3,3,3,3,3,3,3,3,3,3,3,3,3,3,3,3,3,3,3,3,3,3,3,3,3,4),(89.0597207272658,
89.1345030603627,89.2101300368982,89.2857570134337,89.3605558526666,89.4353415867648,
89.51011916698,89.5849025700143,89.6596851808455,89.7344838909835,89.7804750017498,
89.8552738410552,89.9300595752263,90.0048371555148,90.0796205586221,90.1544031695262,
90.2292018797362,90.2751929900658,90.3499918291084,90.4247775630155,90.4995551430398,
90.574338545884,90.6491211565263,90.7239198664782,90.7699109783818,90.844662845243,
90.9194034691721,90.9941340614828,91.0688657268607,91.106186954104),
 .UNSPECIFIED.);
#864=B_SPLINE_CURVE_WITH_KNOTS('',3,(#85641,#85642,#85643,#85644,#85645,
#85646,#85647,#85648,#85649,#85650,#85651,#85652,#85653,#85654,#85655,#85656,
#85657,#85658,#85659,#85660,#85661,#85662,#85663,#85664,#85665,#85666,#85667,
#85668,#85669,#85670,#85671,#85672,#85673,#85674,#85675,#85676,#85677,#85678,
#85679,#85680,#85681,#85682,#85683,#85684,#85685,#85686,#85687,#85688,#85689,
#85690,#85691,#85692,#85693,#85694,#85695,#85696,#85697,#85698,#85699,#85700,
#85701,#85702,#85703,#85704,#85705,#85706,#85707,#85708,#85709,#85710,#85711,
#85712,#85713,#85714,#85715,#85716,#85717,#85718,#85719,#85720,#85721,#85722,
#85723,#85724,#85725,#85726,#85727,#85728,#85729,#85730,#85731,#85732,#85733,
#85734,#85735,#85736,#85737,#85738,#85739,#85740,#85741,#85742,#85743,#85744,
#85745,#85746,#85747,#85748,#85749,#85750,#85751,#85752,#85753,#85754,#85755,
#85756,#85757,#85758,#85759,#85760,#85761,#85762,#85763,#85764,#85765,#85766,
#85767,#85768,#85769,#85770,#85771,#85772,#85773,#85774,#85775,#85776,#85777,
#85778,#85779,#85780,#85781,#85782,#85783,#85784,#85785,#85786,#85787,#85788,
#85789,#85790,#85791,#85792,#85793,#85794,#85795,#85796,#85797,#85798,#85799,
#85800,#85801,#85802,#85803,#85804,#85805,#85806,#85807,#85808,#85809,#85810,
#85811,#85812,#85813,#85814,#85815,#85816,#85817,#85818,#85819,#85820,#85821,
#85822,#85823,#85824,#85825,#85826,#85827,#85828,#85829,#85830,#85831,#85832,
#85833,#85834,#85835,#85836,#85837,#85838,#85839,#85840,#85841,#85842,#85843,
#85844,#85845,#85846),.UNSPECIFIED.,.F.,.F.,(4,2,2,2,2,2,2,2,2,2,2,2,2,
2,2,2,2,2,2,2,2,2,2,2,2,2,2,2,2,2,2,2,2,2,2,2,2,2,2,2,2,2,2,2,2,2,2,2,2,
2,2,2,2,2,2,2,2,2,2,2,2,2,2,2,2,2,2,2,2,2,2,2,2,2,2,2,2,2,2,2,2,2,2,2,2,
2,2,2,2,2,2,2,2,2,2,2,2,2,2,2,2,2,4),(3.97111550692216,3.97113291895875,
4.05886938220161,4.0753469959609,4.08813073331088,4.10410901890245,4.14720834959645,
4.24963595295934,4.29056238122401,4.31555593643396,4.34037718712831,4.38013965713478,
4.43282973021619,4.52464759682786,4.54026339947647,4.55294268108289,4.56969968345249,
4.62316945547823,4.74015577297554,4.76890125462364,4.7902047242648,4.8188615406612,
4.89700492592713,4.98797494789984,5.00374183230533,5.01643515394136,5.03303905472039,
5.08400744818666,5.20595262076944,5.2340115200502,5.25772426301847,5.28856482758201,
5.36213873326477,5.45026796838605,5.4666165203696,5.47938127320626,5.49546317426482,
5.53968671564407,5.59825383041793,5.60908745337636,5.66994420194613,5.69790110751523,
5.72162340382834,5.75261292456542,5.82892088851126,5.91398669658113,5.93031406258297,
5.94307581000045,5.9591751323507,6.00359319168067,6.0570361280124,6.13034059755623,
6.15938195459454,6.18304606453259,6.21266514967658,6.31223090855942,6.35175081649339,
6.38420996516903,6.39954059264249,6.41249050247763,6.4337284912338,6.46173099130339,
6.54623412483111,6.60099653493925,6.62785504108533,6.6517540685518,6.68472296091405,
6.72397753991101,6.83110222091231,6.85452882225789,6.86651426093276,6.88048691393189,
6.90803603368656,6.9877793691155,7.05848750832287,7.08725928390142,7.10856196329304,
7.11361305138611,7.11757744323573,7.12180840095472,7.12584174217891,7.13010887615431,
7.15838277076461,7.20673642095831,7.27959302486014,7.31290626717513,7.3277542678025,
7.33388097037029,7.34868294758195,7.36666252185189,7.40109222177752,7.52017794390152,
7.54964610547424,7.57248418053326,7.5997657930554,7.63094270208009,7.69014620826772,
7.76724077614046,7.78599033757201,7.79867295753841,7.81095914821328,7.82810653147107,
7.94206718808575),.UNSPECIFIED.);
#865=B_SPLINE_CURVE_WITH_KNOTS('',3,(#85852,#85853,#85854,#85855,#85856,
#85857,#85858,#85859,#85860,#85861,#85862,#85863,#85864,#85865,#85866,#85867,
#85868,#85869,#85870,#85871,#85872,#85873,#85874,#85875,#85876,#85877,#85878,
#85879,#85880,#85881,#85882,#85883,#85884,#85885,#85886,#85887,#85888,#85889,
#85890,#85891,#85892,#85893,#85894,#85895,#85896,#85897,#85898,#85899,#85900,
#85901,#85902,#85903,#85904,#85905,#85906,#85907,#85908,#85909,#85910,#85911,
#85912,#85913,#85914,#85915,#85916,#85917,#85918,#85919,#85920,#85921,#85922,
#85923,#85924,#85925,#85926,#85927,#85928,#85929,#85930,#85931,#85932,#85933,
#85934,#85935,#85936,#85937,#85938,#85939),.UNSPECIFIED.,.F.,.F.,(4,3,3,
3,3,3,3,3,3,3,3,3,3,3,3,3,3,3,3,3,3,3,3,3,3,3,3,3,3,4),(-4.09293042005646,
-4.0158857439365,-3.95774390652818,-3.88404094726653,-3.81035073834264,
-3.7366685538583,-3.66298068070267,-3.58929384691513,-3.51559086689293,
-3.46302591821216,-3.38932987780264,-3.3156465955138,-3.24197132533718,
-3.16829029817759,-3.09461026130577,-3.02091395433786,-2.96830792989613,
-2.89461009057983,-2.82092503805656,-2.74724803112181,-2.67356533033049,
-2.59988365776423,-2.52618578604003,-2.47358994158011,-2.4001630892653,
-2.326749936501,-2.25333914533707,-2.17993256163102,-2.10651636312689,-2.07410208625457),
 .UNSPECIFIED.);
#866=B_SPLINE_CURVE_WITH_KNOTS('',3,(#85942,#85943,#85944,#85945,#85946,
#85947),.UNSPECIFIED.,.F.,.F.,(4,1,1,4),(0.,0.494717988316024,0.989435976632052,
1.12274180646091),.UNSPECIFIED.);
#867=B_SPLINE_CURVE_WITH_KNOTS('',3,(#85952,#85953,#85954,#85955,#85956,
#85957,#85958,#85959,#85960,#85961,#85962,#85963,#85964,#85965,#85966,#85967,
#85968,#85969,#85970,#85971,#85972,#85973,#85974,#85975,#85976,#85977,#85978,
#85979,#85980,#85981,#85982,#85983,#85984,#85985,#85986,#85987,#85988,#85989,
#85990,#85991,#85992,#85993,#85994,#85995,#85996,#85997,#85998,#85999,#86000,
#86001,#86002,#86003,#86004,#86005,#86006,#86007,#86008,#86009,#86010,#86011,
#86012,#86013,#86014,#86015,#86016,#86017,#86018,#86019,#86020,#86021,#86022,
#86023,#86024,#86025,#86026,#86027,#86028,#86029,#86030,#86031,#86032,#86033,
#86034,#86035,#86036,#86037,#86038,#86039,#86040,#86041,#86042,#86043,#86044,
#86045,#86046,#86047,#86048,#86049,#86050,#86051,#86052,#86053,#86054,#86055,
#86056,#86057,#86058,#86059,#86060,#86061,#86062,#86063,#86064,#86065,#86066,
#86067,#86068,#86069,#86070,#86071,#86072,#86073,#86074,#86075,#86076,#86077,
#86078,#86079,#86080,#86081,#86082,#86083,#86084,#86085,#86086,#86087,#86088,
#86089,#86090,#86091,#86092,#86093,#86094,#86095,#86096,#86097,#86098,#86099,
#86100,#86101,#86102,#86103,#86104,#86105,#86106,#86107,#86108,#86109,#86110,
#86111,#86112,#86113,#86114,#86115,#86116,#86117,#86118,#86119,#86120,#86121,
#86122,#86123,#86124,#86125,#86126,#86127,#86128,#86129,#86130,#86131,#86132,
#86133,#86134,#86135,#86136,#86137,#86138,#86139,#86140,#86141,#86142,#86143,
#86144,#86145,#86146,#86147,#86148,#86149,#86150,#86151,#86152,#86153,#86154,
#86155,#86156,#86157,#86158,#86159,#86160,#86161,#86162,#86163,#86164,#86165,
#86166,#86167,#86168,#86169,#86170,#86171,#86172,#86173,#86174,#86175,#86176,
#86177,#86178,#86179,#86180,#86181,#86182,#86183,#86184,#86185,#86186,#86187,
#86188,#86189,#86190,#86191,#86192,#86193,#86194,#86195,#86196,#86197,#86198,
#86199,#86200,#86201,#86202,#86203,#86204,#86205,#86206,#86207,#86208,#86209,
#86210,#86211,#86212,#86213,#86214,#86215,#86216,#86217,#86218,#86219),
 .UNSPECIFIED.,.F.,.F.,(4,3,3,3,3,3,3,3,3,3,3,3,3,3,3,3,3,3,3,3,3,3,3,3,
3,3,3,3,3,3,3,3,3,3,3,3,3,3,3,3,3,3,3,3,3,3,3,3,3,3,3,3,3,3,3,3,3,3,3,3,
3,3,3,3,3,3,3,3,3,3,3,3,3,3,3,3,3,3,3,3,3,3,3,3,3,3,3,3,3,4),(-10.3761157273102,
-10.3025013652053,-10.2288999145983,-10.1553063912111,-10.0817072749245,
-10.0081084996647,-9.93449407177046,-9.89435976632045,-9.82066032120756,
-9.7469736341422,-9.67329496895587,-9.59961058593755,-9.52592722042616,
-9.45222765048504,-9.39964177800442,-9.32594233388247,-9.25225564780493,
-9.17857698360052,-9.10489260154891,-9.03120923699388,-8.95750966798643,
-8.9049237896884,-8.83122434794995,-8.75753766427595,-8.6838590024869,-8.61017462285223,
-8.53649126071152,-8.46279169409683,-8.41020580137238,-8.33650634776591,
-8.26281965216746,-8.18914097843315,-8.11545658690664,-8.04177321292283,
-7.96807363462363,-7.91548781305636,-7.8417883910061,-7.76810172708217,
-7.69442308504722,-7.62073872503153,-7.54705538240238,-7.4733558349973,
-7.42076982474033,-7.34707033959855,-7.27338361239049,-7.1997049070654,
-7.12602048420316,-7.05233707907581,-6.97863747014909,-6.92605183642431,
-6.85235244796297,-6.77866581764632,-6.70498720914059,-6.63130288229327,
-6.55761957257925,-6.48392005746314,-6.43133384810829,-6.35763436695287,
-6.28394764394594,-6.21026894302116,-6.13658452482969,-6.06290112451683,
-5.98920152059817,-5.93661585979227,-5.8629163313047,-5.7892295601607,-5.71555081044249,
-5.6418663428139,-5.56818289278328,-5.49448323904549,-5.44189787147625,
-5.36819885346765,-5.29451259553663,-5.22083436025188,-5.14715040521026,
-5.07346746591818,-4.99976831650723,-4.94717988316022,-4.87347930006267,
-4.79979147073412,-4.72611166235466,-4.65242614294801,-4.57874164666216,
-4.50504096253567,-4.4524618948442,-4.37893940144604,-4.30542631917865,
-4.23192289045638,-4.15841395294959,-4.09293042013065),.UNSPECIFIED.);
#868=B_SPLINE_CURVE_WITH_KNOTS('',3,(#86220,#86221,#86222,#86223,#86224,
#86225,#86226,#86227,#86228,#86229,#86230,#86231,#86232,#86233,#86234,#86235),
 .UNSPECIFIED.,.F.,.F.,(4,1,1,1,1,1,1,1,1,1,1,1,1,4),(1.12274180646091,
1.48415396494807,1.97887195326409,2.47358994158012,2.96830792989614,3.46302591821216,
3.95774390652818,4.4524618948442,4.94717988316022,5.44189787147624,5.93661585979226,
6.43133384810828,6.9260518364243,7.4059271136405),.UNSPECIFIED.);
#869=B_SPLINE_CURVE_WITH_KNOTS('',3,(#86240,#86241,#86242,#86243,#86244,
#86245,#86246,#86247,#86248,#86249,#86250,#86251,#86252,#86253,#86254,#86255,
#86256),.UNSPECIFIED.,.F.,.F.,(4,1,1,1,1,1,1,1,1,1,1,1,1,1,4),(-16.6593010344898,
-16.3256936144287,-15.8309756261127,-15.3362576377967,-14.8415396494807,
-14.3468216611646,-13.8521036728486,-13.3573856845326,-12.8626676962166,
-12.3679497079006,-11.8732317195845,-11.3785137312685,-10.8837957429525,
-10.3890777546365,-10.3761157273102),.UNSPECIFIED.);
#870=B_SPLINE_CURVE_WITH_KNOTS('',3,(#86257,#86258,#86259,#86260,#86261,
#86262,#86263,#86264,#86265,#86266,#86267,#86268,#86269,#86270,#86271,#86272,
#86273),.UNSPECIFIED.,.F.,.F.,(4,1,1,1,1,1,1,1,1,1,1,1,1,1,4),(7.4059271136405,
7.42076982474033,7.91548781305635,8.41020580137237,8.90492378968839,9.39964177800441,
9.89435976632044,10.3890777546365,10.8837957429525,11.3785137312685,11.8732317195845,
12.3679497079006,12.8626676962166,13.3573856845326,13.6891124208201),
 .UNSPECIFIED.);
#871=B_SPLINE_CURVE_WITH_KNOTS('',3,(#86278,#86279,#86280,#86281,#86282,
#86283,#86284,#86285,#86286,#86287,#86288,#86289,#86290,#86291,#86292,#86293,
#86294),.UNSPECIFIED.,.F.,.F.,(4,1,1,1,1,1,1,1,1,1,1,1,1,1,4),(-22.9424863074193,
-22.757027462537,-22.262309474221,-21.767591485905,-21.272873497589,-20.7781555092729,
-20.2834375209569,-19.7887195326409,-19.2940015443249,-18.7992835560088,
-18.3045655676928,-17.8098475793768,-17.3151295910608,-16.8204116027448,
-16.6593010344898),.UNSPECIFIED.);
#872=B_SPLINE_CURVE_WITH_KNOTS('',3,(#86295,#86296,#86297,#86298,#86299,
#86300,#86301,#86302,#86303,#86304,#86305,#86306,#86307,#86308,#86309,#86310,
#86311),.UNSPECIFIED.,.F.,.F.,(4,1,1,1,1,1,1,1,1,1,1,1,1,1,4),(13.6891124208201,
13.8521036728486,14.3468216611646,14.8415396494807,15.3362576377967,15.8309756261127,
16.3256936144287,16.8204116027448,17.3151295910608,17.8098475793768,18.3045655676928,
18.7992835560088,19.2940015443249,19.7887195326409,19.9722976935382),
 .UNSPECIFIED.);
#873=B_SPLINE_CURVE_WITH_KNOTS('',3,(#86316,#86317,#86318,#86319,#86320,
#86321,#86322,#86323,#86324,#86325,#86326,#86327,#86328,#86329,#86330,#86331,
#86332,#86333,#86334,#86335,#86336,#86337,#86338,#86339,#86340,#86341,#86342,
#86343,#86344,#86345,#86346,#86347,#86348,#86349,#86350,#86351,#86352,#86353,
#86354,#86355,#86356,#86357,#86358,#86359,#86360,#86361,#86362,#86363,#86364,
#86365,#86366,#86367,#86368,#86369,#86370,#86371,#86372,#86373,#86374,#86375,
#86376,#86377,#86378,#86379,#86380,#86381,#86382,#86383,#86384,#86385,#86386,
#86387,#86388,#86389,#86390,#86391,#86392,#86393,#86394,#86395,#86396,#86397,
#86398,#86399,#86400,#86401,#86402,#86403,#86404,#86405,#86406,#86407,#86408,
#86409,#86410,#86411,#86412,#86413,#86414,#86415,#86416,#86417,#86418,#86419,
#86420,#86421,#86422,#86423,#86424,#86425,#86426,#86427,#86428,#86429,#86430,
#86431,#86432,#86433,#86434,#86435,#86436,#86437,#86438,#86439,#86440,#86441,
#86442,#86443,#86444,#86445,#86446,#86447,#86448,#86449,#86450,#86451,#86452,
#86453,#86454,#86455,#86456,#86457,#86458,#86459,#86460,#86461,#86462,#86463,
#86464,#86465,#86466,#86467,#86468,#86469,#86470,#86471,#86472,#86473,#86474,
#86475,#86476,#86477,#86478,#86479,#86480,#86481,#86482,#86483,#86484,#86485,
#86486,#86487,#86488,#86489,#86490,#86491,#86492,#86493,#86494,#86495,#86496,
#86497,#86498,#86499,#86500,#86501,#86502,#86503,#86504,#86505,#86506,#86507,
#86508,#86509,#86510,#86511,#86512,#86513,#86514,#86515,#86516,#86517,#86518,
#86519,#86520,#86521,#86522,#86523,#86524,#86525,#86526,#86527,#86528,#86529,
#86530,#86531,#86532,#86533,#86534,#86535,#86536,#86537,#86538,#86539,#86540,
#86541,#86542,#86543,#86544,#86545,#86546,#86547,#86548,#86549,#86550,#86551,
#86552,#86553,#86554,#86555,#86556,#86557,#86558,#86559,#86560,#86561,#86562,
#86563,#86564,#86565,#86566,#86567,#86568,#86569,#86570,#86571,#86572,#86573,
#86574,#86575,#86576,#86577,#86578,#86579,#86580,#86581,#86582,#86583,#86584,
#86585,#86586),.UNSPECIFIED.,.F.,.F.,(4,3,3,3,3,3,3,3,3,3,3,3,3,3,3,3,3,
3,3,3,3,3,3,3,3,3,3,3,3,3,3,3,3,3,3,3,3,3,3,3,3,3,3,3,3,3,3,3,3,3,3,3,3,
3,3,3,3,3,3,3,3,3,3,3,3,3,3,3,3,3,3,3,3,3,3,3,3,3,3,3,3,3,3,3,3,3,3,3,3,
3,4),(-29.225671648849,-29.1883613106453,-29.1146618663602,-29.0409751801236,
-28.9672965157639,-28.8936121335643,-28.8199287688656,-28.7462291997225,
-28.6936433223293,-28.6199438780423,-28.5462571918037,-28.4725785274421,
-28.3988941452407,-28.3252107805401,-28.2515112113951,-28.1989253340133,
-28.125225889727,-28.051539203489,-27.9778605391277,-27.9041761569269,-27.830492792227,
-27.7567932230827,-27.7042073456973,-27.6305079014107,-27.5568212151724,
-27.4831425508109,-27.4094581686098,-27.3357748039096,-27.262075234765,
-27.2094893573812,-27.1357899130947,-27.0621032268566,-26.9884245624954,
-26.9147401802944,-26.8410568155944,-26.7673572464499,-26.7147713690652,
-26.6410719247788,-26.5673852385407,-26.4937065741796,-26.4200221919787,
-26.3463388272787,-26.2726392581342,-26.2200533807492,-26.1463539364628,
-26.0726672502246,-25.9989885858634,-25.9253042036624,-25.8516208389624,
-25.7779212698179,-25.7253353924332,-25.6516359481466,-25.5779492619084,
-25.5042705975471,-25.430586215346,-25.3569028506459,-25.2832032815013,
-25.2306174041171,-25.1569179598307,-25.0832312735925,-25.0095526092314,
-24.9358682270305,-24.8621848623305,-24.788485293186,-24.7358994158011,
-24.6621999715146,-24.5885132852765,-24.5148346209152,-24.4411502387143,
-24.3674668740142,-24.2937673048697,-24.2411814274851,-24.1674819831987,
-24.0937952969606,-24.0201166325994,-23.9464322503984,-23.8727488856986,
-23.7990493165541,-23.7464634391691,-23.6727639948825,-23.5990773086443,
-23.525398644283,-23.4517142620819,-23.3780308973818,-23.3043313282371,
-23.251745450853,-23.1744306735571,-23.1005806216386,-23.0267406498906,
-22.9529038759223,-22.9424863416694),.UNSPECIFIED.);
#874=B_SPLINE_CURVE_WITH_KNOTS('',3,(#86587,#86588,#86589,#86590,#86591,
#86592,#86593,#86594,#86595,#86596,#86597,#86598,#86599,#86600,#86601,#86602,
#86603,#86604,#86605,#86606,#86607,#86608,#86609,#86610,#86611,#86612,#86613,
#86614,#86615,#86616,#86617,#86618,#86619,#86620,#86621,#86622,#86623,#86624,
#86625,#86626,#86627,#86628,#86629,#86630,#86631,#86632,#86633,#86634,#86635,
#86636,#86637,#86638,#86639,#86640,#86641,#86642,#86643,#86644,#86645,#86646,
#86647,#86648,#86649,#86650,#86651,#86652,#86653,#86654,#86655,#86656,#86657,
#86658,#86659,#86660,#86661,#86662,#86663,#86664,#86665,#86666,#86667,#86668,
#86669,#86670,#86671,#86672,#86673,#86674,#86675,#86676,#86677,#86678,#86679,
#86680,#86681,#86682,#86683,#86684,#86685,#86686,#86687,#86688,#86689,#86690,
#86691,#86692,#86693,#86694,#86695,#86696,#86697,#86698,#86699,#86700,#86701,
#86702,#86703,#86704,#86705,#86706,#86707,#86708,#86709,#86710,#86711,#86712,
#86713,#86714,#86715,#86716,#86717,#86718,#86719,#86720,#86721,#86722,#86723,
#86724,#86725,#86726,#86727,#86728,#86729,#86730,#86731,#86732,#86733,#86734,
#86735,#86736,#86737,#86738,#86739,#86740,#86741,#86742,#86743,#86744,#86745,
#86746,#86747,#86748,#86749,#86750,#86751,#86752,#86753,#86754,#86755,#86756,
#86757,#86758,#86759,#86760,#86761,#86762,#86763,#86764,#86765,#86766,#86767,
#86768,#86769,#86770,#86771,#86772,#86773,#86774,#86775,#86776,#86777,#86778,
#86779,#86780,#86781,#86782,#86783,#86784,#86785,#86786,#86787,#86788,#86789,
#86790,#86791,#86792,#86793,#86794,#86795,#86796,#86797,#86798,#86799,#86800,
#86801,#86802,#86803,#86804,#86805,#86806,#86807,#86808,#86809,#86810,#86811,
#86812,#86813,#86814,#86815,#86816,#86817,#86818,#86819,#86820,#86821,#86822,
#86823,#86824,#86825,#86826,#86827,#86828,#86829,#86830,#86831,#86832,#86833,
#86834,#86835,#86836,#86837,#86838,#86839,#86840,#86841,#86842,#86843,#86844,
#86845,#86846,#86847,#86848,#86849,#86850,#86851,#86852,#86853,#86854,#86855,
#86856,#86857),.UNSPECIFIED.,.F.,.F.,(4,3,3,3,3,3,3,3,3,3,3,3,3,3,3,3,3,
3,3,3,3,3,3,3,3,3,3,3,3,3,3,3,3,3,3,3,3,3,3,3,3,3,3,3,3,3,3,3,3,3,3,3,3,
3,3,3,3,3,3,3,3,3,3,3,3,3,3,3,3,3,3,3,3,3,3,3,3,3,3,3,3,3,3,3,3,3,3,3,3,
3,4),(19.9722977279997,20.0461173438319,20.1199461706305,20.1937774306606,
20.2676235799437,20.2834375209569,20.3571369652434,20.4308236514814,20.5045023158425,
20.5781866980435,20.6518700627436,20.7255696318881,20.7781555092729,20.8518549535596,
20.925541639798,20.9992203041592,21.0729046863603,21.1465880510605,21.2202876202051,
21.272873497589,21.3465729418755,21.4202596281136,21.4939382924747,21.5676226746756,
21.6413060393754,21.7150056085199,21.767591485905,21.8412909301915,21.9149776164295,
21.9886562807907,22.0623406629917,22.1360240276917,22.2097235968362,22.262309474221,
22.3360089185075,22.4096956047458,22.4833742691071,22.557058651308,22.6307420160076,
22.7044415851521,22.757027462537,22.8307269068236,22.9044135930619,22.9780922574236,
23.0517766396246,23.1254600043248,23.1991595734695,23.2517454508531,23.3254448951396,
23.3991315813778,23.4728102457384,23.5464946279395,23.6201779926391,23.6938775617836,
23.7464634391691,23.8201628834554,23.8938495696935,23.9675282340557,24.0412126162567,
24.1148959809567,24.188595550101,24.2411814274851,24.3148808717717,24.3885675580098,
24.4622462223718,24.5359306045729,24.609613969273,24.6833135384175,24.7358994158011,
24.8095988600875,24.8832855463251,24.9569642106865,25.0306485928871,25.1043319575873,
25.1780315267316,25.2306174041171,25.3043168484037,25.3780035346426,25.4516821990037,
25.5253665812046,25.5990499459048,25.6727495150494,25.7253353924332,25.7990348367194,
25.8727215229571,25.9464001873184,26.0200845695193,26.09376793422,26.1674675033644,
26.2200533807492,26.2554830351793),.UNSPECIFIED.);
#875=B_SPLINE_CURVE_WITH_KNOTS('',3,(#86862,#86863,#86864,#86865,#86866,
#86867,#86868,#86869,#86870,#86871,#86872,#86873,#86874,#86875,#86876,#86877),
 .UNSPECIFIED.,.F.,.F.,(4,1,1,1,1,1,1,1,1,1,1,1,1,4),(-35.5088569560286,
-35.1249771704376,-34.6302591821216,-34.1355411938056,-33.6408232054895,
-33.1461052171735,-32.6513872288575,-32.1566692405415,-31.6619512522254,
-31.1672332639094,-30.6725152755934,-30.1777972872774,-29.6830792989613,
-29.2256716823632),.UNSPECIFIED.);
#876=B_SPLINE_CURVE_WITH_KNOTS('',3,(#86878,#86879,#86880,#86881,#86882,
#86883,#86884,#86885,#86886,#86887,#86888,#86889,#86890,#86891,#86892,#86893),
 .UNSPECIFIED.,.F.,.F.,(4,1,1,1,1,1,1,1,1,1,1,1,1,4),(26.2554830679407,
26.7147713690652,27.2094893573812,27.7042073456972,28.1989253340133,28.6936433223293,
29.1883613106453,29.6830792989613,30.1777972872774,30.6725152755934,31.1672332639094,
31.6619512522254,32.1566692405414,32.5386683423589),.UNSPECIFIED.);
#877=B_SPLINE_CURVE_WITH_KNOTS('',3,(#86898,#86899,#86900,#86901,#86902,
#86903,#86904,#86905,#86906,#86907,#86908,#86909,#86910,#86911,#86912,#86913,
#86914),.UNSPECIFIED.,.F.,.F.,(4,1,1,1,1,1,1,1,1,1,1,1,1,1,4),(-41.7920422544505,
-41.5563110185459,-41.0615930302299,-40.5668750419138,-40.0721570535978,
-39.5774390652818,-39.0827210769658,-38.5880030886497,-38.0932851003337,
-37.5985671120177,-37.1038491237017,-36.6091311353857,-36.1144131470696,
-35.6196951587536,-35.5088569560286),.UNSPECIFIED.);
#878=B_SPLINE_CURVE_WITH_KNOTS('',3,(#86915,#86916,#86917,#86918,#86919,
#86920,#86921,#86922,#86923,#86924,#86925,#86926,#86927,#86928,#86929,#86930,
#86931),.UNSPECIFIED.,.F.,.F.,(4,1,1,1,1,1,1,1,1,1,1,1,1,1,4),(32.5386683423589,
32.6513872288575,33.1461052171735,33.6408232054895,34.1355411938055,34.6302591821215,
35.1249771704376,35.6196951587536,36.1144131470696,36.6091311353856,37.1038491237017,
37.5985671120177,38.0932851003337,38.5880030886497,38.8218536394787),
 .UNSPECIFIED.);
#879=B_SPLINE_CURVE_WITH_KNOTS('',3,(#86936,#86937,#86938,#86939,#86940,
#86941,#86942,#86943,#86944,#86945,#86946,#86947,#86948,#86949,#86950,#86951,
#86952,#86953,#86954,#86955,#86956,#86957,#86958,#86959,#86960,#86961,#86962,
#86963,#86964,#86965,#86966,#86967,#86968,#86969,#86970,#86971,#86972,#86973,
#86974,#86975,#86976,#86977,#86978,#86979,#86980,#86981,#86982,#86983,#86984,
#86985,#86986,#86987,#86988,#86989,#86990,#86991,#86992,#86993,#86994,#86995,
#86996,#86997,#86998,#86999,#87000,#87001,#87002,#87003,#87004,#87005,#87006,
#87007,#87008,#87009,#87010,#87011,#87012,#87013,#87014,#87015,#87016,#87017,
#87018,#87019,#87020,#87021,#87022,#87023,#87024,#87025,#87026,#87027,#87028,
#87029,#87030,#87031,#87032,#87033,#87034,#87035,#87036,#87037,#87038,#87039,
#87040,#87041,#87042,#87043,#87044,#87045,#87046,#87047,#87048,#87049,#87050,
#87051,#87052,#87053,#87054,#87055,#87056,#87057,#87058,#87059,#87060,#87061,
#87062,#87063,#87064,#87065,#87066,#87067,#87068,#87069,#87070,#87071,#87072,
#87073,#87074,#87075,#87076,#87077,#87078,#87079,#87080,#87081,#87082,#87083,
#87084,#87085,#87086,#87087,#87088,#87089,#87090,#87091,#87092,#87093,#87094,
#87095,#87096,#87097,#87098,#87099,#87100,#87101,#87102,#87103,#87104,#87105,
#87106,#87107,#87108,#87109,#87110,#87111,#87112,#87113,#87114,#87115,#87116,
#87117,#87118,#87119,#87120,#87121,#87122,#87123,#87124,#87125,#87126,#87127,
#87128,#87129,#87130,#87131,#87132,#87133,#87134,#87135,#87136,#87137,#87138,
#87139,#87140,#87141,#87142,#87143,#87144,#87145,#87146,#87147,#87148,#87149,
#87150,#87151,#87152,#87153,#87154,#87155,#87156,#87157,#87158,#87159,#87160,
#87161,#87162,#87163,#87164,#87165,#87166,#87167,#87168,#87169,#87170,#87171,
#87172,#87173,#87174,#87175,#87176,#87177,#87178,#87179,#87180,#87181,#87182,
#87183,#87184,#87185,#87186,#87187,#87188,#87189,#87190,#87191,#87192,#87193,
#87194,#87195,#87196,#87197,#87198,#87199,#87200,#87201,#87202,#87203,#87204,
#87205,#87206),.UNSPECIFIED.,.F.,.F.,(4,3,3,3,3,3,3,3,3,3,3,3,3,3,3,3,3,
3,3,3,3,3,3,3,3,3,3,3,3,3,3,3,3,3,3,3,3,3,3,3,3,3,3,3,3,3,3,3,3,3,3,3,3,
3,3,3,3,3,3,3,3,3,3,3,3,3,3,3,3,3,3,3,3,3,3,3,3,3,3,3,3,3,3,3,3,3,3,3,3,
3,4),(-48.0752275703878,-47.9965820207153,-47.9876448666542,-47.9139454223674,
-47.840258736129,-47.7665800717675,-47.6928956895662,-47.6192123248658,
-47.545512755721,-47.4929268783381,-47.4192274340518,-47.3455407478136,
-47.2718620834526,-47.1981777012517,-47.1244943365519,-47.0507947674075,
-46.9982088900221,-46.9245094457356,-46.8508227594974,-46.7771440951362,
-46.7034597129352,-46.6297763482352,-46.5560767790907,-46.5034909017061,
-46.4297914574196,-46.3561047711814,-46.2824261068201,-46.2087417246192,
-46.1350583599191,-46.0613587907746,-46.0087729133901,-45.9350734691036,
-45.8613867828655,-45.7877081185043,-45.7140237363033,-45.6403403716033,
-45.5666408024589,-45.5140549250741,-45.4403554807875,-45.3666687945493,
-45.292990130188,-45.2193057479869,-45.1456223832868,-45.0719228141422,
-45.019336936758,-44.9456374924716,-44.8719508062334,-44.7982721418722,
-44.7245877596713,-44.6509043949712,-44.5772048258267,-44.524618948442,
-44.4509195041556,-44.3772328179174,-44.3035541535563,-44.2298697713553,
-44.1561864066553,-44.0824868375109,-44.029900960126,-43.9562015158396,
-43.8825148296014,-43.8088361652403,-43.7351517830394,-43.6614684183394,
-43.5877688491949,-43.53518297181,-43.4614835275234,-43.3877968412851,-43.3141181769239,
-43.2404337947228,-43.1667504300226,-43.093050860878,-43.0404649834939,
-42.9667655392075,-42.8930788529692,-42.819400188608,-42.7457158064071,
-42.6720324417071,-42.5983328725626,-42.5457469951779,-42.4720475508914,
-42.3983608646531,-42.3246822002922,-42.2509978180912,-42.177314453391,
-42.1036148842465,-42.0510290068619,-41.9765921073299,-41.9021699654454,
-41.8277591073817,-41.7920422632082),.UNSPECIFIED.);
#880=B_SPLINE_CURVE_WITH_KNOTS('',3,(#87207,#87208,#87209,#87210,#87211,
#87212,#87213,#87214,#87215,#87216,#87217,#87218,#87219,#87220,#87221,#87222,
#87223,#87224,#87225,#87226,#87227,#87228,#87229,#87230,#87231,#87232,#87233,
#87234,#87235,#87236,#87237,#87238,#87239,#87240,#87241,#87242,#87243,#87244,
#87245,#87246,#87247,#87248,#87249,#87250,#87251,#87252,#87253,#87254,#87255,
#87256,#87257,#87258,#87259,#87260,#87261,#87262,#87263,#87264,#87265,#87266,
#87267,#87268,#87269,#87270,#87271,#87272,#87273,#87274,#87275,#87276,#87277,
#87278,#87279,#87280,#87281,#87282,#87283,#87284,#87285,#87286,#87287,#87288,
#87289,#87290,#87291,#87292,#87293,#87294,#87295,#87296,#87297,#87298,#87299,
#87300,#87301,#87302,#87303,#87304,#87305,#87306,#87307,#87308,#87309,#87310,
#87311,#87312,#87313,#87314,#87315,#87316,#87317,#87318,#87319,#87320,#87321,
#87322,#87323,#87324,#87325,#87326,#87327,#87328,#87329,#87330,#87331,#87332,
#87333,#87334,#87335,#87336,#87337,#87338,#87339,#87340,#87341,#87342,#87343,
#87344,#87345,#87346,#87347,#87348,#87349,#87350,#87351,#87352,#87353,#87354,
#87355,#87356,#87357,#87358,#87359,#87360,#87361,#87362,#87363,#87364,#87365,
#87366,#87367,#87368,#87369,#87370,#87371,#87372,#87373,#87374,#87375,#87376,
#87377,#87378,#87379,#87380,#87381,#87382,#87383,#87384,#87385,#87386,#87387,
#87388,#87389,#87390,#87391,#87392,#87393,#87394,#87395,#87396,#87397,#87398,
#87399,#87400,#87401,#87402,#87403,#87404,#87405,#87406,#87407,#87408,#87409,
#87410,#87411,#87412,#87413,#87414,#87415,#87416,#87417,#87418,#87419,#87420,
#87421,#87422,#87423,#87424,#87425,#87426,#87427,#87428,#87429,#87430,#87431,
#87432,#87433,#87434,#87435,#87436,#87437,#87438,#87439,#87440,#87441,#87442,
#87443,#87444,#87445,#87446,#87447,#87448,#87449,#87450,#87451,#87452,#87453,
#87454,#87455,#87456,#87457,#87458,#87459,#87460,#87461,#87462,#87463,#87464,
#87465,#87466,#87467,#87468,#87469,#87470,#87471,#87472,#87473,#87474,#87475,
#87476,#87477),.UNSPECIFIED.,.F.,.F.,(4,3,3,3,3,3,3,3,3,3,3,3,3,3,3,3,3,
3,3,3,3,3,3,3,3,3,3,3,3,3,3,3,3,3,3,3,3,3,3,3,3,3,3,3,3,3,3,3,3,3,3,3,3,
3,3,3,3,3,3,3,3,3,3,3,3,3,3,3,3,3,3,3,3,3,3,3,3,3,3,3,3,3,3,3,3,3,3,3,3,
3,4),(38.8218536495384,38.8962424641098,38.9706355075857,39.0450460704514,
39.0827210769657,39.1564205212523,39.2301072074908,39.3037858718524,39.3774702540536,
39.4511536187539,39.5248531878985,39.5774390652818,39.6511385095681,39.7248251958061,
39.7985038601673,39.8721882423682,39.9458716070683,40.0195711762127,40.0721570535978,
40.1458564978843,40.2195431841225,40.2932218484837,40.3669062306847,40.4405895953846,
40.5142891645291,40.5668750419138,40.6405744862003,40.7142611724381,40.7879398367993,
40.8616242190003,40.9353075837005,41.009007152845,41.0615930302298,41.1352924745163,
41.2089791607543,41.2826578251155,41.3563422073166,41.4300255720167,41.5037251411614,
41.5563110185459,41.6300104628323,41.7036971490704,41.7773758134322,41.8510601956332,
41.924743560333,41.9984431294775,42.0510290068619,42.1247284511482,42.1984151373863,
42.2720938017479,42.3457781839489,42.419461548649,42.4931611177934,42.5457469951779,
42.6194464394643,42.6931331257019,42.7668117900624,42.8404961722633,42.9141795369633,
42.9878791061077,43.0404649834939,43.1141644277804,43.1878511140188,43.2615297783803,
43.3352141605814,43.4088975252817,43.4825970944261,43.53518297181,43.6088824160963,
43.6825691023342,43.7562477666954,43.8299321488965,43.9036155135963,43.9773150827406,
44.029900960126,44.1036004044123,44.1772870906506,44.2509657550119,44.3246501372129,
44.3983335019129,44.4720330710574,44.524618948442,44.5983183927284,44.6720050789663,
44.7456837433274,44.8193681255284,44.8930514902286,44.9667510593729,45.019336936758,
45.0980543814215,45.105038956718),.UNSPECIFIED.);
#881=B_SPLINE_CURVE_WITH_KNOTS('',3,(#87482,#87483,#87484,#87485,#87486,
#87487,#87488,#87489,#87490,#87491,#87492,#87493,#87494,#87495,#87496,#87497,
#87498,#87499,#87500,#87501,#87502,#87503,#87504,#87505,#87506,#87507,#87508,
#87509,#87510,#87511,#87512,#87513,#87514,#87515,#87516,#87517,#87518,#87519,
#87520,#87521,#87522,#87523,#87524,#87525,#87526,#87527,#87528,#87529,#87530,
#87531,#87532,#87533,#87534,#87535,#87536,#87537,#87538,#87539,#87540,#87541,
#87542,#87543,#87544,#87545,#87546,#87547,#87548,#87549,#87550,#87551,#87552,
#87553,#87554,#87555,#87556,#87557,#87558,#87559,#87560,#87561,#87562,#87563,
#87564,#87565,#87566,#87567,#87568,#87569,#87570,#87571,#87572,#87573,#87574,
#87575,#87576,#87577,#87578,#87579,#87580,#87581,#87582,#87583,#87584,#87585,
#87586,#87587,#87588,#87589,#87590,#87591,#87592,#87593,#87594,#87595,#87596,
#87597,#87598,#87599,#87600,#87601,#87602,#87603,#87604,#87605,#87606,#87607,
#87608,#87609,#87610,#87611,#87612,#87613,#87614,#87615,#87616,#87617,#87618,
#87619,#87620,#87621,#87622,#87623,#87624,#87625,#87626,#87627,#87628,#87629,
#87630,#87631,#87632,#87633,#87634,#87635,#87636,#87637,#87638,#87639,#87640,
#87641,#87642,#87643,#87644,#87645,#87646,#87647,#87648,#87649,#87650,#87651,
#87652,#87653,#87654,#87655,#87656,#87657,#87658,#87659,#87660,#87661,#87662,
#87663,#87664,#87665,#87666,#87667,#87668,#87669,#87670,#87671,#87672,#87673,
#87674,#87675,#87676,#87677,#87678,#87679,#87680,#87681,#87682,#87683,#87684,
#87685,#87686,#87687,#87688,#87689,#87690,#87691,#87692,#87693,#87694,#87695,
#87696,#87697,#87698,#87699,#87700,#87701,#87702,#87703,#87704,#87705,#87706,
#87707,#87708,#87709,#87710,#87711,#87712,#87713,#87714,#87715,#87716,#87717,
#87718,#87719,#87720,#87721,#87722,#87723,#87724,#87725,#87726,#87727,#87728,
#87729,#87730,#87731,#87732,#87733,#87734,#87735,#87736,#87737,#87738,#87739,
#87740,#87741,#87742,#87743,#87744,#87745,#87746,#87747,#87748,#87749),
 .UNSPECIFIED.,.F.,.F.,(4,3,3,3,3,3,3,3,3,3,3,3,3,3,3,3,3,3,3,3,3,3,3,3,
3,3,3,3,3,3,3,3,3,3,3,3,3,3,3,3,3,3,3,3,3,3,3,3,3,3,3,3,3,3,3,3,3,3,3,3,
3,3,3,3,3,3,3,3,3,3,3,3,3,3,3,3,3,3,3,3,3,3,3,3,3,3,3,3,3,4),(-54.3584128775674,
-54.2849899685177,-54.2115785832115,-54.1381640530566,-54.0647521810993,
-53.9913225211834,-53.9242607264464,-53.85056128216,-53.7768745959221,-53.703195931561,
-53.62951154936,-53.5558281846599,-53.4821286155154,-53.4295427381304,-53.355843293844,
-53.282156607606,-53.2084779432451,-53.1347935610442,-53.0611101963441,
-52.9874106271997,-52.9348247498144,-52.8611253055281,-52.7874386192901,
-52.7137599549282,-52.6400755727273,-52.5663922080273,-52.4926926388828,
-52.4401067614984,-52.3664073172119,-52.2927206309733,-52.2190419666122,
-52.1453575844111,-52.0716742197112,-51.9979746505666,-51.9453887731823,
-51.871689328896,-51.7980026426579,-51.7243239782976,-51.6506395960966,
-51.5769562313966,-51.5032566622521,-51.4506707848663,-51.3769713405799,
-51.3032846543415,-51.2296059899809,-51.1559216077799,-51.0822382430798,
-51.0085386739351,-50.9559527965503,-50.882253352264,-50.8085666660261,
-50.7348880016648,-50.6612036194638,-50.587520254764,-50.5138206856195,
-50.4612348082343,-50.3875353639481,-50.3138486777102,-50.2401700133499,
-50.1664856311489,-50.092802266449,-50.0191026973044,-49.9665168199183,
-49.8928173756317,-49.8191306893936,-49.7454520250325,-49.6717676428314,
-49.5980842781316,-49.5243847089868,-49.4717988316022,-49.3980993873157,
-49.3244127010775,-49.2507340367163,-49.1770496545154,-49.1033662898151,
-49.0296667206704,-48.9770808432862,-48.9033813989998,-48.8296947127613,
-48.7560160484013,-48.6823316662005,-48.6086483015005,-48.5349487323562,
-48.4823628549702,-48.4089545042359,-48.3355599148838,-48.262167220395,
-48.1887787589612,-48.115379492763,-48.0752275704749),.UNSPECIFIED.);
#882=B_SPLINE_CURVE_WITH_KNOTS('',3,(#87750,#87751,#87752,#87753,#87754,
#87755,#87756,#87757,#87758,#87759,#87760,#87761,#87762,#87763,#87764,#87765,
#87766,#87767,#87768,#87769,#87770,#87771,#87772,#87773,#87774,#87775,#87776,
#87777,#87778,#87779,#87780,#87781,#87782,#87783,#87784,#87785,#87786,#87787,
#87788,#87789,#87790,#87791,#87792,#87793,#87794,#87795,#87796,#87797,#87798,
#87799,#87800,#87801,#87802,#87803,#87804,#87805,#87806,#87807,#87808,#87809,
#87810,#87811,#87812,#87813,#87814,#87815,#87816,#87817,#87818,#87819,#87820,
#87821,#87822,#87823,#87824,#87825,#87826,#87827,#87828,#87829,#87830,#87831,
#87832,#87833,#87834,#87835,#87836,#87837,#87838,#87839,#87840,#87841,#87842,
#87843,#87844,#87845,#87846,#87847,#87848,#87849,#87850,#87851,#87852,#87853,
#87854,#87855,#87856,#87857,#87858,#87859,#87860,#87861,#87862,#87863,#87864,
#87865,#87866,#87867,#87868,#87869,#87870,#87871,#87872,#87873,#87874,#87875,
#87876,#87877,#87878,#87879,#87880,#87881,#87882,#87883,#87884,#87885,#87886,
#87887,#87888,#87889,#87890,#87891,#87892,#87893,#87894,#87895,#87896,#87897,
#87898,#87899,#87900,#87901,#87902,#87903,#87904,#87905,#87906,#87907,#87908,
#87909,#87910,#87911,#87912,#87913,#87914,#87915,#87916,#87917,#87918,#87919,
#87920,#87921,#87922,#87923,#87924,#87925,#87926,#87927,#87928,#87929,#87930,
#87931,#87932,#87933,#87934,#87935,#87936,#87937,#87938,#87939,#87940,#87941,
#87942,#87943,#87944,#87945,#87946,#87947,#87948,#87949,#87950,#87951,#87952,
#87953,#87954,#87955,#87956,#87957,#87958,#87959,#87960,#87961,#87962,#87963,
#87964,#87965,#87966,#87967,#87968,#87969,#87970,#87971,#87972,#87973,#87974,
#87975,#87976,#87977,#87978,#87979,#87980,#87981,#87982,#87983,#87984,#87985,
#87986,#87987,#87988,#87989,#87990,#87991,#87992,#87993,#87994,#87995,#87996,
#87997,#87998,#87999,#88000,#88001,#88002,#88003,#88004,#88005,#88006,#88007,
#88008,#88009,#88010,#88011,#88012,#88013,#88014,#88015,#88016,#88017),
 .UNSPECIFIED.,.F.,.F.,(4,3,3,3,3,3,3,3,3,3,3,3,3,3,3,3,3,3,3,3,3,3,3,3,
3,3,3,3,3,3,3,3,3,3,3,3,3,3,3,3,3,3,3,3,3,3,3,3,3,3,3,3,3,3,3,3,3,3,3,3,
3,3,3,3,3,3,3,3,3,3,3,3,3,3,3,3,3,3,3,3,3,3,3,3,3,3,3,3,3,4),(45.1050389568105,
45.1784373110113,45.2518258373623,45.3252185210999,45.3986103264318,45.4720183448909,
45.514054925074,45.5877543693606,45.661441055599,45.7351197199599,45.808804102161,
45.8824874668611,45.9561870360059,46.0087729133901,46.0824723576764,46.1561590439145,
46.2298377082755,46.3035220904764,46.3772054551767,46.4509050243212,46.5034909017061,
46.5771903459926,46.6508770322308,46.7245556965918,46.7982400787927,46.8719234434926,
46.9456230126372,46.9982088900221,47.0719083343085,47.1455950205465,47.2192736849076,
47.2929580671085,47.3666414318084,47.4403410009529,47.4929268783381,47.5666263226245,
47.6403130088627,47.7139916732241,47.7876760554253,47.8613594201254,47.9350589892702,
47.9876448666542,48.0613443109406,48.1350309971786,48.2087096615394,48.2823940437402,
48.3560774084403,48.4297769775848,48.4823628549702,48.5560622992565,48.6297489854944,
48.703427649855,48.7771120320559,48.8507953967557,48.9244949659001,48.9770808432862,
49.0507802875726,49.1244669738108,49.1981456381717,49.2718300203727,49.3455133850727,
49.4192129542173,49.4717988316022,49.5454982758885,49.6191849621266,49.6928636264875,
49.7665480086884,49.8402313733884,49.9139309425329,49.9665168199182,50.0402162642048,
50.1139029504433,50.1875816148053,50.2612659970064,50.334949361707,50.4086489308515,
50.4612348082343,50.5349342525207,50.6086209387594,50.6822996031205,50.7559839853216,
50.8296673500208,50.9033669191653,50.9559527965503,51.0293775994402,51.1027887792278,
51.1761997331969,51.2496062660259,51.3230273800014,51.3882242638976),
 .UNSPECIFIED.);
#883=B_SPLINE_CURVE_WITH_KNOTS('',3,(#88022,#88023,#88024,#88025,#88026,
#88027,#88028,#88029,#88030,#88031,#88032,#88033,#88034,#88035,#88036,#88037,
#88038),.UNSPECIFIED.,.F.,.F.,(4,1,1,1,1,1,1,1,1,1,1,1,1,1,4),(-60.641598184747,
-60.3555945745547,-59.8608765862387,-59.3661585979227,-58.8714406096067,
-58.3767226212906,-57.8820046329746,-57.3872866446586,-56.8925686563426,
-56.3978506680265,-55.9031326797105,-55.4084146913945,-54.9136967030785,
-54.4189787147625,-54.3584128775674),.UNSPECIFIED.);
#884=B_SPLINE_CURVE_WITH_KNOTS('',3,(#88039,#88040,#88041,#88042,#88043,
#88044,#88045,#88046,#88047,#88048,#88049,#88050,#88051,#88052,#88053,#88054,
#88055),.UNSPECIFIED.,.F.,.F.,(4,1,1,1,1,1,1,1,1,1,1,1,1,1,4),(51.3882242638976,
51.4506707848663,51.9453887731823,52.4401067614984,52.9348247498144,53.4295427381304,
53.9242607264464,54.4189787147624,54.9136967030785,55.4084146913945,55.9031326797105,
56.3978506680265,56.8925686563425,57.3872866446586,57.6714095710772),
 .UNSPECIFIED.);
#885=B_SPLINE_CURVE_WITH_KNOTS('',3,(#88060,#88061,#88062,#88063,#88064,
#88065,#88066,#88067,#88068,#88069,#88070,#88071,#88072,#88073,#88074,#88075,
#88076,#88077,#88078,#88079,#88080,#88081,#88082,#88083,#88084,#88085,#88086,
#88087,#88088,#88089,#88090,#88091,#88092,#88093,#88094,#88095,#88096,#88097,
#88098,#88099,#88100,#88101,#88102,#88103,#88104,#88105,#88106,#88107,#88108,
#88109,#88110,#88111,#88112,#88113,#88114,#88115,#88116,#88117,#88118,#88119,
#88120,#88121,#88122,#88123,#88124,#88125,#88126,#88127,#88128,#88129,#88130,
#88131,#88132,#88133,#88134,#88135,#88136,#88137,#88138,#88139,#88140,#88141,
#88142,#88143,#88144,#88145,#88146,#88147,#88148,#88149,#88150,#88151,#88152,
#88153,#88154,#88155,#88156,#88157,#88158,#88159,#88160,#88161,#88162,#88163,
#88164,#88165,#88166,#88167,#88168,#88169,#88170,#88171,#88172,#88173,#88174,
#88175,#88176,#88177,#88178,#88179,#88180,#88181,#88182,#88183,#88184,#88185,
#88186,#88187,#88188,#88189,#88190,#88191,#88192,#88193,#88194,#88195,#88196,
#88197,#88198,#88199,#88200,#88201,#88202,#88203,#88204,#88205,#88206,#88207,
#88208,#88209,#88210,#88211,#88212,#88213,#88214,#88215,#88216,#88217,#88218,
#88219,#88220,#88221,#88222,#88223,#88224,#88225,#88226,#88227,#88228,#88229,
#88230,#88231,#88232,#88233,#88234,#88235,#88236,#88237,#88238,#88239,#88240,
#88241,#88242,#88243,#88244,#88245,#88246,#88247,#88248,#88249,#88250,#88251,
#88252,#88253,#88254,#88255,#88256,#88257,#88258,#88259,#88260,#88261,#88262,
#88263,#88264,#88265,#88266,#88267,#88268,#88269,#88270,#88271,#88272,#88273,
#88274,#88275,#88276,#88277,#88278,#88279,#88280,#88281,#88282,#88283,#88284,
#88285,#88286,#88287,#88288,#88289,#88290,#88291,#88292,#88293,#88294,#88295,
#88296,#88297,#88298,#88299,#88300,#88301,#88302,#88303,#88304,#88305,#88306,
#88307,#88308,#88309,#88310,#88311,#88312,#88313,#88314,#88315,#88316,#88317,
#88318,#88319,#88320,#88321,#88322,#88323,#88324,#88325,#88326,#88327),
 .UNSPECIFIED.,.F.,.F.,(4,3,3,3,3,3,3,3,3,3,3,3,3,3,3,3,3,3,3,3,3,3,3,3,
3,3,3,3,3,3,3,3,3,3,3,3,3,3,3,3,3,3,3,3,3,3,3,3,3,3,3,3,3,3,3,3,3,3,3,3,
3,3,3,3,3,3,3,3,3,3,3,3,3,3,3,3,3,3,3,3,3,3,3,3,3,3,3,3,3,4),(-66.9247834918443,
-66.8478145143248,-66.786928422663,-66.7132289783763,-66.639542292138,-66.5658636277763,
-66.4921792455751,-66.4184958808748,-66.3447963117301,-66.292210434347,
-66.2185109900607,-66.1448243038226,-66.0711456394617,-65.9974612572609,
-65.923777892561,-65.8500783234165,-65.797492446031,-65.7237930017444,-65.650106315506,
-65.5764276511447,-65.5027432689435,-65.4290599042433,-65.3553603350986,
-65.3027744577149,-65.2290750134285,-65.1553883271904,-65.0817096628292,
-65.0080252806283,-64.9343419159282,-64.8606423467837,-64.8080564693989,
-64.7343570251125,-64.6606703388743,-64.5869916745131,-64.5133072923122,
-64.4396239276122,-64.3659243584678,-64.3133384810829,-64.2396390367964,
-64.1659523505581,-64.0922736861969,-64.0185893039959,-63.9449059392958,
-63.8712063701512,-63.8186204927669,-63.7449210484805,-63.6712343622425,
-63.5975556978814,-63.5238713156805,-63.4501879509805,-63.3764883818361,
-63.3239025044509,-63.2502030601643,-63.176516373926,-63.1028377095646,
-63.0291533273635,-62.9554699626634,-62.8817703935188,-62.8291845161348,
-62.7554850718484,-62.6817983856102,-62.608119721249,-62.5344353390481,
-62.4607519743481,-62.3870524052036,-62.3344665278188,-62.2607670835324,
-62.1870803972943,-62.1134017329332,-62.0397173507323,-61.9660339860323,
-61.8923344168878,-61.8397485395028,-61.7660490952164,-61.6923624089782,
-61.6186837446169,-61.5449993624159,-61.4713159977159,-61.3976164285713,
-61.3450305511868,-61.2713311069004,-61.1976444206621,-61.1239657563008,
-61.0502813740998,-60.9765980093998,-60.9028984402553,-60.8503125628708,
-60.7750416493584,-60.6997883345464,-60.6415981883296),.UNSPECIFIED.);
#886=B_SPLINE_CURVE_WITH_KNOTS('',3,(#88328,#88329,#88330,#88331,#88332,
#88333,#88334,#88335,#88336,#88337,#88338,#88339,#88340,#88341,#88342,#88343,
#88344,#88345,#88346,#88347,#88348,#88349,#88350,#88351,#88352,#88353,#88354,
#88355,#88356,#88357,#88358,#88359,#88360,#88361,#88362,#88363,#88364,#88365,
#88366,#88367,#88368,#88369,#88370,#88371,#88372,#88373,#88374,#88375,#88376,
#88377,#88378,#88379,#88380,#88381,#88382,#88383,#88384,#88385,#88386,#88387,
#88388,#88389,#88390,#88391,#88392,#88393,#88394,#88395,#88396,#88397,#88398,
#88399,#88400,#88401,#88402,#88403,#88404,#88405,#88406,#88407,#88408,#88409,
#88410,#88411,#88412,#88413,#88414,#88415,#88416,#88417,#88418,#88419,#88420,
#88421,#88422,#88423,#88424,#88425,#88426,#88427,#88428,#88429,#88430,#88431,
#88432,#88433,#88434,#88435,#88436,#88437,#88438,#88439,#88440,#88441,#88442,
#88443,#88444,#88445,#88446,#88447,#88448,#88449,#88450,#88451,#88452,#88453,
#88454,#88455,#88456,#88457,#88458,#88459,#88460,#88461,#88462,#88463,#88464,
#88465,#88466,#88467,#88468,#88469,#88470,#88471,#88472,#88473,#88474,#88475,
#88476,#88477,#88478,#88479,#88480,#88481,#88482,#88483,#88484,#88485,#88486,
#88487,#88488,#88489,#88490,#88491,#88492,#88493,#88494,#88495,#88496,#88497,
#88498,#88499,#88500,#88501,#88502,#88503,#88504,#88505,#88506,#88507,#88508,
#88509,#88510,#88511,#88512,#88513,#88514,#88515,#88516,#88517,#88518,#88519,
#88520,#88521,#88522,#88523,#88524,#88525,#88526,#88527,#88528,#88529,#88530,
#88531,#88532,#88533,#88534,#88535,#88536,#88537,#88538,#88539,#88540,#88541,
#88542,#88543,#88544,#88545,#88546,#88547,#88548,#88549,#88550,#88551,#88552,
#88553,#88554,#88555,#88556,#88557,#88558,#88559,#88560,#88561,#88562,#88563,
#88564,#88565,#88566,#88567,#88568,#88569,#88570,#88571,#88572,#88573,#88574,
#88575,#88576,#88577,#88578,#88579,#88580,#88581,#88582,#88583,#88584,#88585,
#88586,#88587,#88588,#88589,#88590,#88591,#88592,#88593,#88594,#88595),
 .UNSPECIFIED.,.F.,.F.,(4,3,3,3,3,3,3,3,3,3,3,3,3,3,3,3,3,3,3,3,3,3,3,3,
3,3,3,3,3,3,3,3,3,3,3,3,3,3,3,3,3,3,3,3,3,3,3,3,3,3,3,3,3,3,3,3,3,3,3,3,
3,3,3,3,3,3,3,3,3,3,3,3,3,3,3,3,3,3,3,3,3,3,3,3,3,3,3,3,3,4),(57.6714095742863,
57.7466199377083,57.8218544415793,57.8820046329746,57.9557040772608,58.0293907634987,
58.1030694278597,58.1767538100604,58.2504371747602,58.3241367439045,58.3767226212906,
58.4504220655772,58.5241087518157,58.5977874161769,58.671471798378,58.7451551630782,
58.8188547322229,58.8714406096067,58.9451400538932,59.0188267401314,59.0925054044924,
59.1661897866933,59.2398731513933,59.3135727205378,59.3661585979227,59.4398580422092,
59.5135447284473,59.5872233928085,59.6609077750095,59.7345911397095,59.808290708854,
59.8608765862387,59.9345760305252,60.0082627167634,60.0819413811247,60.1556257633256,
60.2293091280257,60.3030086971702,60.3555945745547,60.4292940188412,60.5029807050793,
60.5766593694405,60.6503437516414,60.7240271163415,60.797726685486,60.8503125628707,
60.9240120071571,60.9976986933953,61.0713773577564,61.1450617399574,61.2187451046574,
61.2924446738019,61.3450305511867,61.4187299954732,61.4924166817115,61.5660953460727,
61.6397797282737,61.7134630929739,61.7871626621185,61.8397485395028,61.9134479837892,
61.9871346700274,62.0608133343884,62.1344977165894,62.2081810812892,62.2818806504337,
62.3344665278188,62.4081659721052,62.4818526583434,62.5555313227047,62.6292157049056,
62.7028990696057,62.7765986387502,62.8291845161348,62.9028839604212,62.9765706466592,
63.0502493110202,63.1239336932211,63.1976170579211,63.2713166270657,63.3239025044508,
63.3976019487374,63.4712886349756,63.5449672993371,63.6186516815382,63.6923350462384,
63.7660346153831,63.8186204927669,63.8956443550278,63.9545948781802),
 .UNSPECIFIED.);
#887=B_SPLINE_CURVE_WITH_KNOTS('',3,(#88600,#88601,#88602,#88603,#88604,
#88605,#88606,#88607,#88608,#88609,#88610,#88611,#88612,#88613,#88614,#88615,
#88616,#88617,#88618,#88619,#88620,#88621,#88622,#88623,#88624,#88625,#88626,
#88627,#88628,#88629,#88630,#88631,#88632,#88633,#88634,#88635,#88636,#88637,
#88638,#88639,#88640,#88641,#88642,#88643,#88644,#88645,#88646,#88647,#88648,
#88649,#88650,#88651,#88652,#88653,#88654,#88655,#88656,#88657,#88658,#88659,
#88660,#88661,#88662,#88663,#88664,#88665,#88666,#88667,#88668,#88669,#88670,
#88671,#88672,#88673,#88674,#88675,#88676,#88677,#88678,#88679,#88680,#88681,
#88682,#88683,#88684,#88685,#88686,#88687,#88688,#88689,#88690,#88691,#88692,
#88693,#88694,#88695,#88696,#88697,#88698,#88699,#88700,#88701,#88702,#88703,
#88704,#88705,#88706,#88707,#88708,#88709,#88710,#88711,#88712,#88713,#88714,
#88715,#88716,#88717,#88718,#88719,#88720,#88721,#88722,#88723,#88724,#88725,
#88726,#88727,#88728,#88729,#88730,#88731,#88732,#88733,#88734,#88735,#88736,
#88737,#88738,#88739,#88740,#88741,#88742,#88743,#88744,#88745,#88746,#88747,
#88748,#88749,#88750,#88751,#88752,#88753,#88754,#88755,#88756,#88757,#88758,
#88759,#88760,#88761,#88762,#88763,#88764,#88765,#88766,#88767,#88768,#88769,
#88770,#88771,#88772,#88773,#88774,#88775,#88776,#88777,#88778,#88779,#88780,
#88781,#88782,#88783,#88784,#88785,#88786,#88787,#88788,#88789,#88790,#88791,
#88792,#88793,#88794,#88795,#88796,#88797,#88798,#88799,#88800,#88801,#88802,
#88803,#88804,#88805,#88806,#88807,#88808,#88809,#88810,#88811,#88812,#88813,
#88814,#88815,#88816,#88817,#88818,#88819,#88820,#88821,#88822,#88823,#88824,
#88825,#88826,#88827,#88828,#88829,#88830,#88831,#88832,#88833,#88834,#88835,
#88836,#88837,#88838,#88839,#88840,#88841,#88842,#88843,#88844,#88845,#88846,
#88847,#88848,#88849,#88850,#88851,#88852,#88853,#88854,#88855,#88856,#88857,
#88858,#88859,#88860,#88861,#88862,#88863,#88864,#88865,#88866,#88867),
 .UNSPECIFIED.,.F.,.F.,(4,3,3,3,3,3,3,3,3,3,3,3,3,3,3,3,3,3,3,3,3,3,3,3,
3,3,3,3,3,3,3,3,3,3,3,3,3,3,3,3,3,3,3,3,3,3,3,3,3,3,3,3,3,3,3,3,3,3,3,3,
3,3,3,3,3,3,3,3,3,3,3,3,3,3,3,3,3,3,3,3,3,3,3,3,3,3,3,3,3,4),(-73.2079687991061,
-73.1343380786446,-73.0607202596719,-72.9871104049237,-72.9134949479314,
-72.8398799780221,-72.7662492451856,-72.7235442824553,-72.6498448381687,
-72.5761581519305,-72.502479487569,-72.4287951053677,-72.3551117406675,
-72.2814121715227,-72.2288262941392,-72.1551268498529,-72.081440163615,
-72.0077614992544,-71.9340771170534,-71.8603937523532,-71.7866941832088,
-71.7341083058232,-71.6604088615369,-71.5867221752989,-71.5130435109382,
-71.4393591287373,-71.3656757640373,-71.2919761948928,-71.2393903175072,
-71.1656908732209,-71.0920041869828,-71.0183255226214,-70.9446411404204,
-70.8709577757201,-70.7972582065759,-70.7446723291912,-70.6709728849046,
-70.5972861986664,-70.5236075343048,-70.4499231521037,-70.3762397874038,
-70.3025402182592,-70.2499543408751,-70.1762548965886,-70.1025682103503,
-70.028889545989,-69.9552051637882,-69.8815217990882,-69.8078222299438,
-69.7552363525591,-69.6815369082727,-69.6078502220346,-69.534171557674,
-69.4604871754731,-69.3868038107734,-69.3131042416287,-69.2605183642431,
-69.1868189199567,-69.1131322337188,-69.039453569357,-68.9657691871559,
-68.8920858224556,-68.8183862533109,-68.7658003759271,-68.6921009316406,
-68.6184142454021,-68.544735581041,-68.4710511988402,-68.3973678341401,
-68.3236682649954,-68.2710823876111,-68.1973829433246,-68.1236962570865,
-68.0500175927256,-67.9763332105245,-67.9026498458241,-67.8289502766797,
-67.7763643992951,-67.7026649550085,-67.62897826877,-67.5552996044088,-67.4816152222079,
-67.4079318575082,-67.3342322883634,-67.281646410979,-67.2081092887614,
-67.134581747801,-67.0610638753131,-66.987541017849,-66.9247834919265),
 .UNSPECIFIED.);
#888=B_SPLINE_CURVE_WITH_KNOTS('',3,(#88868,#88869,#88870,#88871,#88872,
#88873,#88874,#88875,#88876,#88877,#88878,#88879,#88880,#88881,#88882,#88883,
#88884,#88885,#88886,#88887,#88888,#88889,#88890,#88891,#88892,#88893,#88894,
#88895,#88896,#88897,#88898,#88899,#88900,#88901,#88902,#88903,#88904,#88905,
#88906,#88907,#88908,#88909,#88910,#88911,#88912,#88913,#88914,#88915,#88916,
#88917,#88918,#88919,#88920,#88921,#88922,#88923,#88924,#88925,#88926,#88927,
#88928,#88929,#88930,#88931,#88932,#88933,#88934,#88935,#88936,#88937,#88938,
#88939,#88940,#88941,#88942,#88943,#88944,#88945,#88946,#88947,#88948,#88949,
#88950,#88951,#88952,#88953,#88954,#88955,#88956,#88957,#88958,#88959,#88960,
#88961,#88962,#88963,#88964,#88965,#88966,#88967,#88968,#88969,#88970,#88971,
#88972,#88973,#88974,#88975,#88976,#88977,#88978,#88979,#88980,#88981,#88982,
#88983,#88984,#88985,#88986,#88987,#88988,#88989,#88990,#88991,#88992,#88993,
#88994,#88995,#88996,#88997,#88998,#88999,#89000,#89001,#89002,#89003,#89004,
#89005,#89006,#89007,#89008,#89009,#89010,#89011,#89012,#89013,#89014,#89015,
#89016,#89017,#89018,#89019,#89020,#89021,#89022,#89023,#89024,#89025,#89026,
#89027,#89028,#89029,#89030,#89031,#89032,#89033,#89034,#89035,#89036,#89037,
#89038,#89039,#89040,#89041,#89042,#89043,#89044,#89045,#89046,#89047,#89048,
#89049,#89050,#89051,#89052,#89053,#89054,#89055,#89056,#89057,#89058,#89059,
#89060,#89061,#89062,#89063,#89064,#89065,#89066,#89067,#89068,#89069,#89070,
#89071,#89072,#89073,#89074,#89075,#89076,#89077,#89078,#89079,#89080,#89081,
#89082,#89083,#89084,#89085,#89086,#89087,#89088,#89089,#89090,#89091,#89092,
#89093,#89094,#89095,#89096,#89097,#89098,#89099,#89100,#89101,#89102,#89103,
#89104,#89105,#89106,#89107,#89108,#89109,#89110,#89111,#89112,#89113,#89114,
#89115,#89116,#89117,#89118,#89119,#89120,#89121,#89122,#89123,#89124,#89125,
#89126,#89127,#89128,#89129,#89130,#89131,#89132,#89133,#89134,#89135),
 .UNSPECIFIED.,.F.,.F.,(4,3,3,3,3,3,3,3,3,3,3,3,3,3,3,3,3,3,3,3,3,3,3,3,
3,3,3,3,3,3,3,3,3,3,3,3,3,3,3,3,3,3,3,3,3,3,3,3,3,3,3,3,3,3,3,3,3,3,3,3,
3,3,3,3,3,3,3,3,3,3,3,3,3,3,3,3,3,3,3,3,3,3,3,3,3,3,3,3,3,4),(63.9545948782568,
64.0281047268907,64.1016188939417,64.1751309958523,64.2486607942513,64.3133384810829,
64.3870379253694,64.4607246116078,64.5344032759691,64.6080876581701,64.6817710228699,
64.7554705920144,64.8080564693989,64.8817559136852,64.9554425999232,65.0291212642843,
65.1028056464851,65.176489011185,65.2501885803294,65.3027744577149,65.3764739020017,
65.4501605882402,65.5238392526012,65.5975236348023,65.6712069995025,65.7449065686472,
65.797492446031,65.8711918903174,65.9448785765557,66.0185572409169,66.0922416231179,
66.165924987818,66.2396245569625,66.292210434347,66.3659098786334,66.4395965648714,
66.5132752292325,66.5869596114334,66.6606429761336,66.7343425452781,66.786928422663,
66.8606278669494,66.9343145531879,67.0079932175491,67.08167759975,67.15536096445,
67.2290605335945,67.281646410979,67.3553458552654,67.4290325415035,67.5027112058644,
67.5763955880654,67.6500789527652,67.7237785219097,67.776364399295,67.8500638435817,
67.9237505298202,67.9974291941811,68.0711135763821,68.1447969410826,68.2184965102273,
68.2710823876111,68.3447818318976,68.4184685181356,68.492147182497,68.565831564698,
68.6395149293978,68.7132144985424,68.7658003759271,68.8394998202134,68.9131865064515,
68.9868651708136,69.0605495530148,69.1342329177144,69.2079324868591,69.2605183642431,
69.3342178085296,69.4079044947675,69.4815831591289,69.5552675413299,69.6289509060304,
69.7026504751748,69.7552363525591,69.828855753,69.902462147405,69.9760605064764,
70.0496643152218,70.1232676569756,70.1968865583481,70.2377801854364),
 .UNSPECIFIED.);
#889=B_SPLINE_CURVE_WITH_KNOTS('',3,(#89140,#89141,#89142,#89143,#89144,
#89145,#89146,#89147,#89148,#89149,#89150,#89151,#89152,#89153,#89154,#89155,
#89156),.UNSPECIFIED.,.F.,.F.,(4,1,1,1,1,1,1,1,1,1,1,1,1,1,4),(-79.4911541062857,
-79.1548781305636,-78.6601601422475,-78.1654421539315,-77.6707241656155,
-77.1760061772995,-76.6812881889835,-76.1865702006674,-75.6918522123514,
-75.1971342240354,-74.7024162357194,-74.2076982474033,-73.7129802590873,
-73.2182622707713,-73.2079687991061),.UNSPECIFIED.);
#890=B_SPLINE_CURVE_WITH_KNOTS('',3,(#89157,#89158,#89159,#89160,#89161,
#89162,#89163,#89164,#89165,#89166,#89167,#89168,#89169,#89170,#89171,#89172,
#89173,#89174),.UNSPECIFIED.,.F.,.F.,(4,2,1,1,1,1,1,1,1,1,1,1,1,1,4),(70.2377801854364,
70.2499543408751,70.7446723291912,71.2393903175072,71.7341083058232,72.2288262941392,
72.7235442824553,73.2182622707713,73.7129802590873,74.2076982474033,74.7024162357194,
75.1971342240354,75.6918522123514,76.1865702006674,76.520965492616),
 .UNSPECIFIED.);
#891=B_SPLINE_CURVE_WITH_KNOTS('',3,(#89179,#89180,#89181,#89182,#89183,
#89184,#89185,#89186,#89187,#89188,#89189,#89190,#89191,#89192,#89193,#89194,
#89195),.UNSPECIFIED.,.F.,.F.,(4,1,1,1,1,1,1,1,1,1,1,1,1,1,4),(-85.7743394134653,
-85.5862119786719,-85.0914939903558,-84.5967760020398,-84.1020580137238,
-83.6073400254078,-83.1126220370918,-82.6179040487757,-82.1231860604597,
-81.6284680721437,-81.1337500838277,-80.6390320955116,-80.1443141071956,
-79.6495961188796,-79.4911541062857),.UNSPECIFIED.);
#892=B_SPLINE_CURVE_WITH_KNOTS('',3,(#89196,#89197,#89198,#89199,#89200,
#89201,#89202,#89203,#89204,#89205,#89206,#89207,#89208,#89209,#89210,#89211,
#89212),.UNSPECIFIED.,.F.,.F.,(4,1,1,1,1,1,1,1,1,1,1,1,1,1,4),(76.520965492616,
76.6812881889834,77.1760061772995,77.6707241656155,78.1654421539315,78.6601601422475,
79.1548781305636,79.6495961188796,80.1443141071956,80.6390320955116,81.1337500838276,
81.6284680721437,82.1231860604597,82.6179040487757,82.8041507997956),
 .UNSPECIFIED.);
#893=B_SPLINE_CURVE_WITH_KNOTS('',3,(#89215,#89216,#89217,#89218,#89219,
#89220,#89221,#89222,#89223,#89224,#89225,#89226,#89227,#89228),
 .UNSPECIFIED.,.F.,.F.,(4,1,1,1,1,1,1,1,1,1,1,4),(82.8041507997956,83.1126220370917,
83.6073400254078,84.1020580137238,84.5967760020398,85.0914939903558,85.5862119786719,
86.0809299669879,86.5756479553039,87.0703659436199,87.5650839319359,87.9645943005142),
 .UNSPECIFIED.);
#894=B_SPLINE_CURVE_WITH_KNOTS('',3,(#89231,#89232,#89233,#89234,#89235,
#89236,#89237,#89238,#89239,#89240,#89241,#89242),.UNSPECIFIED.,.F.,.F.,
(4,1,1,1,1,1,1,1,1,4),(-90.0386738735161,-89.5439558852,-89.049237896884,
-88.554519908568,-88.059801920252,-87.565083931936,-87.0703659436199,-86.5756479553039,
-86.0809299669879,-85.7743394134653),.UNSPECIFIED.);
#895=B_SPLINE_CURVE_WITH_KNOTS('',3,(#89245,#89246,#89247,#89248,#89249,
#89250,#89251,#89252,#89253,#89254,#89255,#89256,#89257,#89258,#89259,#89260,
#89261,#89262,#89263,#89264,#89265,#89266,#89267,#89268,#89269,#89270,#89271,
#89272,#89273,#89274,#89275,#89276,#89277,#89278,#89279,#89280,#89281,#89282,
#89283,#89284,#89285,#89286,#89287,#89288,#89289,#89290,#89291,#89292,#89293,
#89294,#89295,#89296,#89297,#89298,#89299,#89300,#89301,#89302,#89303,#89304,
#89305,#89306,#89307,#89308,#89309,#89310,#89311,#89312,#89313,#89314,#89315,
#89316,#89317,#89318,#89319,#89320,#89321,#89322,#89323,#89324,#89325,#89326,
#89327,#89328,#89329,#89330,#89331,#89332,#89333,#89334,#89335,#89336,#89337,
#89338,#89339,#89340,#89341,#89342,#89343,#89344,#89345,#89346,#89347,#89348,
#89349,#89350,#89351,#89352,#89353,#89354,#89355,#89356,#89357,#89358,#89359,
#89360,#89361,#89362,#89363,#89364,#89365,#89366,#89367,#89368,#89369,#89370,
#89371,#89372,#89373,#89374,#89375,#89376,#89377,#89378,#89379,#89380,#89381,
#89382,#89383,#89384,#89385,#89386,#89387,#89388,#89389,#89390,#89391,#89392,
#89393,#89394,#89395,#89396,#89397,#89398,#89399,#89400,#89401,#89402,#89403,
#89404,#89405,#89406,#89407,#89408,#89409,#89410,#89411,#89412,#89413,#89414,
#89415,#89416,#89417,#89418,#89419,#89420,#89421,#89422,#89423,#89424,#89425,
#89426,#89427,#89428,#89429,#89430,#89431,#89432,#89433,#89434,#89435,#89436,
#89437,#89438,#89439,#89440,#89441,#89442,#89443,#89444,#89445,#89446,#89447,
#89448,#89449,#89450,#89451,#89452,#89453,#89454,#89455,#89456,#89457,#89458,
#89459,#89460,#89461,#89462,#89463,#89464,#89465,#89466,#89467,#89468,#89469,
#89470,#89471,#89472,#89473,#89474,#89475,#89476,#89477,#89478,#89479,#89480,
#89481,#89482,#89483,#89484,#89485,#89486,#89487,#89488,#89489,#89490,#89491,
#89492,#89493,#89494,#89495,#89496,#89497,#89498,#89499,#89500,#89501,#89502,
#89503,#89504,#89505,#89506,#89507,#89508,#89509,#89510),.UNSPECIFIED.,
 .F.,.F.,(4,2,2,2,2,2,2,2,2,2,2,2,2,2,2,2,2,2,2,2,2,2,2,2,2,2,2,2,2,2,2,
2,2,2,2,2,2,2,2,2,2,2,2,2,2,2,2,2,2,2,2,2,2,2,2,2,2,2,2,2,2,2,2,2,2,2,2,
2,2,2,2,2,2,2,2,2,2,2,2,2,2,2,2,2,2,2,2,2,2,2,2,2,2,2,2,2,2,2,2,2,2,2,2,
2,2,2,2,2,2,2,2,2,2,2,2,2,2,2,2,2,2,2,2,2,2,2,2,2,2,2,2,2,4),(0.000806536570366526,
0.0978003361637292,0.122342092926343,0.144799418030591,0.170108313118547,
0.212755320991058,0.311961287499786,0.341649545444072,0.350237546985673,
0.352689178741491,0.357656528872034,0.361646872304124,0.369787679675562,
0.382333782200091,0.401478017557775,0.456766923535376,0.507133058620796,
0.550622939497385,0.584005853074657,0.602887593835211,0.615707664529721,
0.64389890831545,0.768159170579458,0.802030575372541,0.819832498734995,
0.820510466711981,0.821147232581718,0.821747546569198,0.822315640753646,
0.822855301407632,0.823369932496131,0.823862611612536,0.824336139550256,
0.824793084584511,0.825235822466177,0.82566657306378,0.826087434577109,
0.826500416210535,0.826907470256461,0.827310524617655,0.827711516934067,
0.828112431733179,0.828515342373826,0.828922460087897,0.82933619324368,
0.829759221158954,0.830194588654903,0.830645830450056,0.831117139099606,
0.831613597758712,0.832141511881989,0.832708896547149,0.832988407388964,
0.833454442338801,0.834298637669974,0.834887291990056,0.837917198917195,
0.849841924882182,0.872904700728933,0.980586037635136,1.01991034241355,
1.05292365511241,1.07683603606502,1.1036947511368,1.15842606998003,1.17857090524075,
1.23687903608412,1.2815776031101,1.2977091084122,1.31047768007438,1.32680346737593,
1.41501023402502,1.46871813436071,1.508939195608,1.53382891132972,1.55875272082743,
1.59920151456328,1.69718527454096,1.7446997449492,1.76105644238005,1.77377592145688,
1.7897964777256,1.88298181221335,1.9343978888977,1.95288847865006,1.98349465481415,
2.00719076852861,2.03540940789467,2.09694696682855,2.17258861480466,2.19936264635097,
2.21995029942446,2.23281393268813,2.24843594844663,2.28271950079373,2.35505383464592,
2.42356416928124,2.45169641598032,2.47540641013983,2.5056264398898,2.59858526291233,
2.66907531156463,2.68671086066504,2.69811732658436,2.71454126798159,2.76432041916046,
2.84414567412818,2.87964328691644,2.91047271917343,2.93418332506308,2.96224620540681,
3.0841214683408,3.13514871107225,3.15175565772508,3.16444780888165,3.18334490460585,
3.27745398936972,3.32706045035602,3.36538391255637,3.38999416386613,3.41222778470923,
3.45110120676371,3.55670717924409,3.6002730318699,3.616295430426,3.62907171901554,
3.64549628961051,3.75045023678176,3.81546463042191,3.84333064507004,3.8670621649,
3.89764589794579,3.97111550692216),.UNSPECIFIED.);
#896=B_SPLINE_CURVE_WITH_KNOTS('',3,(#89514,#89515,#89516,#89517,#89518,
#89519,#89520,#89521,#89522,#89523,#89524,#89525,#89526,#89527,#89528,#89529,
#89530,#89531,#89532,#89533,#89534,#89535,#89536,#89537,#89538,#89539,#89540,
#89541,#89542,#89543,#89544,#89545,#89546,#89547,#89548,#89549,#89550,#89551,
#89552,#89553,#89554,#89555,#89556),.UNSPECIFIED.,.F.,.F.,(4,3,3,3,3,3,
3,3,3,3,3,3,3,3,4),(97.3893722664106,97.463731471798,97.5380780115012,97.615056518503,
97.6894051268309,97.76375727863,97.8381276809787,97.8459920395083,97.9212470945102,
97.9964884789106,98.0717196667722,98.1469501062026,98.2221751739854,98.2974062174588,
98.3407100278244),.UNSPECIFIED.);
#897=B_SPLINE_CURVE_WITH_KNOTS('',3,(#89557,#89558,#89559,#89560,#89561,
#89562,#89563,#89564,#89565),.UNSPECIFIED.,.F.,.F.,(4,1,1,1,1,1,4),(95.3428995923426,
95.3724020979282,95.8671200862443,96.3618380745603,96.8565560628763,97.3512740511923,
97.3893722612836),.UNSPECIFIED.);
#898=B_SPLINE_CURVE_WITH_KNOTS('',3,(#90306,#90307,#90308,#90309,#90310,
#90311,#90312,#90313,#90314,#90315,#90316,#90317,#90318,#90319,#90320,#90321,
#90322,#90323,#90324,#90325,#90326,#90327,#90328,#90329,#90330,#90331,#90332,
#90333,#90334,#90335,#90336,#90337,#90338,#90339,#90340,#90341,#90342,#90343,
#90344,#90345,#90346,#90347,#90348,#90349,#90350,#90351,#90352,#90353,#90354,
#90355,#90356,#90357,#90358,#90359,#90360,#90361,#90362,#90363,#90364,#90365,
#90366,#90367,#90368,#90369,#90370,#90371,#90372,#90373,#90374,#90375,#90376,
#90377,#90378,#90379,#90380,#90381,#90382,#90383,#90384,#90385,#90386,#90387,
#90388,#90389,#90390,#90391,#90392,#90393,#90394,#90395,#90396,#90397,#90398,
#90399,#90400,#90401,#90402,#90403,#90404,#90405,#90406,#90407,#90408,#90409,
#90410,#90411,#90412,#90413,#90414,#90415,#90416,#90417,#90418,#90419,#90420,
#90421,#90422,#90423),.UNSPECIFIED.,.F.,.F.,(4,3,3,3,3,3,3,3,3,3,3,3,3,
3,3,3,3,3,3,3,3,3,3,3,3,3,3,3,3,3,3,3,3,3,3,3,3,3,3,4),(3.9627874635238E-7,
0.0743187604012306,0.0947553987316233,0.168865895081324,0.24331753745554,
0.317543543810035,0.384132560472308,0.394183661157522,0.467915452531873,
0.541515418454756,0.583899610459125,0.657733552016035,0.731321143746018,
0.752263425776805,0.765228983131914,0.775235303088961,0.848353720857463,
0.921585303941482,0.99412411295158,1.06639765623861,1.12291086999283,1.13978254049866,
1.15333692391085,1.22526683640984,1.29857596887547,1.37106752217119,1.44478544422177,
1.51850336627235,1.52634774495678,1.54198813411966,1.6136839676136,1.68574649957796,
1.72631299944046,1.74783827110233,1.76349445406413,1.77572612606673,1.84737189178447,
1.91878510437671,1.9892523021272,2.01027849847794),.UNSPECIFIED.);
#899=B_SPLINE_CURVE_WITH_KNOTS('',3,(#90424,#90425,#90426,#90427,#90428,
#90429,#90430,#90431,#90432,#90433,#90434,#90435,#90436,#90437,#90438,#90439,
#90440,#90441,#90442,#90443,#90444,#90445,#90446,#90447,#90448,#90449,#90450,
#90451,#90452,#90453,#90454,#90455,#90456,#90457,#90458,#90459,#90460,#90461,
#90462,#90463,#90464,#90465,#90466,#90467,#90468,#90469,#90470,#90471,#90472,
#90473,#90474,#90475,#90476,#90477,#90478,#90479,#90480,#90481,#90482,#90483,
#90484,#90485,#90486,#90487,#90488,#90489,#90490,#90491,#90492,#90493,#90494,
#90495,#90496,#90497,#90498,#90499,#90500,#90501,#90502,#90503,#90504,#90505,
#90506,#90507,#90508,#90509,#90510,#90511,#90512,#90513,#90514,#90515,#90516,
#90517,#90518,#90519,#90520,#90521,#90522,#90523,#90524,#90525,#90526,#90527,
#90528,#90529,#90530,#90531,#90532,#90533,#90534,#90535,#90536,#90537,#90538,
#90539,#90540,#90541,#90542,#90543,#90544),.UNSPECIFIED.,.F.,.F.,(4,3,3,
3,3,3,3,3,3,3,3,3,3,3,3,3,3,3,3,3,3,3,3,3,3,3,3,3,3,3,3,3,3,3,3,3,3,3,3,
3,4),(-2.01027849847796,-1.93864883240901,-1.92070302042893,-1.84940600763368,
-1.79961994695732,-1.77688322270267,-1.7655613495308,-1.73844370067774,
-1.66642770916695,-1.59440274213944,-1.55318604449898,-1.52608655166908,
-1.51248154317586,-1.4511175222228,-1.37975752627662,-1.30728555503059,
-1.23463428834696,-1.16242067546908,-1.1463119704265,-1.09560707621285,
-1.02237008042034,-0.973988125444813,-0.901002560842819,-0.82780347338264,
-0.785600895008091,-0.772328125694967,-0.76155408296478,-0.688117520641271,
-0.614297719065266,-0.540711111505799,-0.490182846386249,-0.430056172450728,
-0.403750752603938,-0.389451921142354,-0.379313437087383,-0.306096966484562,
-0.231747457148313,-0.157301211215449,-0.0832353330587671,-0.00916945490208512,
-5.46117353640499E-15),.UNSPECIFIED.);
#900=B_SPLINE_CURVE_WITH_KNOTS('',3,(#91286,#91287,#91288,#91289,#91290,
#91291,#91292,#91293,#91294,#91295,#91296,#91297,#91298,#91299,#91300,#91301,
#91302,#91303,#91304,#91305,#91306,#91307,#91308,#91309,#91310,#91311,#91312,
#91313,#91314,#91315,#91316,#91317,#91318,#91319,#91320,#91321,#91322,#91323,
#91324,#91325,#91326,#91327,#91328,#91329,#91330,#91331,#91332,#91333,#91334,
#91335,#91336,#91337,#91338,#91339,#91340,#91341,#91342,#91343,#91344,#91345,
#91346,#91347,#91348,#91349,#91350,#91351,#91352,#91353,#91354,#91355,#91356,
#91357,#91358,#91359,#91360,#91361,#91362,#91363,#91364,#91365,#91366,#91367,
#91368,#91369,#91370,#91371,#91372,#91373,#91374,#91375,#91376,#91377,#91378,
#91379,#91380,#91381,#91382,#91383,#91384,#91385,#91386,#91387,#91388,#91389,
#91390,#91391,#91392,#91393,#91394,#91395,#91396,#91397,#91398,#91399,#91400,
#91401,#91402,#91403,#91404,#91405,#91406),.UNSPECIFIED.,.F.,.F.,(4,3,3,
3,3,3,3,3,3,3,3,3,3,3,3,3,3,3,3,3,3,3,3,3,3,3,3,3,3,3,3,3,3,3,3,3,3,3,3,
3,4),(0.,0.0716146571298102,0.0895455174761734,0.161056667463161,0.232704853117562,
0.304147485270842,0.339868801347482,0.357918124505382,0.366825163752922,
0.375590117424122,0.447629242845613,0.519979645211168,0.559487114576289,
0.63157350721065,0.703843799735493,0.73770758688256,0.745512094209105,0.818142982850016,
0.8910726172438,0.96376737166813,1.03603564877275,1.10887280851242,1.11368092827931,
1.12160931061262,1.19382320400099,1.26874221162545,1.34231143819719,1.41790533634802,
1.49349923449884,1.50227960552724,1.51891527711939,1.59200292456703,1.66575726114028,
1.70851112764835,1.73020926256932,1.74764381613927,1.76035480684199,1.78416451981067,
1.85850190150601,1.93314504735542,2.00778819320483),.UNSPECIFIED.);
#901=B_SPLINE_CURVE_WITH_KNOTS('',3,(#91407,#91408,#91409,#91410),
 .UNSPECIFIED.,.F.,.F.,(4,4),(0.,0.000711284740995393),.UNSPECIFIED.);
#902=B_SPLINE_CURVE_WITH_KNOTS('',3,(#91411,#91412,#91413,#91414,#91415,
#91416,#91417,#91418,#91419,#91420,#91421,#91422,#91423,#91424,#91425,#91426,
#91427,#91428,#91429,#91430,#91431,#91432,#91433,#91434,#91435,#91436,#91437,
#91438,#91439,#91440,#91441,#91442,#91443,#91444,#91445,#91446,#91447,#91448,
#91449,#91450,#91451,#91452,#91453,#91454,#91455,#91456,#91457,#91458,#91459,
#91460,#91461,#91462,#91463,#91464,#91465,#91466,#91467,#91468,#91469,#91470,
#91471,#91472,#91473,#91474,#91475,#91476,#91477,#91478,#91479,#91480,#91481,
#91482,#91483,#91484,#91485,#91486,#91487,#91488,#91489,#91490,#91491,#91492,
#91493,#91494,#91495,#91496,#91497,#91498,#91499,#91500,#91501,#91502,#91503,
#91504,#91505,#91506,#91507,#91508,#91509,#91510,#91511,#91512,#91513,#91514,
#91515,#91516,#91517,#91518,#91519,#91520,#91521,#91522,#91523,#91524,#91525,
#91526,#91527,#91528,#91529,#91530,#91531),.UNSPECIFIED.,.F.,.F.,(4,3,3,
3,3,3,3,3,3,3,3,3,3,3,3,3,3,3,3,3,3,3,3,3,3,3,3,3,3,3,3,3,3,3,3,3,3,3,3,
3,4),(-2.00778819320479,-1.93363330609131,-1.91321255832737,-1.83897355307137,
-1.76467605789325,-1.75162085734409,-1.74164675852145,-1.67739297918314,
-1.60348492023008,-1.53028776793595,-1.49971429773937,-1.49060173162983,
-1.42561568789313,-1.35278602352358,-1.27922221004438,-1.20576872343774,
-1.13312878374067,-1.11692732896057,-1.10856339625353,-1.03571490313795,
-0.96298798677832,-0.943739908687974,-0.870803091850739,-0.797994780817984,
-0.756800525433452,-0.743508832763832,-0.732449565606889,-0.660202669875926,
-0.58787384738682,-0.516205504225887,-0.468440737741721,-0.410352915438056,
-0.384939493180202,-0.37128601545293,-0.360693101664746,-0.28954884186388,
-0.217764646472875,-0.146189250061888,-0.0749637046871438,-0.00373815931239996,
0.),.UNSPECIFIED.);
#948=SHAPE_REPRESENTATION_RELATIONSHIP('SRR','None',#94500,#963);
#963=ADVANCED_BREP_SHAPE_REPRESENTATION('',(#993),#94409);
#978=STYLED_ITEM('',(#94577),#993);
#993=MANIFOLD_SOLID_BREP('Body1',#8263);
#1047=FACE_BOUND('',#1896,.T.);
#1048=FACE_BOUND('',#1900,.T.);
#1049=FACE_BOUND('',#1902,.T.);
#1151=PLANE('',#8880);
#1152=PLANE('',#8887);
#1153=PLANE('',#8888);
#1456=FACE_OUTER_BOUND('',#1863,.T.);
#1457=FACE_OUTER_BOUND('',#1864,.T.);
#1458=FACE_OUTER_BOUND('',#1865,.T.);
#1459=FACE_OUTER_BOUND('',#1866,.T.);
#1460=FACE_OUTER_BOUND('',#1867,.T.);
#1461=FACE_OUTER_BOUND('',#1868,.T.);
#1462=FACE_OUTER_BOUND('',#1869,.T.);
#1463=FACE_OUTER_BOUND('',#1870,.T.);
#1464=FACE_OUTER_BOUND('',#1871,.T.);
#1465=FACE_OUTER_BOUND('',#1872,.T.);
#1466=FACE_OUTER_BOUND('',#1873,.T.);
#1467=FACE_OUTER_BOUND('',#1874,.T.);
#1468=FACE_OUTER_BOUND('',#1875,.T.);
#1469=FACE_OUTER_BOUND('',#1876,.T.);
#1470=FACE_OUTER_BOUND('',#1877,.T.);
#1471=FACE_OUTER_BOUND('',#1878,.T.);
#1472=FACE_OUTER_BOUND('',#1879,.T.);
#1473=FACE_OUTER_BOUND('',#1880,.T.);
#1474=FACE_OUTER_BOUND('',#1881,.T.);
#1475=FACE_OUTER_BOUND('',#1882,.T.);
#1476=FACE_OUTER_BOUND('',#1883,.T.);
#1477=FACE_OUTER_BOUND('',#1884,.T.);
#1478=FACE_OUTER_BOUND('',#1885,.T.);
#1479=FACE_OUTER_BOUND('',#1886,.T.);
#1480=FACE_OUTER_BOUND('',#1887,.T.);
#1481=FACE_OUTER_BOUND('',#1888,.T.);
#1482=FACE_OUTER_BOUND('',#1889,.T.);
#1483=FACE_OUTER_BOUND('',#1890,.T.);
#1484=FACE_OUTER_BOUND('',#1891,.T.);
#1485=FACE_OUTER_BOUND('',#1892,.T.);
#1486=FACE_OUTER_BOUND('',#1893,.T.);
#1487=FACE_OUTER_BOUND('',#1894,.T.);
#1488=FACE_OUTER_BOUND('',#1895,.T.);
#1489=FACE_OUTER_BOUND('',#1897,.T.);
#1490=FACE_OUTER_BOUND('',#1898,.T.);
#1491=FACE_OUTER_BOUND('',#1899,.T.);
#1492=FACE_OUTER_BOUND('',#1901,.T.);
#1863=EDGE_LOOP('',(#7296,#7297,#7298,#7299));
#1864=EDGE_LOOP('',(#7300,#7301,#7302,#7303,#7304,#7305));
#1865=EDGE_LOOP('',(#7306,#7307,#7308,#7309,#7310));
#1866=EDGE_LOOP('',(#7311,#7312,#7313,#7314,#7315));
#1867=EDGE_LOOP('',(#7316,#7317,#7318,#7319,#7320,#7321));
#1868=EDGE_LOOP('',(#7322,#7323,#7324,#7325,#7326));
#1869=EDGE_LOOP('',(#7327,#7328,#7329,#7330,#7331));
#1870=EDGE_LOOP('',(#7332,#7333,#7334,#7335,#7336,#7337));
#1871=EDGE_LOOP('',(#7338,#7339,#7340,#7341,#7342));
#1872=EDGE_LOOP('',(#7343,#7344,#7345,#7346,#7347));
#1873=EDGE_LOOP('',(#7348,#7349,#7350,#7351,#7352));
#1874=EDGE_LOOP('',(#7353,#7354,#7355,#7356,#7357));
#1875=EDGE_LOOP('',(#7358,#7359,#7360,#7361,#7362));
#1876=EDGE_LOOP('',(#7363,#7364,#7365,#7366,#7367,#7368));
#1877=EDGE_LOOP('',(#7369,#7370,#7371,#7372));
#1878=EDGE_LOOP('',(#7373,#7374,#7375,#7376));
#1879=EDGE_LOOP('',(#7377,#7378,#7379,#7380));
#1880=EDGE_LOOP('',(#7381,#7382,#7383,#7384));
#1881=EDGE_LOOP('',(#7385,#7386,#7387,#7388));
#1882=EDGE_LOOP('',(#7389,#7390,#7391,#7392));
#1883=EDGE_LOOP('',(#7393,#7394,#7395,#7396));
#1884=EDGE_LOOP('',(#7397,#7398,#7399,#7400));
#1885=EDGE_LOOP('',(#7401,#7402,#7403,#7404));
#1886=EDGE_LOOP('',(#7405,#7406,#7407,#7408));
#1887=EDGE_LOOP('',(#7409,#7410,#7411,#7412));
#1888=EDGE_LOOP('',(#7413,#7414,#7415,#7416));
#1889=EDGE_LOOP('',(#7417,#7418,#7419,#7420));
#1890=EDGE_LOOP('',(#7421,#7422,#7423,#7424));
#1891=EDGE_LOOP('',(#7425,#7426,#7427,#7428));
#1892=EDGE_LOOP('',(#7429,#7430,#7431,#7432,#7433));
#1893=EDGE_LOOP('',(#7434,#7435,#7436,#7437,#7438,#7439,#7440,#7441,#7442,
#7443,#7444,#7445,#7446,#7447,#7448,#7449,#7450,#7451,#7452,#7453,#7454,
#7455,#7456,#7457,#7458,#7459,#7460,#7461,#7462,#7463,#7464,#7465,#7466,
#7467,#7468,#7469,#7470,#7471,#7472,#7473,#7474));
#1894=EDGE_LOOP('',(#7475,#7476,#7477,#7478,#7479,#7480,#7481,#7482,#7483,
#7484,#7485,#7486,#7487,#7488,#7489,#7490,#7491,#7492,#7493,#7494,#7495,
#7496,#7497,#7498,#7499,#7500,#7501,#7502,#7503,#7504,#7505,#7506,#7507,
#7508,#7509,#7510,#7511,#7512,#7513,#7514,#7515,#7516));
#1895=EDGE_LOOP('',(#7517));
#1896=EDGE_LOOP('',(#7518,#7519,#7520,#7521));
#1897=EDGE_LOOP('',(#7522,#7523,#7524,#7525));
#1898=EDGE_LOOP('',(#7526,#7527,#7528,#7529));
#1899=EDGE_LOOP('',(#7530,#7531,#7532,#7533,#7534));
#1900=EDGE_LOOP('',(#7535));
#1901=EDGE_LOOP('',(#7536));
#1902=EDGE_LOOP('',(#7537));
#2287=LINE('',#79157,#2685);
#2288=LINE('',#79394,#2686);
#2289=LINE('',#79793,#2687);
#2290=LINE('',#80314,#2688);
#2291=LINE('',#80739,#2689);
#2292=LINE('',#81070,#2690);
#2293=LINE('',#81588,#2691);
#2294=LINE('',#81998,#2692);
#2295=LINE('',#82393,#2693);
#2296=LINE('',#82942,#2694);
#2297=LINE('',#83579,#2695);
#2298=LINE('',#84226,#2696);
#2299=LINE('',#84845,#2697);
#2300=LINE('',#85436,#2698);
#2301=LINE('',#85850,#2699);
#2302=LINE('',#85951,#2700);
#2303=LINE('',#86239,#2701);
#2304=LINE('',#86277,#2702);
#2305=LINE('',#86315,#2703);
#2306=LINE('',#86861,#2704);
#2307=LINE('',#86897,#2705);
#2308=LINE('',#86935,#2706);
#2309=LINE('',#87481,#2707);
#2310=LINE('',#88021,#2708);
#2311=LINE('',#88059,#2709);
#2312=LINE('',#88599,#2710);
#2313=LINE('',#89139,#2711);
#2314=LINE('',#89178,#2712);
#2315=LINE('',#91537,#2713);
#2316=LINE('',#91543,#2714);
#2685=VECTOR('',#10127,9.37025);
#2686=VECTOR('',#10132,9.37025);
#2687=VECTOR('',#10135,9.37025);
#2688=VECTOR('',#10138,9.37025);
#2689=VECTOR('',#10141,9.37025);
#2690=VECTOR('',#10144,9.37025);
#2691=VECTOR('',#10147,9.37025);
#2692=VECTOR('',#10150,9.37025);
#2693=VECTOR('',#10153,9.37025);
#2694=VECTOR('',#10156,9.37025);
#2695=VECTOR('',#10159,9.37025);
#2696=VECTOR('',#10162,9.37025);
#2697=VECTOR('',#10165,9.37025);
#2698=VECTOR('',#10168,9.37025);
#2699=VECTOR('',#10171,9.942);
#2700=VECTOR('',#10176,9.942);
#2701=VECTOR('',#10179,9.942);
#2702=VECTOR('',#10182,9.942);
#2703=VECTOR('',#10185,9.942);
#2704=VECTOR('',#10188,9.942);
#2705=VECTOR('',#10191,9.942);
#2706=VECTOR('',#10194,9.942);
#2707=VECTOR('',#10197,9.942);
#2708=VECTOR('',#10200,9.942);
#2709=VECTOR('',#10203,9.942);
#2710=VECTOR('',#10206,9.942);
#2711=VECTOR('',#10209,9.942);
#2712=VECTOR('',#10212,9.942);
#2713=VECTOR('',#10227,14.);
#2714=VECTOR('',#10234,5.);
#2824=CIRCLE('',#8847,9.37025);
#2825=CIRCLE('',#8862,9.942);
#2826=CIRCLE('',#8877,9.942);
#2827=CIRCLE('',#8879,9.37025);
#2828=CIRCLE('',#8881,14.);
#2829=CIRCLE('',#8883,14.);
#2830=CIRCLE('',#8885,5.);
#2831=CIRCLE('',#8886,5.);
#3682=VERTEX_POINT('',#79155);
#3683=VERTEX_POINT('',#79156);
#3684=VERTEX_POINT('',#79158);
#3685=VERTEX_POINT('',#79301);
#3686=VERTEX_POINT('',#79392);
#3687=VERTEX_POINT('',#79393);
#3688=VERTEX_POINT('',#79395);
#3689=VERTEX_POINT('',#79689);
#3690=VERTEX_POINT('',#79791);
#3691=VERTEX_POINT('',#79792);
#3692=VERTEX_POINT('',#80102);
#3693=VERTEX_POINT('',#80312);
#3694=VERTEX_POINT('',#80313);
#3695=VERTEX_POINT('',#80315);
#3696=VERTEX_POINT('',#80737);
#3697=VERTEX_POINT('',#80738);
#3698=VERTEX_POINT('',#80740);
#3699=VERTEX_POINT('',#80944);
#3700=VERTEX_POINT('',#81068);
#3701=VERTEX_POINT('',#81069);
#3702=VERTEX_POINT('',#81369);
#3703=VERTEX_POINT('',#81586);
#3704=VERTEX_POINT('',#81587);
#3705=VERTEX_POINT('',#81589);
#3706=VERTEX_POINT('',#81996);
#3707=VERTEX_POINT('',#81997);
#3708=VERTEX_POINT('',#81999);
#3709=VERTEX_POINT('',#82270);
#3710=VERTEX_POINT('',#82391);
#3711=VERTEX_POINT('',#82392);
#3712=VERTEX_POINT('',#82686);
#3713=VERTEX_POINT('',#82940);
#3714=VERTEX_POINT('',#82941);
#3715=VERTEX_POINT('',#82943);
#3716=VERTEX_POINT('',#83577);
#3717=VERTEX_POINT('',#83578);
#3718=VERTEX_POINT('',#83872);
#3719=VERTEX_POINT('',#84224);
#3720=VERTEX_POINT('',#84225);
#3721=VERTEX_POINT('',#84227);
#3722=VERTEX_POINT('',#84843);
#3723=VERTEX_POINT('',#84844);
#3724=VERTEX_POINT('',#85146);
#3725=VERTEX_POINT('',#85434);
#3726=VERTEX_POINT('',#85435);
#3727=VERTEX_POINT('',#85437);
#3728=VERTEX_POINT('',#85552);
#3729=VERTEX_POINT('',#85848);
#3730=VERTEX_POINT('',#85849);
#3731=VERTEX_POINT('',#85851);
#3732=VERTEX_POINT('',#85940);
#3733=VERTEX_POINT('',#85949);
#3734=VERTEX_POINT('',#85950);
#3735=VERTEX_POINT('',#86237);
#3736=VERTEX_POINT('',#86238);
#3737=VERTEX_POINT('',#86275);
#3738=VERTEX_POINT('',#86276);
#3739=VERTEX_POINT('',#86313);
#3740=VERTEX_POINT('',#86314);
#3741=VERTEX_POINT('',#86859);
#3742=VERTEX_POINT('',#86860);
#3743=VERTEX_POINT('',#86895);
#3744=VERTEX_POINT('',#86896);
#3745=VERTEX_POINT('',#86933);
#3746=VERTEX_POINT('',#86934);
#3747=VERTEX_POINT('',#87479);
#3748=VERTEX_POINT('',#87480);
#3749=VERTEX_POINT('',#88019);
#3750=VERTEX_POINT('',#88020);
#3751=VERTEX_POINT('',#88057);
#3752=VERTEX_POINT('',#88058);
#3753=VERTEX_POINT('',#88597);
#3754=VERTEX_POINT('',#88598);
#3755=VERTEX_POINT('',#89137);
#3756=VERTEX_POINT('',#89138);
#3757=VERTEX_POINT('',#89176);
#3758=VERTEX_POINT('',#89177);
#3759=VERTEX_POINT('',#89214);
#3760=VERTEX_POINT('',#89229);
#3761=VERTEX_POINT('',#89244);
#3762=VERTEX_POINT('',#89511);
#3763=VERTEX_POINT('',#89513);
#3764=VERTEX_POINT('',#91285);
#3765=VERTEX_POINT('',#91533);
#3766=VERTEX_POINT('',#91536);
#3767=VERTEX_POINT('',#91540);
#3768=VERTEX_POINT('',#91542);
#4913=EDGE_CURVE('',#3682,#3683,#2287,.T.);
#4914=EDGE_CURVE('',#3684,#3682,#820,.T.);
#4915=EDGE_CURVE('',#3685,#3684,#2824,.T.);
#4916=EDGE_CURVE('',#3685,#3683,#821,.T.);
#4917=EDGE_CURVE('',#3686,#3687,#2288,.T.);
#4918=EDGE_CURVE('',#3688,#3686,#822,.F.);
#4919=EDGE_CURVE('',#3682,#3688,#823,.T.);
#4920=EDGE_CURVE('',#3683,#3689,#824,.T.);
#4921=EDGE_CURVE('',#3689,#3687,#825,.T.);
#4922=EDGE_CURVE('',#3690,#3691,#2289,.T.);
#4923=EDGE_CURVE('',#3686,#3690,#826,.F.);
#4924=EDGE_CURVE('',#3687,#3692,#827,.T.);
#4925=EDGE_CURVE('',#3692,#3691,#828,.T.);
#4926=EDGE_CURVE('',#3693,#3694,#2290,.T.);
#4927=EDGE_CURVE('',#3695,#3693,#829,.T.);
#4928=EDGE_CURVE('',#3690,#3695,#830,.F.);
#4929=EDGE_CURVE('',#3691,#3694,#831,.T.);
#4930=EDGE_CURVE('',#3696,#3697,#2291,.T.);
#4931=EDGE_CURVE('',#3698,#3696,#832,.F.);
#4932=EDGE_CURVE('',#3693,#3698,#833,.T.);
#4933=EDGE_CURVE('',#3694,#3699,#834,.T.);
#4934=EDGE_CURVE('',#3699,#3697,#835,.T.);
#4935=EDGE_CURVE('',#3700,#3701,#2292,.T.);
#4936=EDGE_CURVE('',#3696,#3700,#836,.F.);
#4937=EDGE_CURVE('',#3697,#3702,#837,.T.);
#4938=EDGE_CURVE('',#3702,#3701,#838,.T.);
#4939=EDGE_CURVE('',#3703,#3704,#2293,.T.);
#4940=EDGE_CURVE('',#3705,#3703,#839,.T.);
#4941=EDGE_CURVE('',#3700,#3705,#840,.F.);
#4942=EDGE_CURVE('',#3701,#3704,#841,.T.);
#4943=EDGE_CURVE('',#3706,#3707,#2294,.T.);
#4944=EDGE_CURVE('',#3708,#3706,#842,.F.);
#4945=EDGE_CURVE('',#3703,#3708,#843,.T.);
#4946=EDGE_CURVE('',#3704,#3709,#844,.T.);
#4947=EDGE_CURVE('',#3709,#3707,#845,.T.);
#4948=EDGE_CURVE('',#3710,#3711,#2295,.T.);
#4949=EDGE_CURVE('',#3706,#3710,#846,.F.);
#4950=EDGE_CURVE('',#3707,#3712,#847,.T.);
#4951=EDGE_CURVE('',#3712,#3711,#848,.T.);
#4952=EDGE_CURVE('',#3713,#3714,#2296,.T.);
#4953=EDGE_CURVE('',#3715,#3713,#849,.F.);
#4954=EDGE_CURVE('',#3710,#3715,#850,.F.);
#4955=EDGE_CURVE('',#3711,#3714,#851,.T.);
#4956=EDGE_CURVE('',#3716,#3717,#2297,.T.);
#4957=EDGE_CURVE('',#3713,#3716,#852,.F.);
#4958=EDGE_CURVE('',#3714,#3718,#853,.T.);
#4959=EDGE_CURVE('',#3718,#3717,#854,.T.);
#4960=EDGE_CURVE('',#3719,#3720,#2298,.T.);
#4961=EDGE_CURVE('',#3721,#3719,#855,.F.);
#4962=EDGE_CURVE('',#3716,#3721,#856,.F.);
#4963=EDGE_CURVE('',#3717,#3720,#857,.T.);
#4964=EDGE_CURVE('',#3722,#3723,#2299,.T.);
#4965=EDGE_CURVE('',#3719,#3722,#858,.F.);
#4966=EDGE_CURVE('',#3720,#3724,#859,.T.);
#4967=EDGE_CURVE('',#3724,#3723,#860,.T.);
#4968=EDGE_CURVE('',#3725,#3726,#2300,.T.);
#4969=EDGE_CURVE('',#3727,#3725,#861,.T.);
#4970=EDGE_CURVE('',#3722,#3727,#862,.F.);
#4971=EDGE_CURVE('',#3723,#3728,#863,.T.);
#4972=EDGE_CURVE('',#3728,#3726,#864,.F.);
#4973=EDGE_CURVE('',#3729,#3730,#2301,.T.);
#4974=EDGE_CURVE('',#3729,#3731,#865,.T.);
#4975=EDGE_CURVE('',#3731,#3732,#2825,.F.);
#4976=EDGE_CURVE('',#3732,#3730,#866,.T.);
#4977=EDGE_CURVE('',#3733,#3734,#2302,.T.);
#4978=EDGE_CURVE('',#3733,#3729,#867,.T.);
#4979=EDGE_CURVE('',#3730,#3734,#868,.T.);
#4980=EDGE_CURVE('',#3735,#3736,#2303,.T.);
#4981=EDGE_CURVE('',#3735,#3733,#869,.T.);
#4982=EDGE_CURVE('',#3734,#3736,#870,.T.);
#4983=EDGE_CURVE('',#3737,#3738,#2304,.T.);
#4984=EDGE_CURVE('',#3737,#3735,#871,.T.);
#4985=EDGE_CURVE('',#3736,#3738,#872,.T.);
#4986=EDGE_CURVE('',#3739,#3740,#2305,.T.);
#4987=EDGE_CURVE('',#3739,#3737,#873,.T.);
#4988=EDGE_CURVE('',#3738,#3740,#874,.T.);
#4989=EDGE_CURVE('',#3741,#3742,#2306,.T.);
#4990=EDGE_CURVE('',#3741,#3739,#875,.T.);
#4991=EDGE_CURVE('',#3740,#3742,#876,.T.);
#4992=EDGE_CURVE('',#3743,#3744,#2307,.T.);
#4993=EDGE_CURVE('',#3743,#3741,#877,.T.);
#4994=EDGE_CURVE('',#3742,#3744,#878,.T.);
#4995=EDGE_CURVE('',#3745,#3746,#2308,.T.);
#4996=EDGE_CURVE('',#3745,#3743,#879,.T.);
#4997=EDGE_CURVE('',#3744,#3746,#880,.T.);
#4998=EDGE_CURVE('',#3747,#3748,#2309,.T.);
#4999=EDGE_CURVE('',#3747,#3745,#881,.T.);
#5000=EDGE_CURVE('',#3746,#3748,#882,.T.);
#5001=EDGE_CURVE('',#3749,#3750,#2310,.T.);
#5002=EDGE_CURVE('',#3749,#3747,#883,.T.);
#5003=EDGE_CURVE('',#3748,#3750,#884,.T.);
#5004=EDGE_CURVE('',#3751,#3752,#2311,.T.);
#5005=EDGE_CURVE('',#3751,#3749,#885,.T.);
#5006=EDGE_CURVE('',#3750,#3752,#886,.T.);
#5007=EDGE_CURVE('',#3753,#3754,#2312,.T.);
#5008=EDGE_CURVE('',#3753,#3751,#887,.T.);
#5009=EDGE_CURVE('',#3752,#3754,#888,.T.);
#5010=EDGE_CURVE('',#3755,#3756,#2313,.T.);
#5011=EDGE_CURVE('',#3755,#3753,#889,.T.);
#5012=EDGE_CURVE('',#3754,#3756,#890,.T.);
#5013=EDGE_CURVE('',#3757,#3758,#2314,.T.);
#5014=EDGE_CURVE('',#3757,#3755,#891,.T.);
#5015=EDGE_CURVE('',#3756,#3758,#892,.T.);
#5016=EDGE_CURVE('',#3758,#3759,#893,.T.);
#5017=EDGE_CURVE('',#3760,#3759,#2826,.F.);
#5018=EDGE_CURVE('',#3760,#3757,#894,.T.);
#5019=EDGE_CURVE('',#3726,#3761,#895,.F.);
#5020=EDGE_CURVE('',#3762,#3761,#2827,.T.);
#5021=EDGE_CURVE('',#3763,#3762,#896,.T.);
#5022=EDGE_CURVE('',#3725,#3763,#897,.T.);
#5023=EDGE_CURVE('',#3759,#3762,#898,.T.);
#5024=EDGE_CURVE('',#3684,#3732,#899,.T.);
#5025=EDGE_CURVE('',#3764,#3760,#900,.T.);
#5026=EDGE_CURVE('',#3761,#3764,#901,.T.);
#5027=EDGE_CURVE('',#3731,#3685,#902,.T.);
#5028=EDGE_CURVE('',#3765,#3765,#2828,.T.);
#5029=EDGE_CURVE('',#3765,#3766,#2315,.T.);
#5030=EDGE_CURVE('',#3766,#3766,#2829,.T.);
#5031=EDGE_CURVE('',#3767,#3767,#2830,.T.);
#5032=EDGE_CURVE('',#3767,#3768,#2316,.T.);
#5033=EDGE_CURVE('',#3768,#3768,#2831,.T.);
#7296=ORIENTED_EDGE('',*,*,#4913,.F.);
#7297=ORIENTED_EDGE('',*,*,#4914,.F.);
#7298=ORIENTED_EDGE('',*,*,#4915,.F.);
#7299=ORIENTED_EDGE('',*,*,#4916,.T.);
#7300=ORIENTED_EDGE('',*,*,#4917,.F.);
#7301=ORIENTED_EDGE('',*,*,#4918,.F.);
#7302=ORIENTED_EDGE('',*,*,#4919,.F.);
#7303=ORIENTED_EDGE('',*,*,#4913,.T.);
#7304=ORIENTED_EDGE('',*,*,#4920,.T.);
#7305=ORIENTED_EDGE('',*,*,#4921,.T.);
#7306=ORIENTED_EDGE('',*,*,#4922,.F.);
#7307=ORIENTED_EDGE('',*,*,#4923,.F.);
#7308=ORIENTED_EDGE('',*,*,#4917,.T.);
#7309=ORIENTED_EDGE('',*,*,#4924,.T.);
#7310=ORIENTED_EDGE('',*,*,#4925,.T.);
#7311=ORIENTED_EDGE('',*,*,#4926,.F.);
#7312=ORIENTED_EDGE('',*,*,#4927,.F.);
#7313=ORIENTED_EDGE('',*,*,#4928,.F.);
#7314=ORIENTED_EDGE('',*,*,#4922,.T.);
#7315=ORIENTED_EDGE('',*,*,#4929,.T.);
#7316=ORIENTED_EDGE('',*,*,#4930,.F.);
#7317=ORIENTED_EDGE('',*,*,#4931,.F.);
#7318=ORIENTED_EDGE('',*,*,#4932,.F.);
#7319=ORIENTED_EDGE('',*,*,#4926,.T.);
#7320=ORIENTED_EDGE('',*,*,#4933,.T.);
#7321=ORIENTED_EDGE('',*,*,#4934,.T.);
#7322=ORIENTED_EDGE('',*,*,#4935,.F.);
#7323=ORIENTED_EDGE('',*,*,#4936,.F.);
#7324=ORIENTED_EDGE('',*,*,#4930,.T.);
#7325=ORIENTED_EDGE('',*,*,#4937,.T.);
#7326=ORIENTED_EDGE('',*,*,#4938,.T.);
#7327=ORIENTED_EDGE('',*,*,#4939,.F.);
#7328=ORIENTED_EDGE('',*,*,#4940,.F.);
#7329=ORIENTED_EDGE('',*,*,#4941,.F.);
#7330=ORIENTED_EDGE('',*,*,#4935,.T.);
#7331=ORIENTED_EDGE('',*,*,#4942,.T.);
#7332=ORIENTED_EDGE('',*,*,#4943,.F.);
#7333=ORIENTED_EDGE('',*,*,#4944,.F.);
#7334=ORIENTED_EDGE('',*,*,#4945,.F.);
#7335=ORIENTED_EDGE('',*,*,#4939,.T.);
#7336=ORIENTED_EDGE('',*,*,#4946,.T.);
#7337=ORIENTED_EDGE('',*,*,#4947,.T.);
#7338=ORIENTED_EDGE('',*,*,#4948,.F.);
#7339=ORIENTED_EDGE('',*,*,#4949,.F.);
#7340=ORIENTED_EDGE('',*,*,#4943,.T.);
#7341=ORIENTED_EDGE('',*,*,#4950,.T.);
#7342=ORIENTED_EDGE('',*,*,#4951,.T.);
#7343=ORIENTED_EDGE('',*,*,#4952,.F.);
#7344=ORIENTED_EDGE('',*,*,#4953,.F.);
#7345=ORIENTED_EDGE('',*,*,#4954,.F.);
#7346=ORIENTED_EDGE('',*,*,#4948,.T.);
#7347=ORIENTED_EDGE('',*,*,#4955,.T.);
#7348=ORIENTED_EDGE('',*,*,#4956,.F.);
#7349=ORIENTED_EDGE('',*,*,#4957,.F.);
#7350=ORIENTED_EDGE('',*,*,#4952,.T.);
#7351=ORIENTED_EDGE('',*,*,#4958,.T.);
#7352=ORIENTED_EDGE('',*,*,#4959,.T.);
#7353=ORIENTED_EDGE('',*,*,#4960,.F.);
#7354=ORIENTED_EDGE('',*,*,#4961,.F.);
#7355=ORIENTED_EDGE('',*,*,#4962,.F.);
#7356=ORIENTED_EDGE('',*,*,#4956,.T.);
#7357=ORIENTED_EDGE('',*,*,#4963,.T.);
#7358=ORIENTED_EDGE('',*,*,#4964,.F.);
#7359=ORIENTED_EDGE('',*,*,#4965,.F.);
#7360=ORIENTED_EDGE('',*,*,#4960,.T.);
#7361=ORIENTED_EDGE('',*,*,#4966,.T.);
#7362=ORIENTED_EDGE('',*,*,#4967,.T.);
#7363=ORIENTED_EDGE('',*,*,#4968,.F.);
#7364=ORIENTED_EDGE('',*,*,#4969,.F.);
#7365=ORIENTED_EDGE('',*,*,#4970,.F.);
#7366=ORIENTED_EDGE('',*,*,#4964,.T.);
#7367=ORIENTED_EDGE('',*,*,#4971,.T.);
#7368=ORIENTED_EDGE('',*,*,#4972,.T.);
#7369=ORIENTED_EDGE('',*,*,#4973,.F.);
#7370=ORIENTED_EDGE('',*,*,#4974,.T.);
#7371=ORIENTED_EDGE('',*,*,#4975,.T.);
#7372=ORIENTED_EDGE('',*,*,#4976,.T.);
#7373=ORIENTED_EDGE('',*,*,#4977,.F.);
#7374=ORIENTED_EDGE('',*,*,#4978,.T.);
#7375=ORIENTED_EDGE('',*,*,#4973,.T.);
#7376=ORIENTED_EDGE('',*,*,#4979,.T.);
#7377=ORIENTED_EDGE('',*,*,#4980,.F.);
#7378=ORIENTED_EDGE('',*,*,#4981,.T.);
#7379=ORIENTED_EDGE('',*,*,#4977,.T.);
#7380=ORIENTED_EDGE('',*,*,#4982,.T.);
#7381=ORIENTED_EDGE('',*,*,#4983,.F.);
#7382=ORIENTED_EDGE('',*,*,#4984,.T.);
#7383=ORIENTED_EDGE('',*,*,#4980,.T.);
#7384=ORIENTED_EDGE('',*,*,#4985,.T.);
#7385=ORIENTED_EDGE('',*,*,#4986,.F.);
#7386=ORIENTED_EDGE('',*,*,#4987,.T.);
#7387=ORIENTED_EDGE('',*,*,#4983,.T.);
#7388=ORIENTED_EDGE('',*,*,#4988,.T.);
#7389=ORIENTED_EDGE('',*,*,#4989,.F.);
#7390=ORIENTED_EDGE('',*,*,#4990,.T.);
#7391=ORIENTED_EDGE('',*,*,#4986,.T.);
#7392=ORIENTED_EDGE('',*,*,#4991,.T.);
#7393=ORIENTED_EDGE('',*,*,#4992,.F.);
#7394=ORIENTED_EDGE('',*,*,#4993,.T.);
#7395=ORIENTED_EDGE('',*,*,#4989,.T.);
#7396=ORIENTED_EDGE('',*,*,#4994,.T.);
#7397=ORIENTED_EDGE('',*,*,#4995,.F.);
#7398=ORIENTED_EDGE('',*,*,#4996,.T.);
#7399=ORIENTED_EDGE('',*,*,#4992,.T.);
#7400=ORIENTED_EDGE('',*,*,#4997,.T.);
#7401=ORIENTED_EDGE('',*,*,#4998,.F.);
#7402=ORIENTED_EDGE('',*,*,#4999,.T.);
#7403=ORIENTED_EDGE('',*,*,#4995,.T.);
#7404=ORIENTED_EDGE('',*,*,#5000,.T.);
#7405=ORIENTED_EDGE('',*,*,#5001,.F.);
#7406=ORIENTED_EDGE('',*,*,#5002,.T.);
#7407=ORIENTED_EDGE('',*,*,#4998,.T.);
#7408=ORIENTED_EDGE('',*,*,#5003,.T.);
#7409=ORIENTED_EDGE('',*,*,#5004,.F.);
#7410=ORIENTED_EDGE('',*,*,#5005,.T.);
#7411=ORIENTED_EDGE('',*,*,#5001,.T.);
#7412=ORIENTED_EDGE('',*,*,#5006,.T.);
#7413=ORIENTED_EDGE('',*,*,#5007,.F.);
#7414=ORIENTED_EDGE('',*,*,#5008,.T.);
#7415=ORIENTED_EDGE('',*,*,#5004,.T.);
#7416=ORIENTED_EDGE('',*,*,#5009,.T.);
#7417=ORIENTED_EDGE('',*,*,#5010,.F.);
#7418=ORIENTED_EDGE('',*,*,#5011,.T.);
#7419=ORIENTED_EDGE('',*,*,#5007,.T.);
#7420=ORIENTED_EDGE('',*,*,#5012,.T.);
#7421=ORIENTED_EDGE('',*,*,#5013,.F.);
#7422=ORIENTED_EDGE('',*,*,#5014,.T.);
#7423=ORIENTED_EDGE('',*,*,#5010,.T.);
#7424=ORIENTED_EDGE('',*,*,#5015,.T.);
#7425=ORIENTED_EDGE('',*,*,#5013,.T.);
#7426=ORIENTED_EDGE('',*,*,#5016,.T.);
#7427=ORIENTED_EDGE('',*,*,#5017,.F.);
#7428=ORIENTED_EDGE('',*,*,#5018,.T.);
#7429=ORIENTED_EDGE('',*,*,#4968,.T.);
#7430=ORIENTED_EDGE('',*,*,#5019,.T.);
#7431=ORIENTED_EDGE('',*,*,#5020,.F.);
#7432=ORIENTED_EDGE('',*,*,#5021,.F.);
#7433=ORIENTED_EDGE('',*,*,#5022,.F.);
#7434=ORIENTED_EDGE('',*,*,#5023,.F.);
#7435=ORIENTED_EDGE('',*,*,#5016,.F.);
#7436=ORIENTED_EDGE('',*,*,#5015,.F.);
#7437=ORIENTED_EDGE('',*,*,#5012,.F.);
#7438=ORIENTED_EDGE('',*,*,#5009,.F.);
#7439=ORIENTED_EDGE('',*,*,#5006,.F.);
#7440=ORIENTED_EDGE('',*,*,#5003,.F.);
#7441=ORIENTED_EDGE('',*,*,#5000,.F.);
#7442=ORIENTED_EDGE('',*,*,#4997,.F.);
#7443=ORIENTED_EDGE('',*,*,#4994,.F.);
#7444=ORIENTED_EDGE('',*,*,#4991,.F.);
#7445=ORIENTED_EDGE('',*,*,#4988,.F.);
#7446=ORIENTED_EDGE('',*,*,#4985,.F.);
#7447=ORIENTED_EDGE('',*,*,#4982,.F.);
#7448=ORIENTED_EDGE('',*,*,#4979,.F.);
#7449=ORIENTED_EDGE('',*,*,#4976,.F.);
#7450=ORIENTED_EDGE('',*,*,#5024,.F.);
#7451=ORIENTED_EDGE('',*,*,#4914,.T.);
#7452=ORIENTED_EDGE('',*,*,#4919,.T.);
#7453=ORIENTED_EDGE('',*,*,#4918,.T.);
#7454=ORIENTED_EDGE('',*,*,#4923,.T.);
#7455=ORIENTED_EDGE('',*,*,#4928,.T.);
#7456=ORIENTED_EDGE('',*,*,#4927,.T.);
#7457=ORIENTED_EDGE('',*,*,#4932,.T.);
#7458=ORIENTED_EDGE('',*,*,#4931,.T.);
#7459=ORIENTED_EDGE('',*,*,#4936,.T.);
#7460=ORIENTED_EDGE('',*,*,#4941,.T.);
#7461=ORIENTED_EDGE('',*,*,#4940,.T.);
#7462=ORIENTED_EDGE('',*,*,#4945,.T.);
#7463=ORIENTED_EDGE('',*,*,#4944,.T.);
#7464=ORIENTED_EDGE('',*,*,#4949,.T.);
#7465=ORIENTED_EDGE('',*,*,#4954,.T.);
#7466=ORIENTED_EDGE('',*,*,#4953,.T.);
#7467=ORIENTED_EDGE('',*,*,#4957,.T.);
#7468=ORIENTED_EDGE('',*,*,#4962,.T.);
#7469=ORIENTED_EDGE('',*,*,#4961,.T.);
#7470=ORIENTED_EDGE('',*,*,#4965,.T.);
#7471=ORIENTED_EDGE('',*,*,#4970,.T.);
#7472=ORIENTED_EDGE('',*,*,#4969,.T.);
#7473=ORIENTED_EDGE('',*,*,#5022,.T.);
#7474=ORIENTED_EDGE('',*,*,#5021,.T.);
#7475=ORIENTED_EDGE('',*,*,#5025,.F.);
#7476=ORIENTED_EDGE('',*,*,#5026,.F.);
#7477=ORIENTED_EDGE('',*,*,#5019,.F.);
#7478=ORIENTED_EDGE('',*,*,#4972,.F.);
#7479=ORIENTED_EDGE('',*,*,#4971,.F.);
#7480=ORIENTED_EDGE('',*,*,#4967,.F.);
#7481=ORIENTED_EDGE('',*,*,#4966,.F.);
#7482=ORIENTED_EDGE('',*,*,#4963,.F.);
#7483=ORIENTED_EDGE('',*,*,#4959,.F.);
#7484=ORIENTED_EDGE('',*,*,#4958,.F.);
#7485=ORIENTED_EDGE('',*,*,#4955,.F.);
#7486=ORIENTED_EDGE('',*,*,#4951,.F.);
#7487=ORIENTED_EDGE('',*,*,#4950,.F.);
#7488=ORIENTED_EDGE('',*,*,#4947,.F.);
#7489=ORIENTED_EDGE('',*,*,#4946,.F.);
#7490=ORIENTED_EDGE('',*,*,#4942,.F.);
#7491=ORIENTED_EDGE('',*,*,#4938,.F.);
#7492=ORIENTED_EDGE('',*,*,#4937,.F.);
#7493=ORIENTED_EDGE('',*,*,#4934,.F.);
#7494=ORIENTED_EDGE('',*,*,#4933,.F.);
#7495=ORIENTED_EDGE('',*,*,#4929,.F.);
#7496=ORIENTED_EDGE('',*,*,#4925,.F.);
#7497=ORIENTED_EDGE('',*,*,#4924,.F.);
#7498=ORIENTED_EDGE('',*,*,#4921,.F.);
#7499=ORIENTED_EDGE('',*,*,#4920,.F.);
#7500=ORIENTED_EDGE('',*,*,#4916,.F.);
#7501=ORIENTED_EDGE('',*,*,#5027,.F.);
#7502=ORIENTED_EDGE('',*,*,#4974,.F.);
#7503=ORIENTED_EDGE('',*,*,#4978,.F.);
#7504=ORIENTED_EDGE('',*,*,#4981,.F.);
#7505=ORIENTED_EDGE('',*,*,#4984,.F.);
#7506=ORIENTED_EDGE('',*,*,#4987,.F.);
#7507=ORIENTED_EDGE('',*,*,#4990,.F.);
#7508=ORIENTED_EDGE('',*,*,#4993,.F.);
#7509=ORIENTED_EDGE('',*,*,#4996,.F.);
#7510=ORIENTED_EDGE('',*,*,#4999,.F.);
#7511=ORIENTED_EDGE('',*,*,#5002,.F.);
#7512=ORIENTED_EDGE('',*,*,#5005,.F.);
#7513=ORIENTED_EDGE('',*,*,#5008,.F.);
#7514=ORIENTED_EDGE('',*,*,#5011,.F.);
#7515=ORIENTED_EDGE('',*,*,#5014,.F.);
#7516=ORIENTED_EDGE('',*,*,#5018,.F.);
#7517=ORIENTED_EDGE('',*,*,#5028,.T.);
#7518=ORIENTED_EDGE('',*,*,#5027,.T.);
#7519=ORIENTED_EDGE('',*,*,#4915,.T.);
#7520=ORIENTED_EDGE('',*,*,#5024,.T.);
#7521=ORIENTED_EDGE('',*,*,#4975,.F.);
#7522=ORIENTED_EDGE('',*,*,#5028,.F.);
#7523=ORIENTED_EDGE('',*,*,#5029,.T.);
#7524=ORIENTED_EDGE('',*,*,#5030,.T.);
#7525=ORIENTED_EDGE('',*,*,#5029,.F.);
#7526=ORIENTED_EDGE('',*,*,#5031,.T.);
#7527=ORIENTED_EDGE('',*,*,#5032,.T.);
#7528=ORIENTED_EDGE('',*,*,#5033,.F.);
#7529=ORIENTED_EDGE('',*,*,#5032,.F.);
#7530=ORIENTED_EDGE('',*,*,#5025,.T.);
#7531=ORIENTED_EDGE('',*,*,#5017,.T.);
#7532=ORIENTED_EDGE('',*,*,#5023,.T.);
#7533=ORIENTED_EDGE('',*,*,#5020,.T.);
#7534=ORIENTED_EDGE('',*,*,#5026,.T.);
#7535=ORIENTED_EDGE('',*,*,#5033,.T.);
#7536=ORIENTED_EDGE('',*,*,#5030,.F.);
#7537=ORIENTED_EDGE('',*,*,#5031,.F.);
#7848=CYLINDRICAL_SURFACE('',#8846,9.37025);
#7849=CYLINDRICAL_SURFACE('',#8848,9.37025);
#7850=CYLINDRICAL_SURFACE('',#8849,9.37025);
#7851=CYLINDRICAL_SURFACE('',#8850,9.37025);
#7852=CYLINDRICAL_SURFACE('',#8851,9.37025);
#7853=CYLINDRICAL_SURFACE('',#8852,9.37025);
#7854=CYLINDRICAL_SURFACE('',#8853,9.37025);
#7855=CYLINDRICAL_SURFACE('',#8854,9.37025);
#7856=CYLINDRICAL_SURFACE('',#8855,9.37025);
#7857=CYLINDRICAL_SURFACE('',#8856,9.37025);
#7858=CYLINDRICAL_SURFACE('',#8857,9.37025);
#7859=CYLINDRICAL_SURFACE('',#8858,9.37025);
#7860=CYLINDRICAL_SURFACE('',#8859,9.37025);
#7861=CYLINDRICAL_SURFACE('',#8860,9.37025);
#7862=CYLINDRICAL_SURFACE('',#8861,9.942);
#7863=CYLINDRICAL_SURFACE('',#8863,9.942);
#7864=CYLINDRICAL_SURFACE('',#8864,9.942);
#7865=CYLINDRICAL_SURFACE('',#8865,9.942);
#7866=CYLINDRICAL_SURFACE('',#8866,9.942);
#7867=CYLINDRICAL_SURFACE('',#8867,9.942);
#7868=CYLINDRICAL_SURFACE('',#8868,9.942);
#7869=CYLINDRICAL_SURFACE('',#8869,9.942);
#7870=CYLINDRICAL_SURFACE('',#8870,9.942);
#7871=CYLINDRICAL_SURFACE('',#8871,9.942);
#7872=CYLINDRICAL_SURFACE('',#8872,9.942);
#7873=CYLINDRICAL_SURFACE('',#8873,9.942);
#7874=CYLINDRICAL_SURFACE('',#8874,9.942);
#7875=CYLINDRICAL_SURFACE('',#8875,9.942);
#7876=CYLINDRICAL_SURFACE('',#8876,9.942);
#7877=CYLINDRICAL_SURFACE('',#8878,9.37025);
#7878=CYLINDRICAL_SURFACE('',#8882,14.);
#7879=CYLINDRICAL_SURFACE('',#8884,5.);
#8193=ADVANCED_FACE('',(#1456),#7848,.T.);
#8194=ADVANCED_FACE('',(#1457),#7849,.T.);
#8195=ADVANCED_FACE('',(#1458),#7850,.T.);
#8196=ADVANCED_FACE('',(#1459),#7851,.T.);
#8197=ADVANCED_FACE('',(#1460),#7852,.T.);
#8198=ADVANCED_FACE('',(#1461),#7853,.T.);
#8199=ADVANCED_FACE('',(#1462),#7854,.T.);
#8200=ADVANCED_FACE('',(#1463),#7855,.T.);
#8201=ADVANCED_FACE('',(#1464),#7856,.T.);
#8202=ADVANCED_FACE('',(#1465),#7857,.T.);
#8203=ADVANCED_FACE('',(#1466),#7858,.T.);
#8204=ADVANCED_FACE('',(#1467),#7859,.T.);
#8205=ADVANCED_FACE('',(#1468),#7860,.T.);
#8206=ADVANCED_FACE('',(#1469),#7861,.T.);
#8207=ADVANCED_FACE('',(#1470),#7862,.T.);
#8208=ADVANCED_FACE('',(#1471),#7863,.T.);
#8209=ADVANCED_FACE('',(#1472),#7864,.T.);
#8210=ADVANCED_FACE('',(#1473),#7865,.T.);
#8211=ADVANCED_FACE('',(#1474),#7866,.T.);
#8212=ADVANCED_FACE('',(#1475),#7867,.T.);
#8213=ADVANCED_FACE('',(#1476),#7868,.T.);
#8214=ADVANCED_FACE('',(#1477),#7869,.T.);
#8215=ADVANCED_FACE('',(#1478),#7870,.T.);
#8216=ADVANCED_FACE('',(#1479),#7871,.T.);
#8217=ADVANCED_FACE('',(#1480),#7872,.T.);
#8218=ADVANCED_FACE('',(#1481),#7873,.T.);
#8219=ADVANCED_FACE('',(#1482),#7874,.T.);
#8220=ADVANCED_FACE('',(#1483),#7875,.T.);
#8221=ADVANCED_FACE('',(#1484),#7876,.T.);
#8222=ADVANCED_FACE('',(#1485),#7877,.T.);
#8223=ADVANCED_FACE('',(#1486),#166,.F.);
#8224=ADVANCED_FACE('',(#1487),#167,.F.);
#8225=ADVANCED_FACE('',(#1488,#1047),#1151,.T.);
#8226=ADVANCED_FACE('',(#1489),#7878,.T.);
#8227=ADVANCED_FACE('',(#1490),#7879,.F.);
#8228=ADVANCED_FACE('',(#1491,#1048),#1152,.T.);
#8229=ADVANCED_FACE('',(#1492,#1049),#1153,.F.);
#8263=CLOSED_SHELL('',(#8193,#8194,#8195,#8196,#8197,#8198,#8199,#8200,
#8201,#8202,#8203,#8204,#8205,#8206,#8207,#8208,#8209,#8210,#8211,#8212,
#8213,#8214,#8215,#8216,#8217,#8218,#8219,#8220,#8221,#8222,#8223,#8224,
#8225,#8226,#8227,#8228,#8229));
#8845=AXIS2_PLACEMENT_3D('',#79153,#10123,#10124);
#8846=AXIS2_PLACEMENT_3D('',#79154,#10125,#10126);
#8847=AXIS2_PLACEMENT_3D('',#79302,#10128,#10129);
#8848=AXIS2_PLACEMENT_3D('',#79391,#10130,#10131);
#8849=AXIS2_PLACEMENT_3D('',#79790,#10133,#10134);
#8850=AXIS2_PLACEMENT_3D('',#80311,#10136,#10137);
#8851=AXIS2_PLACEMENT_3D('',#80736,#10139,#10140);
#8852=AXIS2_PLACEMENT_3D('',#81067,#10142,#10143);
#8853=AXIS2_PLACEMENT_3D('',#81585,#10145,#10146);
#8854=AXIS2_PLACEMENT_3D('',#81995,#10148,#10149);
#8855=AXIS2_PLACEMENT_3D('',#82390,#10151,#10152);
#8856=AXIS2_PLACEMENT_3D('',#82939,#10154,#10155);
#8857=AXIS2_PLACEMENT_3D('',#83576,#10157,#10158);
#8858=AXIS2_PLACEMENT_3D('',#84223,#10160,#10161);
#8859=AXIS2_PLACEMENT_3D('',#84842,#10163,#10164);
#8860=AXIS2_PLACEMENT_3D('',#85433,#10166,#10167);
#8861=AXIS2_PLACEMENT_3D('',#85847,#10169,#10170);
#8862=AXIS2_PLACEMENT_3D('',#85941,#10172,#10173);
#8863=AXIS2_PLACEMENT_3D('',#85948,#10174,#10175);
#8864=AXIS2_PLACEMENT_3D('',#86236,#10177,#10178);
#8865=AXIS2_PLACEMENT_3D('',#86274,#10180,#10181);
#8866=AXIS2_PLACEMENT_3D('',#86312,#10183,#10184);
#8867=AXIS2_PLACEMENT_3D('',#86858,#10186,#10187);
#8868=AXIS2_PLACEMENT_3D('',#86894,#10189,#10190);
#8869=AXIS2_PLACEMENT_3D('',#86932,#10192,#10193);
#8870=AXIS2_PLACEMENT_3D('',#87478,#10195,#10196);
#8871=AXIS2_PLACEMENT_3D('',#88018,#10198,#10199);
#8872=AXIS2_PLACEMENT_3D('',#88056,#10201,#10202);
#8873=AXIS2_PLACEMENT_3D('',#88596,#10204,#10205);
#8874=AXIS2_PLACEMENT_3D('',#89136,#10207,#10208);
#8875=AXIS2_PLACEMENT_3D('',#89175,#10210,#10211);
#8876=AXIS2_PLACEMENT_3D('',#89213,#10213,#10214);
#8877=AXIS2_PLACEMENT_3D('',#89230,#10215,#10216);
#8878=AXIS2_PLACEMENT_3D('',#89243,#10217,#10218);
#8879=AXIS2_PLACEMENT_3D('',#89512,#10219,#10220);
#8880=AXIS2_PLACEMENT_3D('',#91532,#10221,#10222);
#8881=AXIS2_PLACEMENT_3D('',#91534,#10223,#10224);
#8882=AXIS2_PLACEMENT_3D('',#91535,#10225,#10226);
#8883=AXIS2_PLACEMENT_3D('',#91538,#10228,#10229);
#8884=AXIS2_PLACEMENT_3D('',#91539,#10230,#10231);
#8885=AXIS2_PLACEMENT_3D('',#91541,#10232,#10233);
#8886=AXIS2_PLACEMENT_3D('',#91544,#10235,#10236);
#8887=AXIS2_PLACEMENT_3D('',#91545,#10237,#10238);
#8888=AXIS2_PLACEMENT_3D('',#91546,#10239,#10240);
#10123=DIRECTION('axis',(0.,0.,1.));
#10124=DIRECTION('refdir',(1.,0.,0.));
#10125=DIRECTION('center_axis',(0.,0.,1.));
#10126=DIRECTION('ref_axis',(-0.457930858638424,-0.888987811337521,0.));
#10127=DIRECTION('',(0.,0.,-1.));
#10128=DIRECTION('center_axis',(0.,0.,-1.));
#10129=DIRECTION('ref_axis',(1.,7.94191995926203E-14,0.));
#10130=DIRECTION('center_axis',(0.,0.,1.));
#10131=DIRECTION('ref_axis',(-0.457930858638424,-0.888987811337521,0.));
#10132=DIRECTION('',(0.,0.,-1.));
#10133=DIRECTION('center_axis',(0.,0.,1.));
#10134=DIRECTION('ref_axis',(-0.457930858638424,-0.888987811337521,0.));
#10135=DIRECTION('',(0.,0.,-1.));
#10136=DIRECTION('center_axis',(0.,0.,1.));
#10137=DIRECTION('ref_axis',(-0.457930858638424,-0.888987811337521,0.));
#10138=DIRECTION('',(0.,0.,-1.));
#10139=DIRECTION('center_axis',(0.,0.,1.));
#10140=DIRECTION('ref_axis',(-0.457930858638424,-0.888987811337521,0.));
#10141=DIRECTION('',(0.,0.,-1.));
#10142=DIRECTION('center_axis',(0.,0.,1.));
#10143=DIRECTION('ref_axis',(-0.457930858638424,-0.888987811337521,0.));
#10144=DIRECTION('',(0.,0.,-1.));
#10145=DIRECTION('center_axis',(0.,0.,1.));
#10146=DIRECTION('ref_axis',(-0.457930858638424,-0.888987811337521,0.));
#10147=DIRECTION('',(0.,0.,-1.));
#10148=DIRECTION('center_axis',(0.,0.,1.));
#10149=DIRECTION('ref_axis',(-0.457930858638424,-0.888987811337521,0.));
#10150=DIRECTION('',(0.,0.,-1.));
#10151=DIRECTION('center_axis',(0.,0.,1.));
#10152=DIRECTION('ref_axis',(-0.457930858638424,-0.888987811337521,0.));
#10153=DIRECTION('',(0.,0.,-1.));
#10154=DIRECTION('center_axis',(0.,0.,1.));
#10155=DIRECTION('ref_axis',(-0.457930858638424,-0.888987811337521,0.));
#10156=DIRECTION('',(0.,0.,-1.));
#10157=DIRECTION('center_axis',(0.,0.,1.));
#10158=DIRECTION('ref_axis',(-0.457930858638424,-0.888987811337521,0.));
#10159=DIRECTION('',(0.,0.,-1.));
#10160=DIRECTION('center_axis',(0.,0.,1.));
#10161=DIRECTION('ref_axis',(-0.457930858638424,-0.888987811337521,0.));
#10162=DIRECTION('',(0.,0.,-1.));
#10163=DIRECTION('center_axis',(0.,0.,1.));
#10164=DIRECTION('ref_axis',(-0.457930858638424,-0.888987811337521,0.));
#10165=DIRECTION('',(0.,0.,-1.));
#10166=DIRECTION('center_axis',(0.,0.,1.));
#10167=DIRECTION('ref_axis',(-0.457930858638424,-0.888987811337521,0.));
#10168=DIRECTION('',(0.,0.,-1.));
#10169=DIRECTION('center_axis',(0.,0.,1.));
#10170=DIRECTION('ref_axis',(1.,0.,0.));
#10171=DIRECTION('',(0.,0.,-1.));
#10172=DIRECTION('center_axis',(0.,0.,-1.));
#10173=DIRECTION('ref_axis',(1.,0.,0.));
#10174=DIRECTION('center_axis',(0.,0.,1.));
#10175=DIRECTION('ref_axis',(1.,0.,0.));
#10176=DIRECTION('',(0.,0.,-1.));
#10177=DIRECTION('center_axis',(0.,0.,1.));
#10178=DIRECTION('ref_axis',(1.,0.,0.));
#10179=DIRECTION('',(0.,0.,-1.));
#10180=DIRECTION('center_axis',(0.,0.,1.));
#10181=DIRECTION('ref_axis',(1.,0.,0.));
#10182=DIRECTION('',(0.,0.,-1.));
#10183=DIRECTION('center_axis',(0.,0.,1.));
#10184=DIRECTION('ref_axis',(1.,0.,0.));
#10185=DIRECTION('',(0.,0.,-1.));
#10186=DIRECTION('center_axis',(0.,0.,1.));
#10187=DIRECTION('ref_axis',(1.,0.,0.));
#10188=DIRECTION('',(0.,0.,-1.));
#10189=DIRECTION('center_axis',(0.,0.,1.));
#10190=DIRECTION('ref_axis',(1.,0.,0.));
#10191=DIRECTION('',(0.,0.,-1.));
#10192=DIRECTION('center_axis',(0.,0.,1.));
#10193=DIRECTION('ref_axis',(1.,0.,0.));
#10194=DIRECTION('',(0.,0.,-1.));
#10195=DIRECTION('center_axis',(0.,0.,1.));
#10196=DIRECTION('ref_axis',(1.,0.,0.));
#10197=DIRECTION('',(0.,0.,-1.));
#10198=DIRECTION('center_axis',(0.,0.,1.));
#10199=DIRECTION('ref_axis',(1.,0.,0.));
#10200=DIRECTION('',(0.,0.,-1.));
#10201=DIRECTION('center_axis',(0.,0.,1.));
#10202=DIRECTION('ref_axis',(1.,0.,0.));
#10203=DIRECTION('',(0.,0.,-1.));
#10204=DIRECTION('center_axis',(0.,0.,1.));
#10205=DIRECTION('ref_axis',(1.,0.,0.));
#10206=DIRECTION('',(0.,0.,-1.));
#10207=DIRECTION('center_axis',(0.,0.,1.));
#10208=DIRECTION('ref_axis',(1.,0.,0.));
#10209=DIRECTION('',(0.,0.,-1.));
#10210=DIRECTION('center_axis',(0.,0.,1.));
#10211=DIRECTION('ref_axis',(1.,0.,0.));
#10212=DIRECTION('',(0.,0.,-1.));
#10213=DIRECTION('center_axis',(0.,0.,1.));
#10214=DIRECTION('ref_axis',(1.,0.,0.));
#10215=DIRECTION('center_axis',(0.,0.,-1.));
#10216=DIRECTION('ref_axis',(1.,0.,0.));
#10217=DIRECTION('center_axis',(0.,0.,1.));
#10218=DIRECTION('ref_axis',(-0.457930858638424,-0.888987811337521,0.));
#10219=DIRECTION('center_axis',(0.,0.,1.));
#10220=DIRECTION('ref_axis',(1.,7.94191995926203E-14,0.));
#10221=DIRECTION('center_axis',(0.,0.,1.));
#10222=DIRECTION('ref_axis',(1.,0.,0.));
#10223=DIRECTION('center_axis',(0.,0.,1.));
#10224=DIRECTION('ref_axis',(1.,0.,0.));
#10225=DIRECTION('center_axis',(0.,0.,1.));
#10226=DIRECTION('ref_axis',(1.,0.,0.));
#10227=DIRECTION('',(0.,0.,-1.));
#10228=DIRECTION('center_axis',(0.,0.,1.));
#10229=DIRECTION('ref_axis',(1.,0.,0.));
#10230=DIRECTION('center_axis',(0.,0.,1.));
#10231=DIRECTION('ref_axis',(1.,0.,0.));
#10232=DIRECTION('center_axis',(0.,0.,-1.));
#10233=DIRECTION('ref_axis',(1.,0.,0.));
#10234=DIRECTION('',(0.,0.,1.));
#10235=DIRECTION('center_axis',(0.,0.,-1.));
#10236=DIRECTION('ref_axis',(1.,0.,0.));
#10237=DIRECTION('center_axis',(0.,0.,1.));
#10238=DIRECTION('ref_axis',(1.,0.,0.));
#10239=DIRECTION('center_axis',(0.,0.,1.));
#10240=DIRECTION('ref_axis',(1.,0.,0.));
#79153=CARTESIAN_POINT('',(0.,0.,0.));
#79154=CARTESIAN_POINT('Origin',(0.,0.,2.15141010809499));
#79155=CARTESIAN_POINT('',(4.2909266281567,8.33003803918541,4.52288275511062));
#79156=CARTESIAN_POINT('',(4.29092662815669,8.33003803918541,4.32570756359748));
#79157=CARTESIAN_POINT('',(4.29092662815669,8.33003803918541,2.15141010809499));
#79158=CARTESIAN_POINT('',(-5.44048627969075,-7.62906901941493,4.00000000616494));
#79159=CARTESIAN_POINT('Ctrl Pts',(-5.44048627969075,-7.62906901941493,
4.00000000616494));
#79160=CARTESIAN_POINT('Ctrl Pts',(-5.25102146993863,-7.76418127168548,
4.00395293893828));
#79161=CARTESIAN_POINT('Ctrl Pts',(-5.05649608080199,-7.89224980204389,
4.00790587171162));
#79162=CARTESIAN_POINT('Ctrl Pts',(-4.85745790948893,-8.01290756966805,
4.01185880448497));
#79163=CARTESIAN_POINT('Ctrl Pts',(-4.65844439494387,-8.13355039025684,
4.0158112475706));
#79164=CARTESIAN_POINT('Ctrl Pts',(-4.45491946109027,-8.24678413124755,
4.01976369065623));
#79165=CARTESIAN_POINT('Ctrl Pts',(-4.24745820141938,-8.3522861474985,4.02371613374186));
#79166=CARTESIAN_POINT('Ctrl Pts',(-4.03998379596611,-8.45779484888453,
4.02766882727405));
#79167=CARTESIAN_POINT('Ctrl Pts',(-3.82857282246667,-8.55557071332864,
4.03162152080623));
#79168=CARTESIAN_POINT('Ctrl Pts',(-3.61382422694981,-8.645337443918,4.03557421433841));
#79169=CARTESIAN_POINT('Ctrl Pts',(-3.39907558674732,-8.73510419318633,
4.03952690869308));
#79170=CARTESIAN_POINT('Ctrl Pts',(-3.18098959057493,-8.81686169639834,
4.04347960304776));
#79171=CARTESIAN_POINT('Ctrl Pts',(-2.96018499421697,-8.89038187382931,
4.04743229740243));
#79172=CARTESIAN_POINT('Ctrl Pts',(-2.73933409392948,-8.96391746884293,
4.05138582065869));
#79173=CARTESIAN_POINT('Ctrl Pts',(-2.51576372857753,-9.02921219607435,
4.05533934391495));
#79174=CARTESIAN_POINT('Ctrl Pts',(-2.29010878757626,-9.08608754104681,
4.05929286717121));
#79175=CARTESIAN_POINT('Ctrl Pts',(-2.20846628460654,-9.10666517830223,
4.06072326143937));
#79176=CARTESIAN_POINT('Ctrl Pts',(-2.12655103750013,-9.12614118745565,
4.06215365570753));
#79177=CARTESIAN_POINT('Ctrl Pts',(-2.04439351365759,-9.14450874699209,
4.06358404997569));
#79178=CARTESIAN_POINT('Ctrl Pts',(-1.8164772133919,-9.19546288994408,4.06755216092004));
#79179=CARTESIAN_POINT('Ctrl Pts',(-1.58661959870168,-9.23789988448231,
4.07152027186439));
#79180=CARTESIAN_POINT('Ctrl Pts',(-1.35547239192246,-9.27169238366093,
4.07548838280874));
#79181=CARTESIAN_POINT('Ctrl Pts',(-1.12436567230507,-9.3054789638306,4.07945579870879));
#79182=CARTESIAN_POINT('Ctrl Pts',(-0.891970092874594,-9.33062402994177,
4.08342321460883));
#79183=CARTESIAN_POINT('Ctrl Pts',(-0.65894540976201,-9.34705172818968,
4.08739063050888));
#79184=CARTESIAN_POINT('Ctrl Pts',(-0.425946105705265,-9.36347763727317,
4.09135761431191));
#79185=CARTESIAN_POINT('Ctrl Pts',(-0.192318118472125,-9.37118805412488,
4.09532459811494));
#79186=CARTESIAN_POINT('Ctrl Pts',(0.0412748677381543,-9.37015909404922,
4.09929158191797));
#79187=CARTESIAN_POINT('Ctrl Pts',(0.274886125731263,-9.36913005348768,
4.10325887602084));
#79188=CARTESIAN_POINT('Ctrl Pts',(0.508462092689314,-9.35936026837331,
4.10722617012371));
#79189=CARTESIAN_POINT('Ctrl Pts',(0.741339046271913,-9.34087798234046,
4.11119346422658));
#79190=CARTESIAN_POINT('Ctrl Pts',(0.974213587877025,-9.32239588773426,
4.11516071723898));
#79191=CARTESIAN_POINT('Ctrl Pts',(1.20638884712689,-9.2952014974446,4.11912797025138));
#79192=CARTESIAN_POINT('Ctrl Pts',(1.43720550210129,-9.25937500089665,4.12309522326378));
#79193=CARTESIAN_POINT('Ctrl Pts',(1.66807196794911,-9.22354077289151,4.12706333242037));
#79194=CARTESIAN_POINT('Ctrl Pts',(1.89757896236427,-9.17907075958204,4.13103144157696));
#79195=CARTESIAN_POINT('Ctrl Pts',(2.12507535254614,-9.12609663593921,4.13499955073354));
#79196=CARTESIAN_POINT('Ctrl Pts',(2.26498852057068,-9.09351687739329,4.13743998823992));
#79197=CARTESIAN_POINT('Ctrl Pts',(2.40414138272164,-9.05772152559798,4.1398804257463));
#79198=CARTESIAN_POINT('Ctrl Pts',(2.54238478313434,-9.01875072706786,4.14232086325268));
#79199=CARTESIAN_POINT('Ctrl Pts',(2.7671614585895,-8.95538620834737,4.14628888941307));
#79200=CARTESIAN_POINT('Ctrl Pts',(2.98960313356232,-8.88360437568409,4.15025691557347));
#79201=CARTESIAN_POINT('Ctrl Pts',(3.20907578261301,-8.80360254009384,4.15422494173386));
#79202=CARTESIAN_POINT('Ctrl Pts',(3.42850982836864,-8.72361477611788,4.1581922699536));
#79203=CARTESIAN_POINT('Ctrl Pts',(3.64497562342645,-8.63540999266812,4.16215959817334));
#79204=CARTESIAN_POINT('Ctrl Pts',(3.85785651725796,-8.53923463518542,4.16612692639308));
#79205=CARTESIAN_POINT('Ctrl Pts',(4.07071408462154,-8.4430698161374,4.17009381989201));
#79206=CARTESIAN_POINT('Ctrl Pts',(4.27998727585202,-8.33893628395689,4.17406071339094));
#79207=CARTESIAN_POINT('Ctrl Pts',(4.48508065509893,-8.22712808820657,4.17802760688987));
#79208=CARTESIAN_POINT('Ctrl Pts',(4.69018990518877,-8.11531124034704,4.18199480736089));
#79209=CARTESIAN_POINT('Ctrl Pts',(4.89111844574226,-7.99581867584552,4.18596200783191));
#79210=CARTESIAN_POINT('Ctrl Pts',(5.0872955554571,-7.86899034145591,4.18992920830294));
#79211=CARTESIAN_POINT('Ctrl Pts',(5.28347054755643,-7.74216337610293,4.19389636595038));
#79212=CARTESIAN_POINT('Ctrl Pts',(5.47489397364357,-7.60800095560125,4.19786352359783));
#79213=CARTESIAN_POINT('Ctrl Pts',(5.66102364641474,-7.46688665624658,4.20183068124527));
#79214=CARTESIAN_POINT('Ctrl Pts',(5.84719339031636,-7.32574197694542,4.2057986929666));
#79215=CARTESIAN_POINT('Ctrl Pts',(6.02806687655178,-7.17764259984669,4.20976670468793));
#79216=CARTESIAN_POINT('Ctrl Pts',(6.20313356829267,-7.02301352671491,4.21373471640925));
#79217=CARTESIAN_POINT('Ctrl Pts',(6.31082868044312,-6.92789094681666,4.21617570311605));
#79218=CARTESIAN_POINT('Ctrl Pts',(6.41632697248547,-6.83029813531336,4.21861668982285));
#79219=CARTESIAN_POINT('Ctrl Pts',(6.51951615140972,-6.73034131482259,4.22105767652964));
#79220=CARTESIAN_POINT('Ctrl Pts',(6.68727388033173,-6.56783852750894,4.2250260614953));
#79221=CARTESIAN_POINT('Ctrl Pts',(6.84897881607757,-6.39903529653706,4.22899444646095));
#79222=CARTESIAN_POINT('Ctrl Pts',(7.00416659244396,-6.22440643015797,4.2329628314266));
#79223=CARTESIAN_POINT('Ctrl Pts',(7.15932727382635,-6.04980805307677,4.23693052353274));
#79224=CARTESIAN_POINT('Ctrl Pts',(7.30797287830809,-5.86938628342057,4.24089821563888));
#79225=CARTESIAN_POINT('Ctrl Pts',(7.44967766344872,-5.68365091936629,4.24486590774502));
#79226=CARTESIAN_POINT('Ctrl Pts',(7.5913670642109,-5.49793571993192,4.24883316909311));
#79227=CARTESIAN_POINT('Ctrl Pts',(7.72611697770568,-5.3069083039586,4.25280043044121));
#79228=CARTESIAN_POINT('Ctrl Pts',(7.85354293705376,-5.11111029017698,4.2567676917893));
#79229=CARTESIAN_POINT('Ctrl Pts',(7.9809788630519,-4.9152969620097,4.26073526343762));
#79230=CARTESIAN_POINT('Ctrl Pts',(8.10108953265346,-4.71471252726251,4.26470283508595));
#79231=CARTESIAN_POINT('Ctrl Pts',(8.21353402334295,-4.50992726215045,4.26867040673428));
#79232=CARTESIAN_POINT('Ctrl Pts',(8.32597733634152,-4.30514414186331,4.27263793682812));
#79233=CARTESIAN_POINT('Ctrl Pts',(8.43075449607761,-4.09616052962373,4.27660546692196));
#79234=CARTESIAN_POINT('Ctrl Pts',(8.52757040875384,-3.8835715502931,4.28057299701581));
#79235=CARTESIAN_POINT('Ctrl Pts',(8.62440715027032,-3.67093683486632,4.28454138067853));
#79236=CARTESIAN_POINT('Ctrl Pts',(8.71327910398296,-3.45469546121587,4.28850976434126));
#79237=CARTESIAN_POINT('Ctrl Pts',(8.7939387006584,-3.2354639839693,4.29247814800399));
#79238=CARTESIAN_POINT('Ctrl Pts',(8.84350826760687,-3.10073470392698,4.29491692860486));
#79239=CARTESIAN_POINT('Ctrl Pts',(8.88997717625413,-2.96487653354668,4.29735570920574));
#79240=CARTESIAN_POINT('Ctrl Pts',(8.93329716455643,-2.82803586119909,4.29979448980662));
#79241=CARTESIAN_POINT('Ctrl Pts',(9.00378208945738,-2.60538565071178,4.3037625718454));
#79242=CARTESIAN_POINT('Ctrl Pts',(9.06594996777659,-2.38006435863928,4.30773065388419));
#79243=CARTESIAN_POINT('Ctrl Pts',(9.11961752138882,-2.15271022807948,4.31169873592298));
#79244=CARTESIAN_POINT('Ctrl Pts',(9.17327565227445,-1.92539601541551,4.31566612126236));
#79245=CARTESIAN_POINT('Ctrl Pts',(9.21843637224543,-1.69604995349702,4.31963350660175));
#79246=CARTESIAN_POINT('Ctrl Pts',(9.25496700757332,-1.46532274643825,4.32360089194114));
#79247=CARTESIAN_POINT('Ctrl Pts',(9.29149364991311,-1.23462075906115,4.32756784362472));
#79248=CARTESIAN_POINT('Ctrl Pts',(9.31939204656531,-1.00253820888336,4.33153479530829));
#79249=CARTESIAN_POINT('Ctrl Pts',(9.33858095781304,-0.769734211836592,
4.33550174699186));
#79250=CARTESIAN_POINT('Ctrl Pts',(9.35777135971476,-0.536912129855148,
4.33946900684052));
#79251=CARTESIAN_POINT('Ctrl Pts',(9.36825089799271,-0.303368772356388,
4.34343626668917));
#79252=CARTESIAN_POINT('Ctrl Pts',(9.36999026231452,-0.069767805119505,
4.34740352653782));
#79253=CARTESIAN_POINT('Ctrl Pts',(9.37172960811471,0.163830674618765,4.35137074414113));
#79254=CARTESIAN_POINT('Ctrl Pts',(9.36472896622191,0.397486478320609,4.35533796174443));
#79255=CARTESIAN_POINT('Ctrl Pts',(9.34901115800388,0.630535827704491,4.35930517934774));
#79256=CARTESIAN_POINT('Ctrl Pts',(9.33328996401887,0.863635378158366,4.36327325152785));
#79257=CARTESIAN_POINT('Ctrl Pts',(9.30884787032399,1.09612792925555,4.36724132370797));
#79258=CARTESIAN_POINT('Ctrl Pts',(9.27575969940313,1.3273534048733,4.37120939588808));
#79259=CARTESIAN_POINT('Ctrl Pts',(9.25540821168189,1.46957288382631,4.37365003161992));
#79260=CARTESIAN_POINT('Ctrl Pts',(9.23178685324645,1.6113131150379,4.37609066735175));
#79261=CARTESIAN_POINT('Ctrl Pts',(9.2049227175773,1.75242198854309,4.37853130308359));
#79262=CARTESIAN_POINT('Ctrl Pts',(9.16124396846532,1.98185274928728,4.38249956460213));
#79263=CARTESIAN_POINT('Ctrl Pts',(9.10897640766371,2.20968525647264,4.38646782612066));
#79264=CARTESIAN_POINT('Ctrl Pts',(9.04826179870715,2.43527072099938,4.3904360876392));
#79265=CARTESIAN_POINT('Ctrl Pts',(8.98755781666017,2.66081670118501,4.39440365459086));
#79266=CARTESIAN_POINT('Ctrl Pts',(8.91840981162146,2.8841161492307,4.39837122154252));
#79267=CARTESIAN_POINT('Ctrl Pts',(8.84100999989763,3.10453333759039,4.40233878849418));
#79268=CARTESIAN_POINT('Ctrl Pts',(8.76361861725768,3.32492652182233,4.40630592336528));
#79269=CARTESIAN_POINT('Ctrl Pts',(8.67797731640622,3.54243780477886,4.41027305823637));
#79270=CARTESIAN_POINT('Ctrl Pts',(8.58432757403525,3.75644847750612,4.41424019310746));
#79271=CARTESIAN_POINT('Ctrl Pts',(8.49067053215933,3.97047583123993,4.41820763719586));
#79272=CARTESIAN_POINT('Ctrl Pts',(8.38900391283925,4.18100176773534,4.42217508128425));
#79273=CARTESIAN_POINT('Ctrl Pts',(8.2796170556023,4.3874282301913,4.42614252537265));
#79274=CARTESIAN_POINT('Ctrl Pts',(8.17023135513512,4.59385250968034,4.43010992750518));
#79275=CARTESIAN_POINT('Ctrl Pts',(8.05312571522298,4.79617715151202,4.43407732963772));
#79276=CARTESIAN_POINT('Ctrl Pts',(7.92863540959037,4.99382875199879,4.43804473177026));
#79277=CARTESIAN_POINT('Ctrl Pts',(7.80411831327078,5.19152288770252,4.44201298769963));
#79278=CARTESIAN_POINT('Ctrl Pts',(7.67221352701147,5.38454173157018,4.445981243629));
#79279=CARTESIAN_POINT('Ctrl Pts',(7.53330033274568,5.57233982803937,4.44994949955837));
#79280=CARTESIAN_POINT('Ctrl Pts',(7.44790157019147,5.68779124453922,4.45238903849243));
#79281=CARTESIAN_POINT('Ctrl Pts',(7.35985494056502,5.80127013253363,4.4548285774265));
#79282=CARTESIAN_POINT('Ctrl Pts',(7.26925637269257,5.9126556512762,4.45726811636056));
#79283=CARTESIAN_POINT('Ctrl Pts',(7.1218891046023,6.09383489050017,4.4612362606321));
#79284=CARTESIAN_POINT('Ctrl Pts',(6.96772199556515,6.26953005321884,4.46520440490365));
#79285=CARTESIAN_POINT('Ctrl Pts',(6.80718780779681,6.43923747130687,4.46917254917519));
#79286=CARTESIAN_POINT('Ctrl Pts',(6.64668232113569,6.60891454825156,4.47313998400199));
#79287=CARTESIAN_POINT('Ctrl Pts',(6.47981222351787,6.77260581099257,4.4771074188288));
#79288=CARTESIAN_POINT('Ctrl Pts',(6.30704847372739,6.92984304386131,4.48107485365561));
#79289=CARTESIAN_POINT('Ctrl Pts',(6.13429054707556,7.08707497692492,4.48504215475689));
#79290=CARTESIAN_POINT('Ctrl Pts',(5.95563957335986,7.23785312094247,4.48900945585817));
#79291=CARTESIAN_POINT('Ctrl Pts',(5.77160190009354,7.38174752814919,4.49297675695945));
#79292=CARTESIAN_POINT('Ctrl Pts',(5.58757698307014,7.52563196157184,4.49694378307434));
#79293=CARTESIAN_POINT('Ctrl Pts',(5.39816633708207,7.66263343692668,4.50091080918922));
#79294=CARTESIAN_POINT('Ctrl Pts',(5.2039083970397,7.79236308559347,4.50487783530411));
#79295=CARTESIAN_POINT('Ctrl Pts',(5.00962904136831,7.92210703607993,4.5088452987569));
#79296=CARTESIAN_POINT('Ctrl Pts',(4.8105015600904,8.04457739943509,4.51281276220968));
#79297=CARTESIAN_POINT('Ctrl Pts',(4.60709330808357,8.15942867565564,4.51678022566247));
#79298=CARTESIAN_POINT('Ctrl Pts',(4.50280292518609,8.2183146031199,4.51881440214518));
#79299=CARTESIAN_POINT('Ctrl Pts',(4.39738767139772,8.27519837060822,4.5208485786279));
#79300=CARTESIAN_POINT('Ctrl Pts',(4.2909266281567,8.33003803918541,4.52288275511062));
#79301=CARTESIAN_POINT('',(5.44031476324452,-7.62919132931687,4.));
#79302=CARTESIAN_POINT('Origin',(0.,0.,4.));
#79303=CARTESIAN_POINT('Ctrl Pts',(5.4403147632445,-7.62919132931689,4.));
#79304=CARTESIAN_POINT('Ctrl Pts',(5.63163361488636,-7.49276340030762,4.00399116231736));
#79305=CARTESIAN_POINT('Ctrl Pts',(5.81783001121082,-7.34912682304943,4.00798232463471));
#79306=CARTESIAN_POINT('Ctrl Pts',(5.99837034461235,-7.19869003856779,4.01197348695207));
#79307=CARTESIAN_POINT('Ctrl Pts',(6.17889790555384,-7.04826389684825,4.01596436691168));
#79308=CARTESIAN_POINT('Ctrl Pts',(6.35376998977345,-6.89103868632153,4.01995524687129));
#79309=CARTESIAN_POINT('Ctrl Pts',(6.52248626448773,-6.72746296846508,4.0239461268309));
#79310=CARTESIAN_POINT('Ctrl Pts',(6.69119837955165,-6.56389128352005,4.02793690839654));
#79311=CARTESIAN_POINT('Ctrl Pts',(6.85375478956946,-6.39396959740036,4.03192768996218));
#79312=CARTESIAN_POINT('Ctrl Pts',(7.00969145999219,-6.21818387459012,4.03591847152781));
#79313=CARTESIAN_POINT('Ctrl Pts',(7.16565269850069,-6.04237045644239,4.03990988184782));
#79314=CARTESIAN_POINT('Ctrl Pts',(7.31499192758445,-5.86069136148633,4.04390129216783));
#79315=CARTESIAN_POINT('Ctrl Pts',(7.45728404103732,-5.67366722621182,4.04789270248784));
#79316=CARTESIAN_POINT('Ctrl Pts',(7.59957951299597,-5.48663867662633,4.05188420701669));
#79317=CARTESIAN_POINT('Ctrl Pts',(7.73482737157571,-5.29426505732967,4.05587571154554));
#79318=CARTESIAN_POINT('Ctrl Pts',(7.86264424336983,-5.0970982494654,4.05986721607439));
#79319=CARTESIAN_POINT('Ctrl Pts',(7.99048979912466,-4.89988719450848,4.06385961635477));
#79320=CARTESIAN_POINT('Ctrl Pts',(8.11090088481625,-4.69788103431545,4.06785201663515));
#79321=CARTESIAN_POINT('Ctrl Pts',(8.22353799921463,-4.4916598087982,4.07184441691554));
#79322=CARTESIAN_POINT('Ctrl Pts',(8.28835611888543,-4.372987804942,4.07414188236935));
#79323=CARTESIAN_POINT('Ctrl Pts',(8.35060068502593,-4.25292046048218,4.07643934782316));
#79324=CARTESIAN_POINT('Ctrl Pts',(8.41021389672587,-4.13157201000043,4.07873681327698));
#79325=CARTESIAN_POINT('Ctrl Pts',(8.51286305170545,-3.92261974011218,4.0826928639695));
#79326=CARTESIAN_POINT('Ctrl Pts',(8.60774154426674,-3.7097985754997,4.08664891466201));
#79327=CARTESIAN_POINT('Ctrl Pts',(8.69457254615899,-3.49370767267074,4.09060496535453));
#79328=CARTESIAN_POINT('Ctrl Pts',(8.78138469611393,-3.27766368548326,4.09456015714622));
#79329=CARTESIAN_POINT('Ctrl Pts',(8.860152735148,-3.05835164405682,4.09851534893791));
#79330=CARTESIAN_POINT('Ctrl Pts',(8.9306479334078,-2.83639076151701,4.1024705407296));
#79331=CARTESIAN_POINT('Ctrl Pts',(9.00113315883176,-2.61446127940588,4.10642517298702));
#79332=CARTESIAN_POINT('Ctrl Pts',(9.06334779259856,-2.38988397867899,4.11037980524445));
#79333=CARTESIAN_POINT('Ctrl Pts',(9.11711265558626,-2.16329422128587,4.11433443750188));
#79334=CARTESIAN_POINT('Ctrl Pts',(9.17088030342069,-1.93669272727321,4.11828927459653));
#79335=CARTESIAN_POINT('Ctrl Pts',(9.21619723620421,-1.70807884785548,4.12224411169117));
#79336=CARTESIAN_POINT('Ctrl Pts',(9.25293491462444,-1.47810031060957,4.12619894878581));
#79337=CARTESIAN_POINT('Ctrl Pts',(9.28967183907163,-1.24812649324858,4.13015370471472));
#79338=CARTESIAN_POINT('Ctrl Pts',(9.31782981766358,-1.01678835886159,4.13410846064363));
#79339=CARTESIAN_POINT('Ctrl Pts',(9.33733182685642,-0.784741624787566,
4.13806321657254));
#79340=CARTESIAN_POINT('Ctrl Pts',(9.35683815486933,-0.552643502772676,
4.14201884830246));
#79341=CARTESIAN_POINT('Ctrl Pts',(9.367684658499,-0.319836754653946,4.14597448003238));
#79342=CARTESIAN_POINT('Ctrl Pts',(9.36984628052905,-0.0869812724440373,
4.1499301117623));
#79343=CARTESIAN_POINT('Ctrl Pts',(9.371220374384,0.0610396501543117,4.15244461669285));
#79344=CARTESIAN_POINT('Ctrl Pts',(9.36908608027918,0.209080203978885,4.1549591216234));
#79345=CARTESIAN_POINT('Ctrl Pts',(9.36344791379007,0.356970906714329,4.15747362655395));
#79346=CARTESIAN_POINT('Ctrl Pts',(9.35453505750838,0.59075764951879,4.16144857498955));
#79347=CARTESIAN_POINT('Ctrl Pts',(9.3368608834607,0.824241622865925,4.16542352342516));
#79348=CARTESIAN_POINT('Ctrl Pts',(9.31046978563811,1.05675798233078,4.16939847186076));
#79349=CARTESIAN_POINT('Ctrl Pts',(9.28408274894252,1.28923856160682,4.17337280862153));
#79350=CARTESIAN_POINT('Ctrl Pts',(9.24898149814363,1.5207515437012,4.1773471453823));
#79351=CARTESIAN_POINT('Ctrl Pts',(9.20526225747678,1.75063755060077,4.18132148214307));
#79352=CARTESIAN_POINT('Ctrl Pts',(9.16154709179196,1.98050213029045,4.18529544846395));
#79353=CARTESIAN_POINT('Ctrl Pts',(9.10921559300724,2.20873976020429,4.18926941478483));
#79354=CARTESIAN_POINT('Ctrl Pts',(9.04841522339024,2.43470059917432,4.1932433811057));
#79355=CARTESIAN_POINT('Ctrl Pts',(8.98760946972035,2.66068144764617,4.19721769933307));
#79356=CARTESIAN_POINT('Ctrl Pts',(8.91833341744046,2.8843848288063,4.20119201756044));
#79357=CARTESIAN_POINT('Ctrl Pts',(8.84078492762598,3.10517421829458,4.20516633578781));
#79358=CARTESIAN_POINT('Ctrl Pts',(8.76323701558619,3.32596196279246,4.20914062440454));
#79359=CARTESIAN_POINT('Ctrl Pts',(8.67741688511913,3.5438354933019,4.21311491302127));
#79360=CARTESIAN_POINT('Ctrl Pts',(8.58357148754597,3.75817583152888,4.217089201638));
#79361=CARTESIAN_POINT('Ctrl Pts',(8.48970657263908,3.97256074681582,4.22106431680051));
#79362=CARTESIAN_POINT('Ctrl Pts',(8.38781316853626,4.18341074254101,4.22503943196302));
#79363=CARTESIAN_POINT('Ctrl Pts',(8.27818590624073,4.39012792116783,4.22901454712552));
#79364=CARTESIAN_POINT('Ctrl Pts',(8.21203553618309,4.51486348034444,4.23141317802732));
#79365=CARTESIAN_POINT('Ctrl Pts',(8.14307013498791,4.63809468964582,4.23381180892912));
#79366=CARTESIAN_POINT('Ctrl Pts',(8.07136251134545,4.75969455668611,4.23621043983092));
#79367=CARTESIAN_POINT('Ctrl Pts',(7.95282183904832,4.96071265292186,4.24017564332322));
#79368=CARTESIAN_POINT('Ctrl Pts',(7.82674836240878,5.15733320729825,4.24414084681553));
#79369=CARTESIAN_POINT('Ctrl Pts',(7.69349381338828,5.34899411159297,4.24810605030783));
#79370=CARTESIAN_POINT('Ctrl Pts',(7.56026374539025,5.54061980467023,4.25207052532793));
#79371=CARTESIAN_POINT('Ctrl Pts',(7.41985540119335,5.72728743222036,4.25603500034802));
#79372=CARTESIAN_POINT('Ctrl Pts',(7.27266360645564,5.90846419383546,4.25999947536812));
#79373=CARTESIAN_POINT('Ctrl Pts',(7.1254887635541,6.08962008962181,4.26396349380616));
#79374=CARTESIAN_POINT('Ctrl Pts',(6.97153220975379,6.26528616061904,4.26792751224421));
#79375=CARTESIAN_POINT('Ctrl Pts',(6.81122940235113,6.43496224472588,4.27189153068225));
#79376=CARTESIAN_POINT('Ctrl Pts',(6.6509146792536,6.60465094126588,4.27585584377537));
#79377=CARTESIAN_POINT('Ctrl Pts',(6.48425295375723,6.76834855171432,4.27982015686848));
#79378=CARTESIAN_POINT('Ctrl Pts',(6.3117177675682,6.92559050804074,4.28378446996159));
#79379=CARTESIAN_POINT('Ctrl Pts',(6.13918454255197,7.08283067702943,4.28774873799315));
#79380=CARTESIAN_POINT('Ctrl Pts',(5.96077820279671,7.23361514805867,4.29171300602471));
#79381=CARTESIAN_POINT('Ctrl Pts',(5.77700720297046,7.37751806770593,4.29567727405627));
#79382=CARTESIAN_POINT('Ctrl Pts',(5.5931958823245,7.52145256079887,4.29964241187978));
#79383=CARTESIAN_POINT('Ctrl Pts',(5.40401777414671,7.65850230917455,4.30360754970329));
#79384=CARTESIAN_POINT('Ctrl Pts',(5.21001331738214,7.78828262810235,4.30757268752681));
#79385=CARTESIAN_POINT('Ctrl Pts',(5.08974018917379,7.86873998046237,4.31003087605384));
#79386=CARTESIAN_POINT('Ctrl Pts',(4.96761272167605,7.9464042405453,4.31248906458086));
#79387=CARTESIAN_POINT('Ctrl Pts',(4.84376519430004,8.0211921685612,4.31494725310789));
#79388=CARTESIAN_POINT('Ctrl Pts',(4.66305789252323,8.13031606439967,4.31853402327109));
#79389=CARTESIAN_POINT('Ctrl Pts',(4.47863653723643,8.23334587002001,4.32212079343428));
#79390=CARTESIAN_POINT('Ctrl Pts',(4.29092662815669,8.33003803918541,4.32570756359748));
#79391=CARTESIAN_POINT('Origin',(0.,0.,2.15141010809499));
#79392=CARTESIAN_POINT('',(4.29092662824368,8.3300380391406,5.52332385470008));
#79393=CARTESIAN_POINT('',(4.29107337327626,8.33032226950541,5.32570196571484));
#79394=CARTESIAN_POINT('',(4.29092662815669,8.33003803918541,2.15141010809499));
#79395=CARTESIAN_POINT('',(-9.37024999988096,-4.72315641780741E-5,4.84858989189159));
#79396=CARTESIAN_POINT('Ctrl Pts',(4.29092662824368,8.3300380391406,5.52332385470008));
#79397=CARTESIAN_POINT('Ctrl Pts',(4.30909507620923,8.32067920106532,5.52297898293736));
#79398=CARTESIAN_POINT('Ctrl Pts',(4.32723302628988,8.31126086070106,5.52263369329497));
#79399=CARTESIAN_POINT('Ctrl Pts',(4.41533040593975,8.26514870907859,5.52095168178576));
#79400=CARTESIAN_POINT('Ctrl Pts',(4.48485443823517,8.22763066811243,5.5196091375804));
#79401=CARTESIAN_POINT('Ctrl Pts',(4.64323615607706,8.1395572955024,5.51651478898844));
#79402=CARTESIAN_POINT('Ctrl Pts',(4.73175753796161,8.08841798492619,5.51475888294013));
#79403=CARTESIAN_POINT('Ctrl Pts',(4.87244379785407,8.00404264613812,5.51192560151866));
#79404=CARTESIAN_POINT('Ctrl Pts',(4.92514727114748,7.9717207419738,5.51085441560341));
#79405=CARTESIAN_POINT('Ctrl Pts',(5.12344530755721,7.84739163462611,5.5067876207667));
#79406=CARTESIAN_POINT('Ctrl Pts',(5.26681327141406,7.75189815671566,5.50377156838725));
#79407=CARTESIAN_POINT('Ctrl Pts',(5.65818993135744,7.47534090837869,5.49535394952008));
#79408=CARTESIAN_POINT('Ctrl Pts',(5.90005409796334,7.28595889095345,5.48993302101319));
#79409=CARTESIAN_POINT('Ctrl Pts',(6.17316694856976,7.04957676464134,5.48369654948811));
#79410=CARTESIAN_POINT('Ctrl Pts',(6.21384049665758,7.01375142378264,5.48276480463732));
#79411=CARTESIAN_POINT('Ctrl Pts',(6.2858505287979,6.94920676426068,5.48111158818323));
#79412=CARTESIAN_POINT('Ctrl Pts',(6.31730671024373,6.92062334409074,5.48038824199516));
#79413=CARTESIAN_POINT('Ctrl Pts',(6.38816371649126,6.85535175472566,5.47875664165225));
#79414=CARTESIAN_POINT('Ctrl Pts',(6.42744493442588,6.81853613192231,5.47785027718395));
#79415=CARTESIAN_POINT('Ctrl Pts',(6.57501729705512,6.67781811277222,5.47443355503534));
#79416=CARTESIAN_POINT('Ctrl Pts',(6.68112443144793,6.57165761287772,5.47195241033107));
#79417=CARTESIAN_POINT('Ctrl Pts',(7.07939359856972,6.153567907938,5.46245236199959));
#79418=CARTESIAN_POINT('Ctrl Pts',(7.35263722660913,5.82434015209542,5.45550655010311));
#79419=CARTESIAN_POINT('Ctrl Pts',(7.65760418600059,5.40107242808615,5.44677835320756));
#79420=CARTESIAN_POINT('Ctrl Pts',(7.71159425174281,5.32370165250565,5.44519179283013));
#79421=CARTESIAN_POINT('Ctrl Pts',(7.80861322335863,5.1800946378015,5.44226050116453));
#79422=CARTESIAN_POINT('Ctrl Pts',(7.85199075973317,5.11410422302103,5.44091862361481));
#79423=CARTESIAN_POINT('Ctrl Pts',(7.94928526458551,4.96193322788634,5.43783496256));
#79424=CARTESIAN_POINT('Ctrl Pts',(8.00264433563143,4.87540779251708,5.43608918833203));
#79425=CARTESIAN_POINT('Ctrl Pts',(8.11407277047682,4.68795919410896,5.43232353170647));
#79426=CARTESIAN_POINT('Ctrl Pts',(8.17169029613192,4.58678710487238,5.43030097009842));
#79427=CARTESIAN_POINT('Ctrl Pts',(8.34969542963781,4.26021812142622,5.42380980846068));
#79428=CARTESIAN_POINT('Ctrl Pts',(8.46275541558365,4.03096049876388,5.41930591136478));
#79429=CARTESIAN_POINT('Ctrl Pts',(8.6391151273044,3.63311915163546,5.4116660329636));
#79430=CARTESIAN_POINT('Ctrl Pts',(8.70718734253554,3.46680744204485,5.40852335375439));
#79431=CARTESIAN_POINT('Ctrl Pts',(8.78992777798511,3.24681696834646,5.40447128498013));
#79432=CARTESIAN_POINT('Ctrl Pts',(8.80895975538209,3.19482062330553,5.40352115035421));
#79433=CARTESIAN_POINT('Ctrl Pts',(8.84168901153034,3.10288620665194,5.40185641789314));
#79434=CARTESIAN_POINT('Ctrl Pts',(8.85557923190739,3.06301874961054,5.40113965774569));
#79435=CARTESIAN_POINT('Ctrl Pts',(8.88907683694042,2.96474180971866,5.39938497313259));
#79436=CARTESIAN_POINT('Ctrl Pts',(8.90837843762463,2.90623031578625,5.39835056772016));
#79437=CARTESIAN_POINT('Ctrl Pts',(8.99669241159858,2.62936331626399,5.39349579251123));
#79438=CARTESIAN_POINT('Ctrl Pts',(9.05826232367745,2.40871545968441,5.38974134843689));
#79439=CARTESIAN_POINT('Ctrl Pts',(9.18390717722119,1.88501051595979,5.38091335775758));
#79440=CARTESIAN_POINT('Ctrl Pts',(9.24116543460513,1.5805937405746,5.37584209895201));
#79441=CARTESIAN_POINT('Ctrl Pts',(9.29694865280996,1.17408758278307,5.36899291985751));
#79442=CARTESIAN_POINT('Ctrl Pts',(9.30903521166844,1.07405738584783,5.36730211041737));
#79443=CARTESIAN_POINT('Ctrl Pts',(9.32771828769406,0.895265271872616,5.36426686005305));
#79444=CARTESIAN_POINT('Ctrl Pts',(9.33493592288354,0.816578008257973,5.36292653471785));
#79445=CARTESIAN_POINT('Ctrl Pts',(9.34853632443067,0.644387788687521,5.35998263484578));
#79446=CARTESIAN_POINT('Ctrl Pts',(9.35451328451033,0.550861312777691,5.35837661627558));
#79447=CARTESIAN_POINT('Ctrl Pts',(9.3702005036311,0.229779900858516,5.35283875658311));
#79448=CARTESIAN_POINT('Ctrl Pts',(9.37301721710175,0.00196992043196061,
5.34886587277333));
#79449=CARTESIAN_POINT('Ctrl Pts',(9.3595110523351,-0.55855710398833,5.33902828124393));
#79450=CARTESIAN_POINT('Ctrl Pts',(9.33375725204855,-0.890734980494798,
5.33313941316707));
#79451=CARTESIAN_POINT('Ctrl Pts',(9.28229772351839,-1.2823343645511,5.32631522602013));
#79452=CARTESIAN_POINT('Ctrl Pts',(9.27360581838168,-1.3437513167376,5.32524874161302));
#79453=CARTESIAN_POINT('Ctrl Pts',(9.25797073376504,-1.44684042484873,5.3234674583097));
#79454=CARTESIAN_POINT('Ctrl Pts',(9.25135441618257,-1.48855997641121,5.32274913503323));
#79455=CARTESIAN_POINT('Ctrl Pts',(9.2353013604433,-1.58553979211666,5.32108547221462));
#79456=CARTESIAN_POINT('Ctrl Pts',(9.22565038432783,-1.64076282757804,5.32014249847219));
#79457=CARTESIAN_POINT('Ctrl Pts',(9.18256055017881,-1.8749131269906,5.31615694757912));
#79458=CARTESIAN_POINT('Ctrl Pts',(9.14440727346621,-2.05293290461334,5.31315778020996));
#79459=CARTESIAN_POINT('Ctrl Pts',(9.00832253669811,-2.60839058020552,5.30376874740674));
#79460=CARTESIAN_POINT('Ctrl Pts',(8.89201073994553,-2.98089268469196,5.29741166381981));
#79461=CARTESIAN_POINT('Ctrl Pts',(8.7191428358556,-3.43322601229582,5.28931012887362));
#79462=CARTESIAN_POINT('Ctrl Pts',(8.68412033788075,-3.52087298069941,5.2877229279646));
#79463=CARTESIAN_POINT('Ctrl Pts',(8.61737472662243,-3.68085225698182,5.28479104534174));
#79464=CARTESIAN_POINT('Ctrl Pts',(8.58604966783635,-3.75334138927913,5.28344922535036));
#79465=CARTESIAN_POINT('Ctrl Pts',(8.51233498054549,-3.91817051417761,5.28036652751484));
#79466=CARTESIAN_POINT('Ctrl Pts',(8.46935224894049,-4.01023433390722,5.2786216689724));
#79467=CARTESIAN_POINT('Ctrl Pts',(8.3739607644635,-4.20617388656357,5.27485849874081));
#79468=CARTESIAN_POINT('Ctrl Pts',(8.32109727711225,-4.3098094696729,5.27283751600699));
#79469=CARTESIAN_POINT('Ctrl Pts',(8.14622343496993,-4.6374206915481,5.26635639966138));
#79470=CARTESIAN_POINT('Ctrl Pts',(8.01699369787421,-4.85741068153063,5.26186109976634));
#79471=CARTESIAN_POINT('Ctrl Pts',(7.7815146890906,-5.22321928561321,5.25422330514409));
#79472=CARTESIAN_POINT('Ctrl Pts',(7.67973553178773,-5.37174580836739,5.25107432771301));
#79473=CARTESIAN_POINT('Ctrl Pts',(7.5410520259919,-5.56212204368915,5.24701342822879));
#79474=CARTESIAN_POINT('Ctrl Pts',(7.50796466713723,-5.60670436742131,5.24606068472085));
#79475=CARTESIAN_POINT('Ctrl Pts',(7.44902844620289,-5.68465845638359,5.24439350454844));
#79476=CARTESIAN_POINT('Ctrl Pts',(7.42334678089738,-5.71815434680769,5.24367687489309));
#79477=CARTESIAN_POINT('Ctrl Pts',(7.35974181281689,-5.79996185612797,5.24192556279333));
#79478=CARTESIAN_POINT('Ctrl Pts',(7.32156822988528,-5.8480762446981,5.24089435937829));
#79479=CARTESIAN_POINT('Ctrl Pts',(7.13622975671459,-6.077019449251,5.23597328820953));
#79480=CARTESIAN_POINT('Ctrl Pts',(6.9828227890841,-6.25268959347655,5.23215205934308));
#79481=CARTESIAN_POINT('Ctrl Pts',(6.6146762197271,-6.64379744760478,5.22334805705528));
#79482=CARTESIAN_POINT('Ctrl Pts',(6.3956817480936,-6.8548698365087,5.21836708433383));
#79483=CARTESIAN_POINT('Ctrl Pts',(6.09042649808538,-7.12169814943474,5.21160070412585));
#79484=CARTESIAN_POINT('Ctrl Pts',(6.0129562276732,-7.18722733731433,5.20989828161544));
#79485=CARTESIAN_POINT('Ctrl Pts',(5.87325348178848,-7.30155662718354,5.20685067965745));
#79486=CARTESIAN_POINT('Ctrl Pts',(5.81143859198803,-7.35085145402365,5.20550975404875));
#79487=CARTESIAN_POINT('Ctrl Pts',(5.675410858047,-7.45653960185108,5.20257418559018));
#79488=CARTESIAN_POINT('Ctrl Pts',(5.60096544796234,-7.51261986511956,5.2009772018096));
#79489=CARTESIAN_POINT('Ctrl Pts',(5.34736987280335,-7.69779029270513,5.1955688007151));
#79490=CARTESIAN_POINT('Ctrl Pts',(5.16449760945591,-7.82165607741675,5.19171922486761));
#79491=CARTESIAN_POINT('Ctrl Pts',(4.77465652949561,-8.06607183300903,5.18364917760876));
#79492=CARTESIAN_POINT('Ctrl Pts',(4.56709572181718,-8.1853830936207,5.17942735316141));
#79493=CARTESIAN_POINT('Ctrl Pts',(4.24421777957966,-8.35487345114201,5.17305040822101));
#79494=CARTESIAN_POINT('Ctrl Pts',(4.13208193362544,-8.41089733506212,5.17086980193708));
#79495=CARTESIAN_POINT('Ctrl Pts',(3.97184818325022,-8.48697324727121,5.16781689051998));
#79496=CARTESIAN_POINT('Ctrl Pts',(3.92465535052403,-8.50889965192357,5.16692535859639));
#79497=CARTESIAN_POINT('Ctrl Pts',(3.83824324230581,-8.54817599114268,5.16530838173322));
#79498=CARTESIAN_POINT('Ctrl Pts',(3.79908294871078,-8.56565191386198,5.1645814989491));
#79499=CARTESIAN_POINT('Ctrl Pts',(3.69689646509036,-8.61041568987403,5.16269892566188));
#79500=CARTESIAN_POINT('Ctrl Pts',(3.63368772189618,-8.63728055575679,5.16154821345073));
#79501=CARTESIAN_POINT('Ctrl Pts',(3.48757958020344,-8.69749142219622,5.15891419232269));
#79502=CARTESIAN_POINT('Ctrl Pts',(3.404487059831,-8.73035144054452,5.15743513315476));
#79503=CARTESIAN_POINT('Ctrl Pts',(3.08448492985425,-8.85163708170513,5.15179204931195));
#79504=CARTESIAN_POINT('Ctrl Pts',(2.84450167840352,-8.93164804660555,5.14766751778081));
#79505=CARTESIAN_POINT('Ctrl Pts',(2.40543244206359,-9.05854103613891,5.14015352979828));
#79506=CARTESIAN_POINT('Ctrl Pts',(2.20748849201208,-9.10880152014438,5.13677812701546));
#79507=CARTESIAN_POINT('Ctrl Pts',(1.91621330759283,-9.1727070053693,5.13178848039399));
#79508=CARTESIAN_POINT('Ctrl Pts',(1.82406706618621,-9.19147466572156,5.13020694851042));
#79509=CARTESIAN_POINT('Ctrl Pts',(1.65402536571385,-9.22344970516967,5.12728027256988));
#79510=CARTESIAN_POINT('Ctrl Pts',(1.57621524195944,-9.237065002016,5.12593791945143));
#79511=CARTESIAN_POINT('Ctrl Pts',(1.39749140633512,-9.26601424108131,5.12284655789034));
#79512=CARTESIAN_POINT('Ctrl Pts',(1.29648070178976,-9.28068638980815,5.12109347874753));
#79513=CARTESIAN_POINT('Ctrl Pts',(1.13407825325526,-9.30157274539724,5.11826564271921));
#79514=CARTESIAN_POINT('Ctrl Pts',(1.07282970459229,-9.30883587961009,5.11719706510379));
#79515=CARTESIAN_POINT('Ctrl Pts',(0.840940592752878,-9.33401533690024,
5.11314435610554));
#79516=CARTESIAN_POINT('Ctrl Pts',(0.669891012023075,-9.34784837302521,
5.11013991607962));
#79517=CARTESIAN_POINT('Ctrl Pts',(0.189337248990873,-9.37345324890715,
5.1016873489309));
#79518=CARTESIAN_POINT('Ctrl Pts',(-0.120510981533038,-9.37459075531224,
5.09621887966962));
#79519=CARTESIAN_POINT('Ctrl Pts',(-0.483389314709819,-9.35792673690669,
5.08994832228886));
#79520=CARTESIAN_POINT('Ctrl Pts',(-0.536911076156703,-9.35500852782843,
5.08902709174467));
#79521=CARTESIAN_POINT('Ctrl Pts',(-0.632744057619878,-9.34895821832732,
5.08738577131017));
#79522=CARTESIAN_POINT('Ctrl Pts',(-0.675064556748423,-9.34599768205513,
5.0866639081461));
#79523=CARTESIAN_POINT('Ctrl Pts',(-0.771557788055997,-9.33858864907045,
5.08502515085003));
#79524=CARTESIAN_POINT('Ctrl Pts',(-0.825714729355456,-9.33395599843451,
5.08411025858169));
#79525=CARTESIAN_POINT('Ctrl Pts',(-1.03542689403885,-9.31417749798637,
5.08058151734085));
#79526=CARTESIAN_POINT('Ctrl Pts',(-1.1906343964783,-9.29561193914324,5.07799942852732));
#79527=CARTESIAN_POINT('Ctrl Pts',(-1.6677299979759,-9.22639732005442,5.07007179193347));
#79528=CARTESIAN_POINT('Ctrl Pts',(-1.98749561648295,-9.1628375654723,5.06476480547068));
#79529=CARTESIAN_POINT('Ctrl Pts',(-2.43560509423968,-9.0492012474576,5.05710358327929));
#79530=CARTESIAN_POINT('Ctrl Pts',(-2.56716098837107,-9.01276315605733,
5.05482762174399));
#79531=CARTESIAN_POINT('Ctrl Pts',(-2.77765854105335,-8.9494770304733,5.05113242463971));
#79532=CARTESIAN_POINT('Ctrl Pts',(-2.85711987703535,-8.9244267075862,5.04972512089733));
#79533=CARTESIAN_POINT('Ctrl Pts',(-3.01478295436201,-8.87240159829483,
5.04690646764129));
#79534=CARTESIAN_POINT('Ctrl Pts',(-3.09298270675076,-8.84544426924775,
5.04549534488736));
#79535=CARTESIAN_POINT('Ctrl Pts',(-3.29543773716293,-8.77264010189487,
5.04180709418841));
#79536=CARTESIAN_POINT('Ctrl Pts',(-3.41909588813482,-8.72518810101619,
5.03951958685846));
#79537=CARTESIAN_POINT('Ctrl Pts',(-3.70411089490155,-8.60882796228113,
5.03416912915469));
#79538=CARTESIAN_POINT('Ctrl Pts',(-3.86462120026677,-8.53797746290866,
5.03109618261708));
#79539=CARTESIAN_POINT('Ctrl Pts',(-4.29836974891504,-8.33177866316471,
5.02265890395396));
#79540=CARTESIAN_POINT('Ctrl Pts',(-4.56714084589703,-8.18753583542816,
5.01727751785577));
#79541=CARTESIAN_POINT('Ctrl Pts',(-4.87352912645226,-8.00331628677599,
5.01110860639607));
#79542=CARTESIAN_POINT('Ctrl Pts',(-4.91842681612778,-7.97580311960925,
5.01020391518273));
#79543=CARTESIAN_POINT('Ctrl Pts',(-4.99898258372196,-7.92549990805732,
5.00858103466217));
#79544=CARTESIAN_POINT('Ctrl Pts',(-5.03472264660238,-7.90284401676706,
5.00786123290643));
#79545=CARTESIAN_POINT('Ctrl Pts',(-5.11675589977332,-7.85006017285951,
5.00620988021578));
#79546=CARTESIAN_POINT('Ctrl Pts',(-5.16293852386699,-7.81976351771826,
5.00528051957097));
#79547=CARTESIAN_POINT('Ctrl Pts',(-5.34872575716939,-7.69552029511861,
5.00153775658285));
#79548=CARTESIAN_POINT('Ctrl Pts',(-5.48605626666353,-7.5982291888244,4.99876131523456));
#79549=CARTESIAN_POINT('Ctrl Pts',(-5.93190998958374,-7.26397430503297,
4.98960562722068));
#79550=CARTESIAN_POINT('Ctrl Pts',(-6.22829694162656,-7.01150455702873,
4.98327068926761));
#79551=CARTESIAN_POINT('Ctrl Pts',(-6.58021918381101,-6.67175686134455,
4.9751016317372));
#79552=CARTESIAN_POINT('Ctrl Pts',(-6.65118275884932,-6.60101446507654,
4.97341936824743));
#79553=CARTESIAN_POINT('Ctrl Pts',(-6.775979279902,-6.47255096499091,4.97039400392658));
#79554=CARTESIAN_POINT('Ctrl Pts',(-6.83024335164318,-6.41526203048747,
4.9690549279602));
#79555=CARTESIAN_POINT('Ctrl Pts',(-6.94106091539931,-6.29526705291492,
4.96626984407561));
#79556=CARTESIAN_POINT('Ctrl Pts',(-6.9975034646115,-6.23246814039217,4.96482303795468));
#79557=CARTESIAN_POINT('Ctrl Pts',(-7.07247150911673,-6.14675512301173,
4.96286256331029));
#79558=CARTESIAN_POINT('Ctrl Pts',(-7.09174896482245,-6.1245039315732,4.96235489540127));
#79559=CARTESIAN_POINT('Ctrl Pts',(-7.14436707674367,-6.06318742893959,
4.96095945445767));
#79560=CARTESIAN_POINT('Ctrl Pts',(-7.17749190410883,-6.0239383034768,4.96007009994488));
#79561=CARTESIAN_POINT('Ctrl Pts',(-7.31276281609086,-5.86095793001278,
4.9563934710575));
#79562=CARTESIAN_POINT('Ctrl Pts',(-7.41204515851131,-5.73488572178633,
4.95358743790647));
#79563=CARTESIAN_POINT('Ctrl Pts',(-7.70580535318572,-5.34147954251365,
4.94497010133452));
#79564=CARTESIAN_POINT('Ctrl Pts',(-7.88941712361181,-5.06635346696581,
4.93912543085288));
#79565=CARTESIAN_POINT('Ctrl Pts',(-8.08791570527353,-4.73187238007334,
4.93241108558769));
#79566=CARTESIAN_POINT('Ctrl Pts',(-8.11725446204665,-4.68136483270345,
4.93140752800033));
#79567=CARTESIAN_POINT('Ctrl Pts',(-8.1595668887964,-4.60692888611154,4.92994536341637));
#79568=CARTESIAN_POINT('Ctrl Pts',(-8.17291157676088,-4.58321305838657,
4.92948199469067));
#79569=CARTESIAN_POINT('Ctrl Pts',(-8.20501409254679,-4.52557524869298,
4.92836212830084));
#79570=CARTESIAN_POINT('Ctrl Pts',(-8.22366509940608,-4.49159436396222,
4.9277070783752));
#79571=CARTESIAN_POINT('Ctrl Pts',(-8.26571891481978,-4.41383506998117,
4.92621882304978));
#79572=CARTESIAN_POINT('Ctrl Pts',(-8.28898578134038,-4.3699844316459,4.92538722935787));
#79573=CARTESIAN_POINT('Ctrl Pts',(-8.33188936037925,-4.28754928659676,
4.92383647634219));
#79574=CARTESIAN_POINT('Ctrl Pts',(-8.35160924465963,-4.24900955865545,
4.92311655950612));
#79575=CARTESIAN_POINT('Ctrl Pts',(-8.4890706996906,-3.97570626977537,4.91804294957473));
#79576=CARTESIAN_POINT('Ctrl Pts',(-8.59716371885337,-3.73621979453179,
4.91375796074802));
#79577=CARTESIAN_POINT('Ctrl Pts',(-8.7836339157327,-3.27197810478023,4.90554848595926));
#79578=CARTESIAN_POINT('Ctrl Pts',(-8.86379163783522,-3.04815728187916,
4.90163179999078));
#79579=CARTESIAN_POINT('Ctrl Pts',(-8.96469883642099,-2.7285999022936,4.89603082504856));
#79580=CARTESIAN_POINT('Ctrl Pts',(-8.99259261697984,-2.63521547886795,
4.89439336229877));
#79581=CARTESIAN_POINT('Ctrl Pts',(-9.04041372930677,-2.46550682924856,
4.89141331303917));
#79582=CARTESIAN_POINT('Ctrl Pts',(-9.06084372199404,-2.38933365902394,
4.89007420702657));
#79583=CARTESIAN_POINT('Ctrl Pts',(-9.09895901610244,-2.23969601352763,
4.88743978025226));
#79584=CARTESIAN_POINT('Ctrl Pts',(-9.11672210829258,-2.16625745950231,
4.88614507862456));
#79585=CARTESIAN_POINT('Ctrl Pts',(-9.1742065975365,-1.91535571926908,4.88171552388456));
#79586=CARTESIAN_POINT('Ctrl Pts',(-9.2096493356327,-1.73695509247306,4.87855461468278));
#79587=CARTESIAN_POINT('Ctrl Pts',(-9.28017682298766,-1.31858710597104,
4.87113282955306));
#79588=CARTESIAN_POINT('Ctrl Pts',(-9.31118319396439,-1.07806358201149,
4.86685789418943));
#79589=CARTESIAN_POINT('Ctrl Pts',(-9.34726139722848,-0.675591935739253,
4.85977058185828));
#79590=CARTESIAN_POINT('Ctrl Pts',(-9.35752588391314,-0.51422725676902,
4.8569473045786));
#79591=CARTESIAN_POINT('Ctrl Pts',(-9.36564690581209,-0.298613729662839,
4.85322873812419));
#79592=CARTESIAN_POINT('Ctrl Pts',(-9.36721494029457,-0.244533032443576,
4.85230060338259));
#79593=CARTESIAN_POINT('Ctrl Pts',(-9.36895425008626,-0.158971942375714,
4.85084096482924));
#79594=CARTESIAN_POINT('Ctrl Pts',(-9.36943540354766,-0.127499186728518,
4.85030597995095));
#79595=CARTESIAN_POINT('Ctrl Pts',(-9.37008580015194,-0.0640355894891263,
4.84923110042245));
#79596=CARTESIAN_POINT('Ctrl Pts',(-9.37024981349469,-0.0320452041784548,
4.84869121345059));
#79597=CARTESIAN_POINT('Ctrl Pts',(-9.37024999984103,-5.45819878978748E-5,
4.8481529963742));
#79598=CARTESIAN_POINT('Ctrl Pts',(4.2909266281567,8.33003803918541,4.52288275511062));
#79599=CARTESIAN_POINT('Ctrl Pts',(4.08324923132093,8.4370157586096,4.52685089654315));
#79600=CARTESIAN_POINT('Ctrl Pts',(3.87159094101272,8.5362119836809,4.53081903797568));
#79601=CARTESIAN_POINT('Ctrl Pts',(3.6565558870526,8.62735093220167,4.53478717940821));
#79602=CARTESIAN_POINT('Ctrl Pts',(3.63455910839878,8.63667389253038,4.53519309615132));
#79603=CARTESIAN_POINT('Ctrl Pts',(3.61252701312059,8.64591258237561,4.53559901289443));
#79604=CARTESIAN_POINT('Ctrl Pts',(3.59046025986583,8.65506673485677,4.53600492963755));
#79605=CARTESIAN_POINT('Ctrl Pts',(3.37473763072933,8.74455692029336,4.53997313583552));
#79606=CARTESIAN_POINT('Ctrl Pts',(3.15563410300656,8.82599184272615,4.54394134203349));
#79607=CARTESIAN_POINT('Ctrl Pts',(2.93376971124411,8.89913368502163,4.54790954823147));
#79608=CARTESIAN_POINT('Ctrl Pts',(2.71194418949467,8.97226271307352,4.55187705921096));
#79609=CARTESIAN_POINT('Ctrl Pts',(2.48735903927923,9.0371014721892,4.55584457019044));
#79610=CARTESIAN_POINT('Ctrl Pts',(2.26065108681041,9.09346148208717,4.55981208116993));
#79611=CARTESIAN_POINT('Ctrl Pts',(2.03396785131846,9.14981534729967,4.56377915958904));
#79612=CARTESIAN_POINT('Ctrl Pts',(1.80516255165042,9.19769224036156,4.56774623800816));
#79613=CARTESIAN_POINT('Ctrl Pts',(1.57488484377305,9.2369541945034,4.57171331642727));
#79614=CARTESIAN_POINT('Ctrl Pts',(1.34458920502211,9.27621920582842,4.57568070374811));
#79615=CARTESIAN_POINT('Ctrl Pts',(1.11282120893339,9.30686788712794,4.57964809106895));
#79616=CARTESIAN_POINT('Ctrl Pts',(0.880239536965458,9.32881361267674,4.58361547838978));
#79617=CARTESIAN_POINT('Ctrl Pts',(0.647660329530003,9.35075910567947,4.58758282367053));
#79618=CARTESIAN_POINT('Ctrl Pts',(0.4142677469141,9.36400180288017,4.59155016895128));
#79619=CARTESIAN_POINT('Ctrl Pts',(0.18072509314386,9.3685070050253,4.59551751423203));
#79620=CARTESIAN_POINT('Ctrl Pts',(-0.0528678350307668,9.37301317699907,
4.59948571355771));
#79621=CARTESIAN_POINT('Ctrl Pts',(-0.286610614390155,9.36877808960251,
4.60345391288339));
#79622=CARTESIAN_POINT('Ctrl Pts',(-0.519839129798677,9.35581916999416,
4.60742211220908));
#79623=CARTESIAN_POINT('Ctrl Pts',(-0.663241419070258,9.34785128178346,
4.60986198911089));
#79624=CARTESIAN_POINT('Ctrl Pts',(-0.806449300964467,9.33658637512197,
4.6123018660127));
#79625=CARTESIAN_POINT('Ctrl Pts',(-0.949309040297671,9.32203826469883,
4.61474174291451));
#79626=CARTESIAN_POINT('Ctrl Pts',(-1.1816554027776,9.29837729098048,4.61870994645234));
#79627=CARTESIAN_POINT('Ctrl Pts',(-1.4131527990255,9.26602167570447,4.62267814999016));
#79628=CARTESIAN_POINT('Ctrl Pts',(-1.64314262419167,9.22505649733727,4.62664635352799));
#79629=CARTESIAN_POINT('Ctrl Pts',(-1.87309215598527,9.18409849591884,4.63061386185113));
#79630=CARTESIAN_POINT('Ctrl Pts',(-2.1015343639731,9.13453399216639,4.63458137017427));
#79631=CARTESIAN_POINT('Ctrl Pts',(-2.32781928923107,9.07649945844673,4.63854887849741));
#79632=CARTESIAN_POINT('Ctrl Pts',(-2.55407954429396,9.01847125180903,4.64251595427205));
#79633=CARTESIAN_POINT('Ctrl Pts',(-2.77818271075123,8.95197492958084,4.6464830300467));
#79634=CARTESIAN_POINT('Ctrl Pts',(-2.99949152115984,8.87719751255937,4.65045010582134));
#79635=CARTESIAN_POINT('Ctrl Pts',(-3.22081756616842,8.80241427218696,4.65441749053517));
#79636=CARTESIAN_POINT('Ctrl Pts',(-3.43934854982918,8.71934873670342,4.658384875249));
#79637=CARTESIAN_POINT('Ctrl Pts',(-3.65446363721919,8.6282373974493,4.66235225996283));
#79638=CARTESIAN_POINT('Ctrl Pts',(-3.86957644654803,8.53712702306105,4.6663196026622));
#79639=CARTESIAN_POINT('Ctrl Pts',(-4.08127317085655,8.43797112833676,4.67028694536157));
#79640=CARTESIAN_POINT('Ctrl Pts',(-4.28895356073467,8.33105409995406,4.67425428806094));
#79641=CARTESIAN_POINT('Ctrl Pts',(-4.49667866070997,8.22411405413226,4.6782224848625));
#79642=CARTESIAN_POINT('Ctrl Pts',(-4.70038544530948,8.1094096658853,4.68219068166407));
#79643=CARTESIAN_POINT('Ctrl Pts',(-4.89949770003467,7.98727158357941,4.68615887846563));
#79644=CARTESIAN_POINT('Ctrl Pts',(-5.02192421672368,7.91217354407187,4.68859877104092));
#79645=CARTESIAN_POINT('Ctrl Pts',(-5.14261424304615,7.83426605531338,4.6910386636162));
#79646=CARTESIAN_POINT('Ctrl Pts',(-5.26143903274313,7.75363426834327,4.69347855619149));
#79647=CARTESIAN_POINT('Ctrl Pts',(-5.45469360010939,7.62249613507483,4.69744675495926));
#79648=CARTESIAN_POINT('Ctrl Pts',(-5.64307293369046,7.48410891559784,4.70141495372704));
#79649=CARTESIAN_POINT('Ctrl Pts',(-5.82603778824631,7.33886018073829,4.70538315249482));
#79650=CARTESIAN_POINT('Ctrl Pts',(-6.00897058460416,7.19363689564456,4.70935065597441));
#79651=CARTESIAN_POINT('Ctrl Pts',(-6.18649057295735,7.04155467179857,4.713318159454));
#79652=CARTESIAN_POINT('Ctrl Pts',(-6.35809051827845,6.88304220703881,4.71728566293359));
#79653=CARTESIAN_POINT('Ctrl Pts',(-6.52967175275135,6.72454702609963,4.72125273380607));
#79654=CARTESIAN_POINT('Ctrl Pts',(-6.69533402412701,6.5596231971171,4.72521980467856));
#79655=CARTESIAN_POINT('Ctrl Pts',(-6.85460526669439,6.38873788007503,4.72918687555104));
#79656=CARTESIAN_POINT('Ctrl Pts',(-7.01388891051791,6.21783925747601,4.73315425530956));
#79657=CARTESIAN_POINT('Ctrl Pts',(-7.16678033507799,6.04097842544005,4.73712163506808));
#79658=CARTESIAN_POINT('Ctrl Pts',(-7.31284542473205,5.85865828125139,4.7410890148266));
#79659=CARTESIAN_POINT('Ctrl Pts',(-7.45890896675378,5.67634006883543,4.74505635254875));
#79660=CARTESIAN_POINT('Ctrl Pts',(-7.5981461423945,5.48856288339455,4.74902369027091));
#79661=CARTESIAN_POINT('Ctrl Pts',(-7.73016369326455,5.29586200139643,4.75299102799306));
#79662=CARTESIAN_POINT('Ctrl Pts',(-7.86220966529799,5.10311963413203,4.75695921981645));
#79663=CARTESIAN_POINT('Ctrl Pts',(-7.98703274566321,4.90545168679088,4.76092741163984));
#79664=CARTESIAN_POINT('Ctrl Pts',(-8.10428279342827,4.70342273952092,4.76489560346324));
#79665=CARTESIAN_POINT('Ctrl Pts',(-8.17637632720368,4.579201206044,4.76733552546498));
#79666=CARTESIAN_POINT('Ctrl Pts',(-8.24560762261028,4.45333148453508,4.76977544746672));
#79667=CARTESIAN_POINT('Ctrl Pts',(-8.3119037953007,4.32594964836229,4.77221536946846));
#79668=CARTESIAN_POINT('Ctrl Pts',(-8.41958533930194,4.11904972880207,4.77617841224646));
#79669=CARTESIAN_POINT('Ctrl Pts',(-8.51955540201662,3.90809337079972,4.78014145502446));
#79670=CARTESIAN_POINT('Ctrl Pts',(-8.61152381266068,3.69367603973035,4.78410449780246));
#79671=CARTESIAN_POINT('Ctrl Pts',(-8.70347571661736,3.47929719274295,4.78806682928506));
#79672=CARTESIAN_POINT('Ctrl Pts',(-8.78742872247465,3.2614588753116,4.79202916076765));
#79673=CARTESIAN_POINT('Ctrl Pts',(-8.86314034588119,3.04077757682359,4.79599149225024));
#79674=CARTESIAN_POINT('Ctrl Pts',(-8.93884369382226,2.82012039934083,4.79995339064032));
#79675=CARTESIAN_POINT('Ctrl Pts',(-9.0063073650719,2.59662113164217,4.8039152890304));
#79676=CARTESIAN_POINT('Ctrl Pts',(-9.06533808393958,2.37091342869679,4.80787718742048));
#79677=CARTESIAN_POINT('Ctrl Pts',(-9.12437314964507,2.14518910534093,4.81183937755238));
#79678=CARTESIAN_POINT('Ctrl Pts',(-9.17497394725667,1.91725629782274,4.81580156768429));
#79679=CARTESIAN_POINT('Ctrl Pts',(-9.21699757135214,1.68776207807521,4.8197637578162));
#79680=CARTESIAN_POINT('Ctrl Pts',(-9.25902113879243,1.45826816772595,4.82372594260638));
#79681=CARTESIAN_POINT('Ctrl Pts',(-9.29246750688886,1.22721313113998,4.82768812739656));
#79682=CARTESIAN_POINT('Ctrl Pts',(-9.31724510133541,0.995253125662686,
4.83165031218674));
#79683=CARTESIAN_POINT('Ctrl Pts',(-9.34202778586263,0.763245468459468,
4.83561331093165));
#79684=CARTESIAN_POINT('Ctrl Pts',(-9.35813810845432,0.530332755368636,
4.83957630967657));
#79685=CARTESIAN_POINT('Ctrl Pts',(-9.36553635714658,0.297176387799428,
4.84353930842148));
#79686=CARTESIAN_POINT('Ctrl Pts',(-9.36867921898414,0.198128859080778,
4.84522283624485));
#79687=CARTESIAN_POINT('Ctrl Pts',(-9.37025049932568,0.0990373939094512,
4.84690636406822));
#79688=CARTESIAN_POINT('Ctrl Pts',(-9.37024999988096,-4.72315641784071E-5,
4.84858989189159));
#79689=CARTESIAN_POINT('',(-9.37024999716748,0.000230397442772534,4.65141010809498));
#79690=CARTESIAN_POINT('Ctrl Pts',(4.29092662815669,8.33003803918541,4.32570756359748));
#79691=CARTESIAN_POINT('Ctrl Pts',(4.08323685626887,8.43702213318318,4.32967610996065));
#79692=CARTESIAN_POINT('Ctrl Pts',(3.87152104582792,8.53624681226013,4.33364465632381));
#79693=CARTESIAN_POINT('Ctrl Pts',(3.65637888263525,8.62742595037008,4.33761320268698));
#79694=CARTESIAN_POINT('Ctrl Pts',(3.44126117347791,8.7185947246451,4.34158129796714));
#79695=CARTESIAN_POINT('Ctrl Pts',(3.22271815071608,8.80171967295272,4.3455493932473));
#79696=CARTESIAN_POINT('Ctrl Pts',(3.00137009412446,8.87656254529845,4.34951748852746));
#79697=CARTESIAN_POINT('Ctrl Pts',(2.78000532367065,8.95141106898567,4.35348588343617));
#79698=CARTESIAN_POINT('Ctrl Pts',(2.55583536440449,9.01797617310764,4.35745427834489));
#79699=CARTESIAN_POINT('Ctrl Pts',(2.32949747142113,9.07606889535016,4.3614226732536));
#79700=CARTESIAN_POINT('Ctrl Pts',(2.10316342368601,9.13416063065701,4.36539100074337));
#79701=CARTESIAN_POINT('Ctrl Pts',(1.87466179169094,9.18378020323483,4.36935932823313));
#79702=CARTESIAN_POINT('Ctrl Pts',(1.64464254583845,9.2247892094572,4.37332765572289));
#79703=CARTESIAN_POINT('Ctrl Pts',(1.41457270427431,9.26580723614152,4.37729685609767));
#79704=CARTESIAN_POINT('Ctrl Pts',(1.18298486156662,9.29821086110538,4.38126605647245));
#79705=CARTESIAN_POINT('Ctrl Pts',(0.950537996967608,9.32191303214211,4.38523525684723));
#79706=CARTESIAN_POINT('Ctrl Pts',(0.785609791352374,9.33873045209318,4.38805152669311));
#79707=CARTESIAN_POINT('Ctrl Pts',(0.620249312325084,9.35116833922283,4.39086779653899));
#79708=CARTESIAN_POINT('Ctrl Pts',(0.454693388915478,9.35921145100251,4.39368406638487));
#79709=CARTESIAN_POINT('Ctrl Pts',(0.221425913977992,9.37054415560678,4.3976521766292));
#79710=CARTESIAN_POINT('Ctrl Pts',(-0.0123016923509516,9.37315340084888,
4.40162028687353));
#79711=CARTESIAN_POINT('Ctrl Pts',(-0.245825537082703,9.36702486747089,
4.40558839711786));
#79712=CARTESIAN_POINT('Ctrl Pts',(-0.479308478010276,9.3608974075607,4.40955581231195));
#79713=CARTESIAN_POINT('Ctrl Pts',(-0.712587444304115,9.34603523157118,
4.41352322750604));
#79714=CARTESIAN_POINT('Ctrl Pts',(-0.944999409875851,9.32247612911046,
4.41749064270013));
#79715=CARTESIAN_POINT('Ctrl Pts',(-1.17738606289793,9.2989195925286,4.42145762579343));
#79716=CARTESIAN_POINT('Ctrl Pts',(-1.40890562077441,9.26666804936217,4.42542460888673));
#79717=CARTESIAN_POINT('Ctrl Pts',(-1.63890005106618,9.22581116678178,4.42939159198003));
#79718=CARTESIAN_POINT('Ctrl Pts',(-1.86891247163174,9.18495108835658,4.43335888537263));
#79719=CARTESIAN_POINT('Ctrl Pts',(-2.09739924558008,9.13548437240156,4.43732617876524));
#79720=CARTESIAN_POINT('Ctrl Pts',(-2.32371119420569,9.07755205704838,4.44129347215784));
#79721=CARTESIAN_POINT('Ctrl Pts',(-2.55002079889967,9.01962034170499,4.44526072446086));
#79722=CARTESIAN_POINT('Ctrl Pts',(-2.7741553482376,8.95322327506606,4.44922797676388));
#79723=CARTESIAN_POINT('Ctrl Pts',(-2.99547885963476,8.87855232929227,4.4531952290669));
#79724=CARTESIAN_POINT('Ctrl Pts',(-3.21685013360765,8.80386526920383,4.4571633375202));
#79725=CARTESIAN_POINT('Ctrl Pts',(-3.43540888766111,8.72090085272899,4.46113144597351));
#79726=CARTESIAN_POINT('Ctrl Pts',(-3.65053599001042,8.62989988633348,4.46509955442682));
#79727=CARTESIAN_POINT('Ctrl Pts',(-3.78284214223221,8.57393302962054,4.46753999617183));
#79728=CARTESIAN_POINT('Ctrl Pts',(-3.91385065471667,8.51492737183186,4.46998043791684));
#79729=CARTESIAN_POINT('Ctrl Pts',(-4.04342140416922,8.45294791246263,4.47242087966185));
#79730=CARTESIAN_POINT('Ctrl Pts',(-4.25409642109582,8.35217267031204,4.47638890568709));
#79731=CARTESIAN_POINT('Ctrl Pts',(-4.4610349470167,8.2435017315231,4.48035693171233));
#79732=CARTESIAN_POINT('Ctrl Pts',(-4.66364590191146,8.12723765889029,4.48432495773758));
#79733=CARTESIAN_POINT('Ctrl Pts',(-4.86622121919317,8.01099403615879,4.48829228581943));
#79734=CARTESIAN_POINT('Ctrl Pts',(-5.06447023819458,7.88716008710131,4.49225961390129));
#79735=CARTESIAN_POINT('Ctrl Pts',(-5.25782737985817,7.75608382536662,4.49622694198314));
#79736=CARTESIAN_POINT('Ctrl Pts',(-5.45116333425983,7.62502192641713,4.50019383534188));
#79737=CARTESIAN_POINT('Ctrl Pts',(-5.63960824613416,7.48671945886708,4.50416072870062));
#79738=CARTESIAN_POINT('Ctrl Pts',(-5.82262555986898,7.3415677244074,4.50812762205936));
#79739=CARTESIAN_POINT('Ctrl Pts',(-6.0056570360086,7.19640475769008,4.51209482238769));
#79740=CARTESIAN_POINT('Ctrl Pts',(-6.18325984999699,7.04439163952304,4.51606202271602));
#79741=CARTESIAN_POINT('Ctrl Pts',(-6.35492962710765,6.88596068076266,4.52002922304435));
#79742=CARTESIAN_POINT('Ctrl Pts',(-6.52659755109422,6.72753143221728,4.52399638054793));
#79743=CARTESIAN_POINT('Ctrl Pts',(-6.69233235869759,6.56268467626563,4.52796353805151));
#79744=CARTESIAN_POINT('Ctrl Pts',(-6.85166523277426,6.39189084704147,4.53193069555509));
#79745=CARTESIAN_POINT('Ctrl Pts',(-7.01103240896822,6.22106024831824,4.53589870713165));
#79746=CARTESIAN_POINT('Ctrl Pts',(-7.16399470317032,6.04428022584574,4.53986671870821));
#79747=CARTESIAN_POINT('Ctrl Pts',(-7.31012155068943,5.86205663369487,4.54383473028477));
#79748=CARTESIAN_POINT('Ctrl Pts',(-7.40001388311578,5.74995879541495,4.54627571783612));
#79749=CARTESIAN_POINT('Ctrl Pts',(-7.48732024782275,5.63580162497169,4.54871670538747));
#79750=CARTESIAN_POINT('Ctrl Pts',(-7.57194811517745,5.51970894192444,4.55115769293881));
#79751=CARTESIAN_POINT('Ctrl Pts',(-7.70953013057689,5.33097364933076,4.55512607826361));
#79752=CARTESIAN_POINT('Ctrl Pts',(-7.84007340603901,5.13706263804828,4.55909446358841));
#79753=CARTESIAN_POINT('Ctrl Pts',(-7.96320136618022,4.93852296381878,4.5630628489132));
#79754=CARTESIAN_POINT('Ctrl Pts',(-8.08630782896132,4.7400179533559,4.56703054138312));
#79755=CARTESIAN_POINT('Ctrl Pts',(-8.20200141091816,4.53688613470146,4.57099823385303));
#79756=CARTESIAN_POINT('Ctrl Pts',(-8.30994956254122,4.32970245288531,4.57496592632294));
#79757=CARTESIAN_POINT('Ctrl Pts',(-8.41788599471889,4.1225412640698,4.57893318803833));
#79758=CARTESIAN_POINT('Ctrl Pts',(-8.51807854411905,3.91132934254721,4.58290044975372));
#79759=CARTESIAN_POINT('Ctrl Pts',(-8.61024075945783,3.69666594740059,4.5868677114691));
#79760=CARTESIAN_POINT('Ctrl Pts',(-8.70241018334596,3.48198576216627,4.59083528348738));
#79761=CARTESIAN_POINT('Ctrl Pts',(-8.78654790321575,3.26385382410653,4.59480285550565));
#79762=CARTESIAN_POINT('Ctrl Pts',(-8.86241526205238,3.0428902026595,4.59877042752393));
#79763=CARTESIAN_POINT('Ctrl Pts',(-8.93828182630696,2.82192889543202,4.60273795798861));
#79764=CARTESIAN_POINT('Ctrl Pts',(-9.00587811252011,2.59813623389435,4.60670548845329));
#79765=CARTESIAN_POINT('Ctrl Pts',(-9.06501485916737,2.37214895518278,4.61067301891797));
#79766=CARTESIAN_POINT('Ctrl Pts',(-9.12416432839442,2.14611305794979,4.61464140295046));
#79767=CARTESIAN_POINT('Ctrl Pts',(-9.17485054897775,1.91788187526179,4.61860978698294));
#79768=CARTESIAN_POINT('Ctrl Pts',(-9.21693474273365,1.68810515391944,4.62257817101543));
#79769=CARTESIAN_POINT('Ctrl Pts',(-9.24279766877059,1.54689540701168,4.62501694941555));
#79770=CARTESIAN_POINT('Ctrl Pts',(-9.26541282832956,1.40510218022082,4.62745572781567));
#79771=CARTESIAN_POINT('Ctrl Pts',(-9.28475763552364,1.26287794821412,4.62989450621579));
#79772=CARTESIAN_POINT('Ctrl Pts',(-9.31766281178971,1.02095703494084,4.63404282531376));
#79773=CARTESIAN_POINT('Ctrl Pts',(-9.3411101003066,0.777738127303933,4.63819114441173));
#79774=CARTESIAN_POINT('Ctrl Pts',(-9.35502482080844,0.5339435031519,4.6423394635097));
#79775=CARTESIAN_POINT('Ctrl Pts',(-9.36516671854218,0.356251098488865,
4.6453630117048));
#79776=CARTESIAN_POINT('Ctrl Pts',(-9.37024561991429,0.17825301840621,4.64838655989989));
#79777=CARTESIAN_POINT('Ctrl Pts',(-9.37024999716748,0.000230397442772201,
4.65141010809498));
#79778=CARTESIAN_POINT('Ctrl Pts',(-9.37005177233215,0.000230392568781948,
4.65141010809498));
#79779=CARTESIAN_POINT('Ctrl Pts',(-9.36899086722885,-1.12278293672488,
4.67048384522757));
#79780=CARTESIAN_POINT('Ctrl Pts',(-8.88872140496492,-3.79195700889602,
4.71580318678582));
#79781=CARTESIAN_POINT('Ctrl Pts',(-6.41096662595373,-7.36066080332452,
4.78736813276973));
#79782=CARTESIAN_POINT('Ctrl Pts',(-2.14758775427819,-9.52195991129607,
4.86610494604671));
#79783=CARTESIAN_POINT('Ctrl Pts',(2.63077110884112,-9.39994022549094,4.94484175932368));
#79784=CARTESIAN_POINT('Ctrl Pts',(6.77828505812936,-7.0238660749718,5.02357857260066));
#79785=CARTESIAN_POINT('Ctrl Pts',(9.30040197326703,-2.96350510038334,5.10231538587762));
#79786=CARTESIAN_POINT('Ctrl Pts',(9.59233161819711,1.80748833353102,5.18105219915461));
#79787=CARTESIAN_POINT('Ctrl Pts',(7.69309920158116,5.90956937174799,5.25551439243367));
#79788=CARTESIAN_POINT('Ctrl Pts',(5.44029904606853,7.73691003764319,5.30373098128708));
#79789=CARTESIAN_POINT('Ctrl Pts',(4.29107337327626,8.33032226950541,5.32570196571484));
#79790=CARTESIAN_POINT('Origin',(0.,0.,2.15141010809499));
#79791=CARTESIAN_POINT('',(4.29092662818983,8.33003803916834,6.5228999581952));
#79792=CARTESIAN_POINT('',(4.2909266281297,8.33003803919931,6.32526713834515));
#79793=CARTESIAN_POINT('',(4.29092662815669,8.33003803918541,2.15141010809499));
#79794=CARTESIAN_POINT('Ctrl Pts',(4.29092662818983,8.33003803916834,6.5228999581952));
#79795=CARTESIAN_POINT('Ctrl Pts',(4.29797836970654,8.32640558211273,6.52276053773968));
#79796=CARTESIAN_POINT('Ctrl Pts',(4.30502553725844,8.32276415076952,6.52262110685617));
#79797=CARTESIAN_POINT('Ctrl Pts',(4.47939483293704,8.23238285509755,6.51916868615752));
#79798=CARTESIAN_POINT('Ctrl Pts',(4.64406688057744,8.14062334548274,6.51585119351331));
#79799=CARTESIAN_POINT('Ctrl Pts',(4.85195946814674,8.01641803857893,6.51162498623148));
#79800=CARTESIAN_POINT('Ctrl Pts',(4.89782183385779,7.98847983939348,6.51069028967824));
#79801=CARTESIAN_POINT('Ctrl Pts',(5.00742201422516,7.92041552435395,6.50845285726873));
#79802=CARTESIAN_POINT('Ctrl Pts',(5.07092125250739,7.8799121187666,6.50715347214246));
#79803=CARTESIAN_POINT('Ctrl Pts',(5.17058929057112,7.8146344968257,6.50511305185087));
#79804=CARTESIAN_POINT('Ctrl Pts',(5.20708436143209,7.79036445920005,6.50436575312504));
#79805=CARTESIAN_POINT('Ctrl Pts',(5.28436655602216,7.73818438394952,6.50278388491557));
#79806=CARTESIAN_POINT('Ctrl Pts',(5.32510580567832,7.71020593959584,6.50195019760504));
#79807=CARTESIAN_POINT('Ctrl Pts',(5.45625696894976,7.61860009271787,6.49926387070566));
#79808=CARTESIAN_POINT('Ctrl Pts',(5.54576482713954,7.55369446553352,6.49742661690263));
#79809=CARTESIAN_POINT('Ctrl Pts',(5.82822047147332,7.34114771683431,6.49158496139705));
#79810=CARTESIAN_POINT('Ctrl Pts',(6.01658374320558,7.1875812426981,6.48761995136545));
#79811=CARTESIAN_POINT('Ctrl Pts',(6.37565826412705,6.87082293595608,6.47975956464935));
#79812=CARTESIAN_POINT('Ctrl Pts',(6.54659443707317,6.70815376287564,6.47586829353886));
#79813=CARTESIAN_POINT('Ctrl Pts',(6.77698558293327,6.47170263741448,6.47034476269931));
#79814=CARTESIAN_POINT('Ctrl Pts',(6.84173918542697,6.40320806179622,6.46875964211212));
#79815=CARTESIAN_POINT('Ctrl Pts',(6.9588298524724,6.27554849879587,6.46582967635094));
#79816=CARTESIAN_POINT('Ctrl Pts',(7.01147339696298,6.21667617351406,6.46448766695632));
#79817=CARTESIAN_POINT('Ctrl Pts',(7.12910111627834,6.0817357737788,6.46143133272535));
#79818=CARTESIAN_POINT('Ctrl Pts',(7.19362390436604,6.00527832861569,6.45971334397219));
#79819=CARTESIAN_POINT('Ctrl Pts',(7.45659510795616,5.68334480834854,6.45253620193066));
#79820=CARTESIAN_POINT('Ctrl Pts',(7.64379975319975,5.42895409634451,6.44699132615086));
#79821=CARTESIAN_POINT('Ctrl Pts',(7.90556553848391,5.03278848210838,6.43864347000669));
#79822=CARTESIAN_POINT('Ctrl Pts',(7.98992439449997,4.89775812708453,6.43584667517733));
#79823=CARTESIAN_POINT('Ctrl Pts',(8.10723019040145,4.69888759006388,6.43182325388195));
#79824=CARTESIAN_POINT('Ctrl Pts',(8.1429480494839,4.6367146814176,6.43057866774914));
#79825=CARTESIAN_POINT('Ctrl Pts',(8.2066495018906,4.52282497540583,6.42832650363028));
#79826=CARTESIAN_POINT('Ctrl Pts',(8.2348666078045,4.47124297917986,6.42731664269658));
#79827=CARTESIAN_POINT('Ctrl Pts',(8.28052529076429,4.3858785913627,6.42566410413058));
#79828=CARTESIAN_POINT('Ctrl Pts',(8.29824998887332,4.35224967583713,6.42501791034206));
#79829=CARTESIAN_POINT('Ctrl Pts',(8.34098544902496,4.26995788076397,6.42344839470047));
#79830=CARTESIAN_POINT('Ctrl Pts',(8.36577553788806,4.22118208945593,6.42252783638855));
#79831=CARTESIAN_POINT('Ctrl Pts',(8.4637719890552,4.024114535551,6.41884232653913));
#79832=CARTESIAN_POINT('Ctrl Pts',(8.53347413533364,3.87411326280363,6.41611299551519));
#79833=CARTESIAN_POINT('Ctrl Pts',(8.70502288045284,3.47781025192313,6.40901655426777));
#79834=CARTESIAN_POINT('Ctrl Pts',(8.80039658885993,3.22887092662536,6.40466878052362));
#79835=CARTESIAN_POINT('Ctrl Pts',(8.92263273869552,2.8639526516323,6.39831646930224));
#79836=CARTESIAN_POINT('Ctrl Pts',(8.95810338300139,2.75099681531146,6.39635365658527));
#79837=CARTESIAN_POINT('Ctrl Pts',(9.02035773920073,2.53875921789903,6.39266260587086));
#79838=CARTESIAN_POINT('Ctrl Pts',(9.04766606901024,2.43964971760152,6.39093779054136));
#79839=CARTESIAN_POINT('Ctrl Pts',(9.09307541141424,2.26358358695376,6.38786788633506));
#79840=CARTESIAN_POINT('Ctrl Pts',(9.11184368551238,2.18680948184148,6.38652733855971));
#79841=CARTESIAN_POINT('Ctrl Pts',(9.15069325699719,2.01869813387108,6.38358673408461));
#79842=CARTESIAN_POINT('Ctrl Pts',(9.17038300423659,1.92727910274634,6.3819842738755));
#79843=CARTESIAN_POINT('Ctrl Pts',(9.26833835446695,1.43692618078032,6.37337066577344));
#79844=CARTESIAN_POINT('Ctrl Pts',(9.32194726066565,1.03351261863197,6.36619798043127));
#79845=CARTESIAN_POINT('Ctrl Pts',(9.36056632967618,0.458489235388605,6.35608538475653));
#79846=CARTESIAN_POINT('Ctrl Pts',(9.3673373467023,0.288800448365255,6.35311809429535));
#79847=CARTESIAN_POINT('Ctrl Pts',(9.37019690329816,0.0636928941325103,
6.34923783549445));
#79848=CARTESIAN_POINT('Ctrl Pts',(9.37040964598114,0.00835923589021939,
6.34828858091579));
#79849=CARTESIAN_POINT('Ctrl Pts',(9.36992018507858,-0.0892777163247355,
6.34662348338829));
#79850=CARTESIAN_POINT('Ctrl Pts',(9.36942161718815,-0.131580195257945,
6.34590549206801));
#79851=CARTESIAN_POINT('Ctrl Pts',(9.36766138818819,-0.22642220979244,6.3443029237654));
#79852=CARTESIAN_POINT('Ctrl Pts',(9.3662441640581,-0.278957300985878,6.34341999739258));
#79853=CARTESIAN_POINT('Ctrl Pts',(9.35365790987852,-0.634524243101665,
6.3374689104538));
#79854=CARTESIAN_POINT('Ctrl Pts',(9.32822644121875,-0.936872642381898,
6.33252414150284));
#79855=CARTESIAN_POINT('Ctrl Pts',(9.26487977208946,-1.41234446645252,6.32465700099598));
#79856=CARTESIAN_POINT('Ctrl Pts',(9.23664464906192,-1.586540119386,6.32175652438732));
#79857=CARTESIAN_POINT('Ctrl Pts',(9.17854881997311,-1.89036728723269,6.31662717101886));
#79858=CARTESIAN_POINT('Ctrl Pts',(9.1508150188378,-2.02035424545892,6.31440994942017));
#79859=CARTESIAN_POINT('Ctrl Pts',(9.10133451121557,-2.23027976250025,6.3107829131888));
#79860=CARTESIAN_POINT('Ctrl Pts',(9.08127624989633,-2.31059718232633,6.30938415407222));
#79861=CARTESIAN_POINT('Ctrl Pts',(9.03891947307997,-2.47112294977449,6.30656478489693));
#79862=CARTESIAN_POINT('Ctrl Pts',(9.01661103990227,-2.5513210674882,6.30514422179718));
#79863=CARTESIAN_POINT('Ctrl Pts',(8.9550483655426,-2.76173660934026,6.30138462669632));
#79864=CARTESIAN_POINT('Ctrl Pts',(8.91402267510996,-2.89141486447328,6.29903438682642));
#79865=CARTESIAN_POINT('Ctrl Pts',(8.76511594765119,-3.3287537872509,6.2910003379743));
#79866=CARTESIAN_POINT('Ctrl Pts',(8.64400983001463,-3.63165970240849,6.28524440192507));
#79867=CARTESIAN_POINT('Ctrl Pts',(8.44161305504887,-4.07005668263084,6.276778427748));
#79868=CARTESIAN_POINT('Ctrl Pts',(8.37229436885112,-4.21080510197038,6.27404042195399));
#79869=CARTESIAN_POINT('Ctrl Pts',(8.27422225465868,-4.3979302471218,6.27040042071508));
#79870=CARTESIAN_POINT('Ctrl Pts',(8.24855035923976,-4.44589264010016,6.26946750886459));
#79871=CARTESIAN_POINT('Ctrl Pts',(8.20212052503937,-4.53085015952079,6.26781689374751));
#79872=CARTESIAN_POINT('Ctrl Pts',(8.18152636757493,-4.56793285560849,6.26709723844419));
#79873=CARTESIAN_POINT('Ctrl Pts',(8.13436536245574,-4.65151079431682,6.26547645212584));
#79874=CARTESIAN_POINT('Ctrl Pts',(8.10765032454756,-4.69792068375847,6.26457714179801));
#79875=CARTESIAN_POINT('Ctrl Pts',(7.92364234787666,-5.01133817118041,6.25850057302204));
#79876=CARTESIAN_POINT('Ctrl Pts',(7.7535845761446,-5.27063053081631,6.25345045743045));
#79877=CARTESIAN_POINT('Ctrl Pts',(7.42230898386911,-5.72490979123455,6.24422680341853));
#79878=CARTESIAN_POINT('Ctrl Pts',(7.26545059468403,-5.92270967411836,6.24006968033552));
#79879=CARTESIAN_POINT('Ctrl Pts',(7.03871309445834,-6.18604539636911,6.23425738695618));
#79880=CARTESIAN_POINT('Ctrl Pts',(6.97553083379545,-6.25720458376089,6.2326575134944));
#79881=CARTESIAN_POINT('Ctrl Pts',(6.85798355628047,-6.38559903867024,6.2297138089068));
#79882=CARTESIAN_POINT('Ctrl Pts',(6.80395806979736,-6.44313340632123,6.22837299684091));
#79883=CARTESIAN_POINT('Ctrl Pts',(6.67942499876343,-6.5724415504481,6.22530858688787));
#79884=CARTESIAN_POINT('Ctrl Pts',(6.60847534566374,-6.64377601865944,6.223581199562));
#79885=CARTESIAN_POINT('Ctrl Pts',(6.29810138241555,-6.94594156012155,6.21610323311482));
#79886=CARTESIAN_POINT('Ctrl Pts',(6.04763116742202,-7.165077850579,6.21025558557988));
#79887=CARTESIAN_POINT('Ctrl Pts',(5.62686625070864,-7.49539284920534,6.20085307228581));
#79888=CARTESIAN_POINT('Ctrl Pts',(5.46368154606181,-7.61516395416045,6.19730176973065));
#79889=CARTESIAN_POINT('Ctrl Pts',(5.24316996232073,-7.76627144920301,6.19267881502676));
#79890=CARTESIAN_POINT('Ctrl Pts',(5.18921263392935,-7.80242755461016,6.19156114438331));
#79891=CARTESIAN_POINT('Ctrl Pts',(5.09936073018297,-7.86129179410294,6.18972490364699));
#79892=CARTESIAN_POINT('Ctrl Pts',(5.06367996591732,-7.88432202222585,6.18900221662726));
#79893=CARTESIAN_POINT('Ctrl Pts',(4.98222752880574,-7.9361146713629,6.18736758330726));
#79894=CARTESIAN_POINT('Ctrl Pts',(4.9363611414305,-7.96472510040765,6.18645757473401));
#79895=CARTESIAN_POINT('Ctrl Pts',(4.77906301488812,-8.06096345532177,6.18336800656867));
#79896=CARTESIAN_POINT('Ctrl Pts',(4.66646870967089,-8.12666260381104,6.18120937408592));
#79897=CARTESIAN_POINT('Ctrl Pts',(4.34465584543885,-8.30554753097073,6.17514298835352));
#79898=CARTESIAN_POINT('Ctrl Pts',(4.13244691829045,-8.41314667080247,6.17126130703369));
#79899=CARTESIAN_POINT('Ctrl Pts',(3.78197144090259,-8.57439005388915,6.16492046631412));
#79900=CARTESIAN_POINT('Ctrl Pts',(3.64612306664921,-8.63303302623325,6.16247964835117));
#79901=CARTESIAN_POINT('Ctrl Pts',(3.39853799328566,-8.73302365249722,6.15804064072109));
#79902=CARTESIAN_POINT('Ctrl Pts',(3.28729281796078,-8.77550388492159,6.15604953240927));
#79903=CARTESIAN_POINT('Ctrl Pts',(3.0992567467844,-8.8432301798998,6.15268339896144));
#79904=CARTESIAN_POINT('Ctrl Pts',(3.02289414871753,-8.86962362939408,6.15131627246433));
#79905=CARTESIAN_POINT('Ctrl Pts',(2.86437967720139,-8.9221266022952,6.14847682098003));
#79906=CARTESIAN_POINT('Ctrl Pts',(2.78218956367326,-8.94809673789507,6.14700370183043));
#79907=CARTESIAN_POINT('Ctrl Pts',(2.54985574724562,-9.01799817913463,6.14283650197007));
#79908=CARTESIAN_POINT('Ctrl Pts',(2.39895380235328,-9.05930879884373,6.14012602362838));
#79909=CARTESIAN_POINT('Ctrl Pts',(1.94294509942392,-9.17195166287925,6.13193426643136));
#79910=CARTESIAN_POINT('Ctrl Pts',(1.63522489843687,-9.23178052515135,6.12639920138766));
#79911=CARTESIAN_POINT('Ctrl Pts',(1.25640516750639,-9.28589494026231,6.11969931301949));
#79912=CARTESIAN_POINT('Ctrl Pts',(1.18761448160606,-9.29494328376726,6.11848757379081));
#79913=CARTESIAN_POINT('Ctrl Pts',(1.03015114826317,-9.31387853026773,6.1157289574021));
#79914=CARTESIAN_POINT('Ctrl Pts',(0.941424887848997,-9.32326465939015,
6.11418542965282));
#79915=CARTESIAN_POINT('Ctrl Pts',(0.806637048814814,-9.33557978508224,
6.11186328709341));
#79916=CARTESIAN_POINT('Ctrl Pts',(0.760665659336862,-9.33943793913225,
6.11107528946117));
#79917=CARTESIAN_POINT('Ctrl Pts',(0.668656956501475,-9.34647592960889,
6.10950741242211));
#79918=CARTESIAN_POINT('Ctrl Pts',(0.62262087780027,-9.34965548471017,6.10872755630882));
#79919=CARTESIAN_POINT('Ctrl Pts',(0.487440543333029,-9.35798908965392,
6.10644885548497));
#79920=CARTESIAN_POINT('Ctrl Pts',(0.39824377356692,-9.36220914353442,6.10495962525912));
#79921=CARTESIAN_POINT('Ctrl Pts',(-0.0331035061062979,-9.37644130616774,
6.0978015585962));
#79922=CARTESIAN_POINT('Ctrl Pts',(-0.375569396244216,-9.36897520793617,
6.09224150176936));
#79923=CARTESIAN_POINT('Ctrl Pts',(-0.845687809321002,-9.33290372724416,
6.08447323246501));
#79924=CARTESIAN_POINT('Ctrl Pts',(-0.974299004435995,-9.32035520804936,
6.0823352537515));
#79925=CARTESIAN_POINT('Ctrl Pts',(-1.2108281733077,-9.2923278010977,6.07836669457467));
#79926=CARTESIAN_POINT('Ctrl Pts',(-1.31881490934292,-9.27761758119378,
6.07654075023429));
#79927=CARTESIAN_POINT('Ctrl Pts',(-1.50514886545598,-9.24891567160424,
6.07336097741795));
#79928=CARTESIAN_POINT('Ctrl Pts',(-1.58361990668614,-9.23580327662374,
6.07201293080726));
#79929=CARTESIAN_POINT('Ctrl Pts',(-1.75042590141695,-9.20574184790195,
6.06912712952669));
#79930=CARTESIAN_POINT('Ctrl Pts',(-1.83870307526634,-9.18851700538763,
6.06758771273284));
#79931=CARTESIAN_POINT('Ctrl Pts',(-2.10897489767909,-9.13173005448163,
6.06283659647974));
#79932=CARTESIAN_POINT('Ctrl Pts',(-2.29004861689295,-9.08801110613602,
6.05959949585475));
#79933=CARTESIAN_POINT('Ctrl Pts',(-2.73735902819464,-8.96579283545478,
6.05148702746107));
#79934=CARTESIAN_POINT('Ctrl Pts',(-3.00163855594821,-8.88080746592874,
6.04658743583834));
#79935=CARTESIAN_POINT('Ctrl Pts',(-3.38593459776506,-8.73811068617633,
6.03941460946368));
#79936=CARTESIAN_POINT('Ctrl Pts',(-3.50912161481898,-8.68937265396421,
6.03710864202932));
#79937=CARTESIAN_POINT('Ctrl Pts',(-3.67928076784952,-8.61784163956654,
6.03393157693828));
#79938=CARTESIAN_POINT('Ctrl Pts',(-3.72715816494055,-8.59724336768051,
6.03303859831938));
#79939=CARTESIAN_POINT('Ctrl Pts',(-3.81409027490409,-8.55897993295781,
6.03142053305565));
#79940=CARTESIAN_POINT('Ctrl Pts',(-3.85320026453933,-8.54144424774349,
6.03069399017489));
#79941=CARTESIAN_POINT('Ctrl Pts',(-3.95450570122614,-8.49518468852865,
6.02881462164188));
#79942=CARTESIAN_POINT('Ctrl Pts',(-4.01650896232153,-8.46604594965714,
6.02766673834312));
#79943=CARTESIAN_POINT('Ctrl Pts',(-4.24400346178812,-8.356072043054,6.0234548202241));
#79944=CARTESIAN_POINT('Ctrl Pts',(-4.40742086466586,-8.27104268183566,
6.02042803844561));
#79945=CARTESIAN_POINT('Ctrl Pts',(-4.65862540963312,-8.1307757476858,6.01570927403594));
#79946=CARTESIAN_POINT('Ctrl Pts',(-4.74818167273247,-8.07880410522671,
6.01401360517946));
#79947=CARTESIAN_POINT('Ctrl Pts',(-5.05541858156953,-7.89363340305294,
6.00812922588155));
#79948=CARTESIAN_POINT('Ctrl Pts',(-5.26850614530403,-7.75303474666433,
6.00392624755133));
#79949=CARTESIAN_POINT('Ctrl Pts',(-5.55291261219695,-7.54823330863531,
5.99806447957599));
#79950=CARTESIAN_POINT('Ctrl Pts',(-5.62938311193821,-7.49137572701669,
5.99646247084077));
#79951=CARTESIAN_POINT('Ctrl Pts',(-5.76757545985104,-7.38531555798363,
5.99351675087762));
#79952=CARTESIAN_POINT('Ctrl Pts',(-5.82956837730591,-7.33648042842947,
5.99217608511301));
#79953=CARTESIAN_POINT('Ctrl Pts',(-5.96904774795024,-7.22372085032136,
5.98911461852156));
#79954=CARTESIAN_POINT('Ctrl Pts',(-6.04613801525816,-7.15932182358294,
5.98739005921991));
#79955=CARTESIAN_POINT('Ctrl Pts',(-6.37509514466811,-6.87541706319275,
5.97988897899086));
#79956=CARTESIAN_POINT('Ctrl Pts',(-6.61615684437095,-6.64376885822131,
5.97401424475727));
#79957=CARTESIAN_POINT('Ctrl Pts',(-6.94578318227007,-6.29124361292791,
5.96553126290414));
#79958=CARTESIAN_POINT('Ctrl Pts',(-7.04464193042249,-6.18034549131344,
5.96292373882137));
#79959=CARTESIAN_POINT('Ctrl Pts',(-7.20284675540514,-5.99414378659714,
5.95866883074758));
#79960=CARTESIAN_POINT('Ctrl Pts',(-7.26374801988948,-5.92019644062888,
5.95700966611933));
#79961=CARTESIAN_POINT('Ctrl Pts',(-7.35295932851441,-5.80842522315705,
5.95455446022486));
#79962=CARTESIAN_POINT('Ctrl Pts',(-7.3821345084353,-5.77130007640062,5.95374742496283));
#79963=CARTESIAN_POINT('Ctrl Pts',(-7.43525214507516,-5.70264655188049,
5.95227171676185));
#79964=CARTESIAN_POINT('Ctrl Pts',(-7.45927777044506,-5.67118394184633,
5.95160182563131));
#79965=CARTESIAN_POINT('Ctrl Pts',(-7.52861826158614,-5.57917656238893,
5.94965995209038));
#79966=CARTESIAN_POINT('Ctrl Pts',(-7.57340051885043,-5.51823419822869,
5.94839505712186));
#79967=CARTESIAN_POINT('Ctrl Pts',(-7.82736911044628,-5.1637029629282,5.94113963924782));
#79968=CARTESIAN_POINT('Ctrl Pts',(-8.02021247361393,-4.85877858788658,
5.93528986976471));
#79969=CARTESIAN_POINT('Ctrl Pts',(-8.2586217050041,-4.42876550521456,5.9271915306902));
#79970=CARTESIAN_POINT('Ctrl Pts',(-8.31981803805225,-4.31270496076447,
5.92502147048924));
#79971=CARTESIAN_POINT('Ctrl Pts',(-8.42784465491668,-4.09696686404027,
5.92100249862582));
#79972=CARTESIAN_POINT('Ctrl Pts',(-8.47539365344757,-3.99767499291938,
5.91915846108813));
#79973=CARTESIAN_POINT('Ctrl Pts',(-8.55432243203215,-3.82511446594908,
5.91595859966093));
#79974=CARTESIAN_POINT('Ctrl Pts',(-8.58653729177827,-3.7522406974054,5.91460878320093));
#79975=CARTESIAN_POINT('Ctrl Pts',(-8.65292864388995,-3.59672178566555,
5.91173017171816));
#79976=CARTESIAN_POINT('Ctrl Pts',(-8.68685929488228,-3.5139802592186,5.91019982629159));
#79977=CARTESIAN_POINT('Ctrl Pts',(-8.7861365804028,-3.26165810067457,5.90553606838316));
#79978=CARTESIAN_POINT('Ctrl Pts',(-8.84773900544608,-3.09065101830168,
5.9023787313846));
#79979=CARTESIAN_POINT('Ctrl Pts',(-8.92143575200027,-2.86576110103158,
5.89824015406613));
#79980=CARTESIAN_POINT('Ctrl Pts',(-8.93808253384746,-2.813411306161,5.89727780029478));
#79981=CARTESIAN_POINT('Ctrl Pts',(-9.02492128230767,-2.53177404848862,
5.8921080068485));
#79982=CARTESIAN_POINT('Ctrl Pts',(-9.08675259832259,-2.30000242308958,
5.88787790850983));
#79983=CARTESIAN_POINT('Ctrl Pts',(-9.15313115094227,-2.00637157004691,
5.88261507124184));
#79984=CARTESIAN_POINT('Ctrl Pts',(-9.16605072242308,-1.94649708756365,
5.88154704021331));
#79985=CARTESIAN_POINT('Ctrl Pts',(-9.18634564342182,-1.84775628457683,
5.8797960962851));
#79986=CARTESIAN_POINT('Ctrl Pts',(-9.19406357114437,-1.80896230547793,
5.87911080001503));
#79987=CARTESIAN_POINT('Ctrl Pts',(-9.21305141692628,-1.71025866895324,
5.87737475558814));
#79988=CARTESIAN_POINT('Ctrl Pts',(-9.22398277836167,-1.65028568873828,
5.87632697283346));
#79989=CARTESIAN_POINT('Ctrl Pts',(-9.2414876487661,-1.54863515568507,5.87456528383404));
#79990=CARTESIAN_POINT('Ctrl Pts',(-9.24836627933908,-1.50701227075214,
5.87384806991923));
#79991=CARTESIAN_POINT('Ctrl Pts',(-9.26370188605477,-1.41015414784513,
5.87218878995313));
#79992=CARTESIAN_POINT('Ctrl Pts',(-9.27194631986713,-1.35488701197608,
5.87124905520164));
#79993=CARTESIAN_POINT('Ctrl Pts',(-9.30470506315215,-1.12096655920038,
5.86729561230279));
#79994=CARTESIAN_POINT('Ctrl Pts',(-9.3245539718842,-0.941698441403416,
5.86432427290705));
#79995=CARTESIAN_POINT('Ctrl Pts',(-9.35989205572344,-0.50857055636118,
5.85718944343998));
#79996=CARTESIAN_POINT('Ctrl Pts',(-9.37024469947905,-0.254435793981661,
5.85303770209661));
#79997=CARTESIAN_POINT('Ctrl Pts',(-9.37025337653925,0.161920866284036,
5.84616237230288));
#79998=CARTESIAN_POINT('Ctrl Pts',(-9.36604956202626,0.32400939424748,5.84346835364772));
#79999=CARTESIAN_POINT('Ctrl Pts',(-9.35313306729956,0.572756601392295,
5.83928903134108));
#80000=CARTESIAN_POINT('Ctrl Pts',(-9.34741440879344,0.659539328381405,
5.83782263723035));
#80001=CARTESIAN_POINT('Ctrl Pts',(-9.33408152616977,0.826425788163054,
5.83498477956949));
#80002=CARTESIAN_POINT('Ctrl Pts',(-9.3266419559059,0.906535885206288,5.83361455810884));
#80003=CARTESIAN_POINT('Ctrl Pts',(-9.30590426327884,1.10240970446815,5.83024393264564));
#80004=CARTESIAN_POINT('Ctrl Pts',(-9.29147670765068,1.21804014813801,5.8282366022995));
#80005=CARTESIAN_POINT('Ctrl Pts',(-9.25453854669684,1.47498107085413,5.82373830076327));
#80006=CARTESIAN_POINT('Ctrl Pts',(-9.23094006979387,1.61610586103673,5.82124181962598));
#80007=CARTESIAN_POINT('Ctrl Pts',(-9.15982028755866,1.98874737800959,5.81459446969821));
#80008=CARTESIAN_POINT('Ctrl Pts',(-9.10675651189692,2.21910106209131,5.81042655133858));
#80009=CARTESIAN_POINT('Ctrl Pts',(-9.00820080604955,2.58337036682101,5.80381665043818));
#80010=CARTESIAN_POINT('Ctrl Pts',(-8.96828910552953,2.71868992655045,5.80135750874224));
#80011=CARTESIAN_POINT('Ctrl Pts',(-8.90874957789901,2.90494992414661,5.79798828779435));
#80012=CARTESIAN_POINT('Ctrl Pts',(-8.89170929156123,2.95669731222532,5.79705397262397));
#80013=CARTESIAN_POINT('Ctrl Pts',(-8.86060430044073,3.04845448913544,5.79540213715716));
#80014=CARTESIAN_POINT('Ctrl Pts',(-8.84671749096731,3.08852278247073,5.79468264775012));
#80015=CARTESIAN_POINT('Ctrl Pts',(-8.81109853745735,3.18908438125109,5.79288080152028));
#80016=CARTESIAN_POINT('Ctrl Pts',(-8.78901504353268,3.2494509105338,5.79180251080762));
#80017=CARTESIAN_POINT('Ctrl Pts',(-8.75124199561557,3.34950281330605,5.79001754411294));
#80018=CARTESIAN_POINT('Ctrl Pts',(-8.73589935815571,3.38931674125589,5.78930783492399));
#80019=CARTESIAN_POINT('Ctrl Pts',(-8.62482910979277,3.67177732170096,5.78427297957588));
#80020=CARTESIAN_POINT('Ctrl Pts',(-8.519277803058,3.91043888348666,5.7800164718201));
#80021=CARTESIAN_POINT('Ctrl Pts',(-8.29622964708334,4.36273173068542,5.77174222042305));
#80022=CARTESIAN_POINT('Ctrl Pts',(-8.18008400091835,4.57679798033519,5.7677308151304));
#80023=CARTESIAN_POINT('Ctrl Pts',(-8.00632577414337,4.86925968558907,5.76204374878382));
#80024=CARTESIAN_POINT('Ctrl Pts',(-7.95563229643581,4.95165194586734,5.76041810259866));
#80025=CARTESIAN_POINT('Ctrl Pts',(-7.86130708763694,5.09977023372098,5.75744966370739));
#80026=CARTESIAN_POINT('Ctrl Pts',(-7.81810368657875,5.16575844142914,5.75611020708584));
#80027=CARTESIAN_POINT('Ctrl Pts',(-7.71892638309235,5.31314575875241,5.7530789228856));
#80028=CARTESIAN_POINT('Ctrl Pts',(-7.66248799979673,5.39422097711547,5.7513836579507));
#80029=CARTESIAN_POINT('Ctrl Pts',(-7.5396056171217,5.56492374772573,5.74775451231939));
#80030=CARTESIAN_POINT('Ctrl Pts',(-7.47282137830764,5.65428773124383,5.74581838759129));
#80031=CARTESIAN_POINT('Ctrl Pts',(-7.26299883473211,5.92483870400857,5.73984878710464));
#80032=CARTESIAN_POINT('Ctrl Pts',(-7.1148486581083,6.10195001087115,5.73578644039121));
#80033=CARTESIAN_POINT('Ctrl Pts',(-6.94012615383007,6.29580359824902,5.73119970603883));
#80034=CARTESIAN_POINT('Ctrl Pts',(-6.91983385748313,6.31810045536646,5.73066999538527));
#80035=CARTESIAN_POINT('Ctrl Pts',(-6.77448107054488,6.47627154568714,5.72689771971454));
#80036=CARTESIAN_POINT('Ctrl Pts',(-6.6455352368933,6.60852091175285,5.72366571988583));
#80037=CARTESIAN_POINT('Ctrl Pts',(-6.4723246343232,6.77596951443039,5.71951081612198));
#80038=CARTESIAN_POINT('Ctrl Pts',(-6.43153220993575,6.81470046919124,5.71854526454732));
#80039=CARTESIAN_POINT('Ctrl Pts',(-6.35955184330272,6.88182125059916,5.71686589235061));
#80040=CARTESIAN_POINT('Ctrl Pts',(-6.32851653348345,6.91037204968196,5.71614972884859));
#80041=CARTESIAN_POINT('Ctrl Pts',(-6.25248567924997,6.9793745180606,5.71441409449984));
#80042=CARTESIAN_POINT('Ctrl Pts',(-6.20728911051949,7.01960168064195,5.71339791475549));
#80043=CARTESIAN_POINT('Ctrl Pts',(-6.13222377202788,7.085121599341,5.71173277944348));
#80044=CARTESIAN_POINT('Ctrl Pts',(-6.10258055835842,7.11066994041068,5.71108091403971));
#80045=CARTESIAN_POINT('Ctrl Pts',(-6.02684683139344,7.17511950169752,5.70942877853367));
#80046=CARTESIAN_POINT('Ctrl Pts',(-5.98053915367905,7.21376282102248,5.70843091286447));
#80047=CARTESIAN_POINT('Ctrl Pts',(-5.75377046770128,7.39931468068321,5.70359646046525));
#80048=CARTESIAN_POINT('Ctrl Pts',(-5.56825253617325,7.53991354848985,5.69979769622794));
#80049=CARTESIAN_POINT('Ctrl Pts',(-5.32336961606374,7.71153172122506,5.69488759623671));
#80050=CARTESIAN_POINT('Ctrl Pts',(-5.26864300773012,7.74902486802278,5.69379687088433));
#80051=CARTESIAN_POINT('Ctrl Pts',(-5.06542434549197,7.88510169512479,5.68976623371663));
#80052=CARTESIAN_POINT('Ctrl Pts',(-4.91452683398795,7.98002370086844,5.68681070606336));
#80053=CARTESIAN_POINT('Ctrl Pts',(-4.68363054104729,8.11623448779535,5.68231818233365));
#80054=CARTESIAN_POINT('Ctrl Pts',(-4.6055941483689,8.16076955922156,5.68080496026396));
#80055=CARTESIAN_POINT('Ctrl Pts',(-4.45725626679338,8.24261997046261,5.67793589359257));
#80056=CARTESIAN_POINT('Ctrl Pts',(-4.38709623516137,8.28017536011301,5.67658195657102));
#80057=CARTESIAN_POINT('Ctrl Pts',(-4.21957067892398,8.36712173638765,5.67335540794998));
#80058=CARTESIAN_POINT('Ctrl Pts',(-4.12180364422911,8.4157137248719,5.67147734535286));
#80059=CARTESIAN_POINT('Ctrl Pts',(-3.78534652021014,8.57566928264624,5.66503193458509));
#80060=CARTESIAN_POINT('Ctrl Pts',(-3.54282168133793,8.67867303179076,5.66041269444136));
#80061=CARTESIAN_POINT('Ctrl Pts',(-3.05760085682517,8.86102004005712,5.65129975405944));
#80062=CARTESIAN_POINT('Ctrl Pts',(-2.81535784850433,8.94093729681579,5.64681101242222));
#80063=CARTESIAN_POINT('Ctrl Pts',(-2.50988256764019,9.02806752346637,5.64132137755137));
#80064=CARTESIAN_POINT('Ctrl Pts',(-2.44943644833561,9.04465448888287,5.64024347965621));
#80065=CARTESIAN_POINT('Ctrl Pts',(-2.34794387842794,9.07141291855236,5.63845009821669));
#80066=CARTESIAN_POINT('Ctrl Pts',(-2.30698692145097,9.08191522506695,5.63773095817806));
#80067=CARTESIAN_POINT('Ctrl Pts',(-2.21203624626077,9.10557900923839,5.63607457769256));
#80068=CARTESIAN_POINT('Ctrl Pts',(-2.15799384139358,9.11853804334601,5.6351396001533));
#80069=CARTESIAN_POINT('Ctrl Pts',(-1.93469469456448,9.16998747010512,5.63130281407443));
#80070=CARTESIAN_POINT('Ctrl Pts',(-1.76449932718783,9.20425207409953,5.62844039362714));
#80071=CARTESIAN_POINT('Ctrl Pts',(-1.19802870119357,9.30200660162239,5.61899845871164));
#80072=CARTESIAN_POINT('Ctrl Pts',(-0.798633312236216,9.34477310776482,
5.61246080334827));
#80073=CARTESIAN_POINT('Ctrl Pts',(-0.304015341916333,9.36578655495732,
5.60417653922342));
#80074=CARTESIAN_POINT('Ctrl Pts',(-0.210247573615239,9.36836053027925,
5.6025988438428));
#80075=CARTESIAN_POINT('Ctrl Pts',(-0.0374557112724693,9.37050822109672,
5.59967566187743));
#80076=CARTESIAN_POINT('Ctrl Pts',(0.0415548547491671,9.3704909376299,5.59833291818088));
#80077=CARTESIAN_POINT('Ctrl Pts',(0.22293590423829,9.36815713473454,5.5952355165982));
#80078=CARTESIAN_POINT('Ctrl Pts',(0.325287513047653,9.36516185023385,5.59347672545005));
#80079=CARTESIAN_POINT('Ctrl Pts',(0.489479198022377,9.35766188821574,5.59063788466171));
#80080=CARTESIAN_POINT('Ctrl Pts',(0.551359490608713,9.35421982837435,5.58956403485926));
#80081=CARTESIAN_POINT('Ctrl Pts',(0.785724603006797,9.33884973187025,5.58548282153041));
#80082=CARTESIAN_POINT('Ctrl Pts',(0.957901646960043,9.32276255626564,5.5824548761334));
#80083=CARTESIAN_POINT('Ctrl Pts',(1.19745369199001,9.29367369569156,5.57821609179894));
#80084=CARTESIAN_POINT('Ctrl Pts',(1.26528055767802,9.28468261244795,5.57701309724961));
#80085=CARTESIAN_POINT('Ctrl Pts',(1.39967898785248,9.26536676720865,5.57462589253961));
#80086=CARTESIAN_POINT('Ctrl Pts',(1.46624987638042,9.25506531061842,5.57344174909946));
#80087=CARTESIAN_POINT('Ctrl Pts',(1.69493854922914,9.21714771648842,5.56937225193449));
#80088=CARTESIAN_POINT('Ctrl Pts',(1.85643733937426,9.1859822199621,5.56649507576767));
#80089=CARTESIAN_POINT('Ctrl Pts',(2.07811015190131,9.13711962346229,5.5625724296476));
#80090=CARTESIAN_POINT('Ctrl Pts',(2.13905173157476,9.12304524446193,5.56149689495644));
#80091=CARTESIAN_POINT('Ctrl Pts',(2.24093903202218,9.09843746414717,5.55970602659849));
#80092=CARTESIAN_POINT('Ctrl Pts',(2.28196248477532,9.08823521196743,5.55898706378743));
#80093=CARTESIAN_POINT('Ctrl Pts',(2.37684966566549,9.06395443914295,5.55732921714552));
#80094=CARTESIAN_POINT('Ctrl Pts',(2.43065964684377,9.04967281776047,5.55639261714228));
#80095=CARTESIAN_POINT('Ctrl Pts',(2.65326570889496,8.98846259871728,5.55252721304878));
#80096=CARTESIAN_POINT('Ctrl Pts',(2.82085680085678,8.93728404406734,5.54963855329337));
#80097=CARTESIAN_POINT('Ctrl Pts',(3.36514064422939,8.75423603011843,5.54020740940771));
#80098=CARTESIAN_POINT('Ctrl Pts',(3.73485381572756,8.60300453240689,5.53370493249914));
#80099=CARTESIAN_POINT('Ctrl Pts',(4.15989264231646,8.39656342359426,5.52579822219299));
#80100=CARTESIAN_POINT('Ctrl Pts',(4.22560673919744,8.36368528660159,5.52456375066252));
#80101=CARTESIAN_POINT('Ctrl Pts',(4.29092662824368,8.3300380391406,5.52332385470008));
#80102=CARTESIAN_POINT('',(-9.37096239705712,-4.07005226067136E-5,5.65143860498297));
#80103=CARTESIAN_POINT('Ctrl Pts',(4.29107337327626,8.33032226950541,5.32570196571484));
#80104=CARTESIAN_POINT('Ctrl Pts',(4.06748288923697,8.44577507507538,5.32997658571274));
#80105=CARTESIAN_POINT('Ctrl Pts',(2.43791876811844,9.20543064297083,5.3604968101363));
#80106=CARTESIAN_POINT('Ctrl Pts',(-0.970645488733943,9.71275900755431,
5.41726263898552));
#80107=CARTESIAN_POINT('Ctrl Pts',(-5.46572508632491,8.08737839383646,5.4959994522625));
#80108=CARTESIAN_POINT('Ctrl Pts',(-8.62234106295286,4.55381982533101,5.57404860769815));
#80109=CARTESIAN_POINT('Ctrl Pts',(-9.37063486116336,1.50430010234368,5.62585215870815));
#80110=CARTESIAN_POINT('Ctrl Pts',(-9.3710117781914,-4.11794517302605E-5,
5.65141010529249));
#80111=CARTESIAN_POINT('Ctrl Pts',(-9.37024999993907,-3.37912498182759E-5,
5.65184975587397));
#80112=CARTESIAN_POINT('Ctrl Pts',(-9.37024989579904,-0.0289116261349408,
5.65234466512349));
#80113=CARTESIAN_POINT('Ctrl Pts',(-9.37011629532077,-0.0577893348672783,
5.65283817878753));
#80114=CARTESIAN_POINT('Ctrl Pts',(-9.36958296607992,-0.115449952971927,
5.65382049981617));
#80115=CARTESIAN_POINT('Ctrl Pts',(-9.36918409739989,-0.144232451791148,
5.65430925987687));
#80116=CARTESIAN_POINT('Ctrl Pts',(-9.36765285470081,-0.22714934709786,
5.65571291340118));
#80117=CARTESIAN_POINT('Ctrl Pts',(-9.36618387985989,-0.28127633830779,
5.65662395395215));
#80118=CARTESIAN_POINT('Ctrl Pts',(-9.35846354684279,-0.496833177514481,
5.66023613480282));
#80119=CARTESIAN_POINT('Ctrl Pts',(-9.34850706241727,-0.658102699117982,
5.662903321492));
#80120=CARTESIAN_POINT('Ctrl Pts',(-9.31375530258424,-1.05416221238166,
5.66943839173724));
#80121=CARTESIAN_POINT('Ctrl Pts',(-9.28424756929226,-1.28842654786451,
5.67329194823512));
#80122=CARTESIAN_POINT('Ctrl Pts',(-9.21560675066315,-1.70559407591073,
5.68025348527256));
#80123=CARTESIAN_POINT('Ctrl Pts',(-9.17978558185586,-1.88891378916537,
5.68334704105314));
#80124=CARTESIAN_POINT('Ctrl Pts',(-9.12177378990983,-2.14489213035734,
5.68774328943355));
#80125=CARTESIAN_POINT('Ctrl Pts',(-9.1041422414575,-2.21853856044011,5.68901699097461));
#80126=CARTESIAN_POINT('Ctrl Pts',(-9.06632832593687,-2.36843751355314,
5.69162916419587));
#80127=CARTESIAN_POINT('Ctrl Pts',(-9.04607193855923,-2.44466521596368,
5.69296802678948));
#80128=CARTESIAN_POINT('Ctrl Pts',(-8.99883070541919,-2.6138077123164,5.69596331360591));
#80129=CARTESIAN_POINT('Ctrl Pts',(-8.97136427215402,-2.70657862575678,
5.69762278063558));
#80130=CARTESIAN_POINT('Ctrl Pts',(-8.86969277872221,-3.0314174889467,5.70349221376078));
#80131=CARTESIAN_POINT('Ctrl Pts',(-8.78787913977127,-3.2610000671582,5.70774945973942));
#80132=CARTESIAN_POINT('Ctrl Pts',(-8.60017657053575,-3.72914669000218,
5.71660729636332));
#80133=CARTESIAN_POINT('Ctrl Pts',(-8.49308173452594,-3.967005779683,5.72120741426368));
#80134=CARTESIAN_POINT('Ctrl Pts',(-8.35709812718722,-4.23819694879667,
5.7264833822988));
#80135=CARTESIAN_POINT('Ctrl Pts',(-8.3377293872886,-4.27617482744637,5.72722287248126));
#80136=CARTESIAN_POINT('Ctrl Pts',(-8.2954431205099,-4.35770934711342,5.72881092762362));
#80137=CARTESIAN_POINT('Ctrl Pts',(-8.27244021015677,-4.40122031953226,
5.72965867337914));
#80138=CARTESIAN_POINT('Ctrl Pts',(-8.23075656345284,-4.47858530181541,
5.73116524002601));
#80139=CARTESIAN_POINT('Ctrl Pts',(-8.21220706887636,-4.51250872325204,
5.73182557814925));
#80140=CARTESIAN_POINT('Ctrl Pts',(-8.1792144487369,-4.57196857993514,5.73298187667849));
#80141=CARTESIAN_POINT('Ctrl Pts',(-8.16486038344219,-4.59755376402362,
5.73347902203042));
#80142=CARTESIAN_POINT('Ctrl Pts',(-8.12032239722587,-4.6760733860798,5.73500407578025));
#80143=CARTESIAN_POINT('Ctrl Pts',(-8.08974204413658,-4.7287812203867,5.73602689665022));
#80144=CARTESIAN_POINT('Ctrl Pts',(-7.92605554652935,-5.00467340397007,
5.74138510962711));
#80145=CARTESIAN_POINT('Ctrl Pts',(-7.78422154660125,-5.22254806498498,
5.74563493653989));
#80146=CARTESIAN_POINT('Ctrl Pts',(-7.51975885549578,-5.59404027625978,
5.75310958534515));
#80147=CARTESIAN_POINT('Ctrl Pts',(-7.40101298807343,-5.75022316452486,
5.75632766516728));
#80148=CARTESIAN_POINT('Ctrl Pts',(-7.22990259146722,-5.9611904641756,5.76082578575394));
#80149=CARTESIAN_POINT('Ctrl Pts',(-7.18164520809691,-6.01924042669869,
5.76207992244942));
#80150=CARTESIAN_POINT('Ctrl Pts',(-7.11119041329583,-6.10193864436893,
5.7638922317589));
#80151=CARTESIAN_POINT('Ctrl Pts',(-7.08955530454295,-6.12706209332143,
5.76444627605989));
#80152=CARTESIAN_POINT('Ctrl Pts',(-7.01196733192476,-6.21619880240184,
5.76642472547702));
#80153=CARTESIAN_POINT('Ctrl Pts',(-6.95527721952354,-6.27956464848709,
5.76785480225397));
#80154=CARTESIAN_POINT('Ctrl Pts',(-6.84433833877763,-6.40022195420276,
5.77062600334781));
#80155=CARTESIAN_POINT('Ctrl Pts',(-6.79021280718335,-6.45761708049246,
5.7719659884356));
#80156=CARTESIAN_POINT('Ctrl Pts',(-6.66612540844515,-6.58591507542862,
5.77501210351289));
#80157=CARTESIAN_POINT('Ctrl Pts',(-6.5957447901225,-6.65639962288557,5.77672182945038));
#80158=CARTESIAN_POINT('Ctrl Pts',(-6.24064946601922,-7.00085675724952,
5.78525986158919));
#80159=CARTESIAN_POINT('Ctrl Pts',(-5.93992882897042,-7.25775057819928,
5.79223458689192));
#80160=CARTESIAN_POINT('Ctrl Pts',(-5.49241591368908,-7.59354808339555,
5.80204878857817));
#80161=CARTESIAN_POINT('Ctrl Pts',(-5.35836315436023,-7.68872873936398,
5.80491999001603));
#80162=CARTESIAN_POINT('Ctrl Pts',(-5.17623845460289,-7.81096418633117,
5.80869999228001));
#80163=CARTESIAN_POINT('Ctrl Pts',(-5.13033222445535,-7.8411923420122,5.80964278023133));
#80164=CARTESIAN_POINT('Ctrl Pts',(-5.04859240513639,-7.89399093801382,
5.81130208134062));
#80165=CARTESIAN_POINT('Ctrl Pts',(-5.01286699732228,-7.91672550188332,
5.81202066478612));
#80166=CARTESIAN_POINT('Ctrl Pts',(-4.92314657136959,-7.9729700304823,5.81380943499928));
#80167=CARTESIAN_POINT('Ctrl Pts',(-4.86896255644299,-8.00617429995087,
5.81487570446277));
#80168=CARTESIAN_POINT('Ctrl Pts',(-4.65897621502866,-8.13193492871861,
5.81896194121221));
#80169=CARTESIAN_POINT('Ctrl Pts',(-4.50083869776133,-8.22051558191104,
5.8219433426094));
#80170=CARTESIAN_POINT('Ctrl Pts',(-4.12461908357614,-8.41714262003123,
5.8289083865292));
#80171=CARTESIAN_POINT('Ctrl Pts',(-3.90469932876008,-8.52139047096103,
5.8328842860495));
#80172=CARTESIAN_POINT('Ctrl Pts',(-3.57605834438582,-8.6617785360276,5.83878805626679));
#80173=CARTESIAN_POINT('Ctrl Pts',(-3.47033427033911,-8.70467579328038,
5.84068128097275));
#80174=CARTESIAN_POINT('Ctrl Pts',(-3.27025966716364,-8.78163097126256,
5.84426111042753));
#80175=CARTESIAN_POINT('Ctrl Pts',(-3.17609418153422,-8.81612536729526,
5.84594473506969));
#80176=CARTESIAN_POINT('Ctrl Pts',(-3.00757029402036,-8.87480797823594,
5.84895903747043));
#80177=CARTESIAN_POINT('Ctrl Pts',(-2.93342854093253,-8.89958946730819,
5.85028555830016));
#80178=CARTESIAN_POINT('Ctrl Pts',(-2.76846507914372,-8.95244219328348,
5.85323889290671));
#80179=CARTESIAN_POINT('Ctrl Pts',(-2.6775087629876,-8.98006497108694,5.8548685395246));
#80180=CARTESIAN_POINT('Ctrl Pts',(-2.22586671497069,-9.10975344980545,
5.86296697387117));
#80181=CARTESIAN_POINT('Ctrl Pts',(-1.85970338242008,-9.1914955855669,5.8695683725386));
#80182=CARTESIAN_POINT('Ctrl Pts',(-1.29841769536839,-9.28187524300104,
5.87955474604179));
#80183=CARTESIAN_POINT('Ctrl Pts',(-1.10629282416263,-9.30672945098972,
5.88294659698164));
#80184=CARTESIAN_POINT('Ctrl Pts',(-0.85718651856507,-9.33113187370542,
5.88726292983199));
#80185=CARTESIAN_POINT('Ctrl Pts',(-0.800788287175399,-9.33614100746879,
5.88823470407168));
#80186=CARTESIAN_POINT('Ctrl Pts',(-0.702278390065371,-9.34399118261003,
5.88992062896209));
#80187=CARTESIAN_POINT('Ctrl Pts',(-0.660186722569009,-9.34705941217063,
5.89063719723311));
#80188=CARTESIAN_POINT('Ctrl Pts',(-0.556893519628924,-9.35388765530491,
5.89238676057105));
#80189=CARTESIAN_POINT('Ctrl Pts',(-0.49567316430912,-9.3573314999089,5.89341629746416));
#80190=CARTESIAN_POINT('Ctrl Pts',(-0.148751782971023,-9.3734327754173,
5.89921859690431));
#80191=CARTESIAN_POINT('Ctrl Pts',(0.137378082591571,-9.37360643657555,
5.90388657303226));
#80192=CARTESIAN_POINT('Ctrl Pts',(0.673437879476852,-9.34937857496442,
5.91268538258595));
#80193=CARTESIAN_POINT('Ctrl Pts',(0.923252734535412,-9.32802241842335,
5.91680711075412));
#80194=CARTESIAN_POINT('Ctrl Pts',(1.27393290959422,-9.28381678721565,5.92270552928298));
#80195=CARTESIAN_POINT('Ctrl Pts',(1.37573731508842,-9.26927753213982,5.92443090862054));
#80196=CARTESIAN_POINT('Ctrl Pts',(1.55532738118887,-9.24060540239003,5.92750141527083));
#80197=CARTESIAN_POINT('Ctrl Pts',(1.63321228097212,-9.22715823408952,5.92884199466574));
#80198=CARTESIAN_POINT('Ctrl Pts',(1.80283291570744,-9.19565758063653,5.93178222275854));
#80199=CARTESIAN_POINT('Ctrl Pts',(1.89448744222888,-9.17721320110186,5.93338427021411));
#80200=CARTESIAN_POINT('Ctrl Pts',(2.38356005989273,-9.07115416345611,5.94200468403278));
#80201=CARTESIAN_POINT('Ctrl Pts',(2.77522746517241,-8.95909065037087,5.9491849994521));
#80202=CARTESIAN_POINT('Ctrl Pts',(3.31793600891249,-8.76479395183734,5.95929956410146));
#80203=CARTESIAN_POINT('Ctrl Pts',(3.47593008452458,-8.70334548886938,5.96226151706799));
#80204=CARTESIAN_POINT('Ctrl Pts',(3.68315929617666,-8.61620462959695,5.96613622428821));
#80205=CARTESIAN_POINT('Ctrl Pts',(3.73395717965211,-8.59431256236282,5.9670851352119));
#80206=CARTESIAN_POINT('Ctrl Pts',(3.8232613194498,-8.55488444411153,5.96874992511386));
#80207=CARTESIAN_POINT('Ctrl Pts',(3.86184798868055,-8.5375350707468,5.969467948299));
#80208=CARTESIAN_POINT('Ctrl Pts',(3.95763751639169,-8.49368381194098,5.97124775036518));
#80209=CARTESIAN_POINT('Ctrl Pts',(4.01469281919533,-8.46686488627385,5.97230571577114));
#80210=CARTESIAN_POINT('Ctrl Pts',(4.2943905263886,-8.33192970363889,5.97749098320125));
#80211=CARTESIAN_POINT('Ctrl Pts',(4.51296022332444,-8.21559696187818,5.98154205998362));
#80212=CARTESIAN_POINT('Ctrl Pts',(4.90127265389691,-7.9887422866103,5.98891320350184));
#80213=CARTESIAN_POINT('Ctrl Pts',(5.07252944799921,-7.88111171000584,5.99222895008845));
#80214=CARTESIAN_POINT('Ctrl Pts',(5.29669247002343,-7.7298953858856,5.99670493233763));
#80215=CARTESIAN_POINT('Ctrl Pts',(5.35279778207977,-7.69115008866333,5.99783688370306));
#80216=CARTESIAN_POINT('Ctrl Pts',(5.49750932464677,-7.58886445666173,6.0007894917787));
#80217=CARTESIAN_POINT('Ctrl Pts',(5.58543813831908,-7.5243839109072,6.00261631358706));
#80218=CARTESIAN_POINT('Ctrl Pts',(5.73554978053464,-7.41022157855666,6.00579706183785));
#80219=CARTESIAN_POINT('Ctrl Pts',(5.79826198238004,-7.36125485754256,6.00714519553937));
#80220=CARTESIAN_POINT('Ctrl Pts',(5.93050039040628,-7.25526253176817,6.01003064519876));
#80221=CARTESIAN_POINT('Ctrl Pts',(5.9998447730445,-7.19802277959892,6.01156961779686));
#80222=CARTESIAN_POINT('Ctrl Pts',(6.21008701616427,-7.01933072453739,6.01631635684503));
#80223=CARTESIAN_POINT('Ctrl Pts',(6.3482006653884,-6.89467421333244,6.01954944924155));
#80224=CARTESIAN_POINT('Ctrl Pts',(6.68304780143827,-6.57385633702655,6.02766218432736));
#80225=CARTESIAN_POINT('Ctrl Pts',(6.87494211602099,-6.37290244745842,6.03256623544286));
#80226=CARTESIAN_POINT('Ctrl Pts',(7.11868235019254,-6.09381340562548,6.03904980089865));
#80227=CARTESIAN_POINT('Ctrl Pts',(7.17869567645664,-6.02299997189171,6.04066808171214));
#80228=CARTESIAN_POINT('Ctrl Pts',(7.28243353406133,-5.8968397757551,6.04349723011847));
#80229=CARTESIAN_POINT('Ctrl Pts',(7.32660380893084,-5.84186906573156,6.04471245642751));
#80230=CARTESIAN_POINT('Ctrl Pts',(7.39677938674177,-5.7524863658962,6.04665711473027));
#80231=CARTESIAN_POINT('Ctrl Pts',(7.42317490797182,-5.71838429931365,6.04739180323136));
#80232=CARTESIAN_POINT('Ctrl Pts',(7.48039739906122,-5.64339100616804,6.04899089194547));
#80233=CARTESIAN_POINT('Ctrl Pts',(7.51112641869461,-5.60242690575665,6.04985398855079));
#80234=CARTESIAN_POINT('Ctrl Pts',(7.60611145105714,-5.47361843266442,6.05253897098111));
#80235=CARTESIAN_POINT('Ctrl Pts',(7.66917390194261,-5.38490500557184,6.05434665620785));
#80236=CARTESIAN_POINT('Ctrl Pts',(7.8676380456355,-5.09515441374848,6.06014851421637));
#80237=CARTESIAN_POINT('Ctrl Pts',(7.99678989160347,-4.88995692451142,6.06410411972999));
#80238=CARTESIAN_POINT('Ctrl Pts',(8.23452758477266,-4.47758008298047,6.07191898043548));
#80239=CARTESIAN_POINT('Ctrl Pts',(8.34360334940062,-4.27088405500965,6.07577381401048));
#80240=CARTESIAN_POINT('Ctrl Pts',(8.48561924244266,-3.97551351444562,6.08125750714715));
#80241=CARTESIAN_POINT('Ctrl Pts',(8.52511868798272,-3.89008906491107,6.08284028780693));
#80242=CARTESIAN_POINT('Ctrl Pts',(8.59539006149435,-3.73190209083887,6.08576811064334));
#80243=CARTESIAN_POINT('Ctrl Pts',(8.6265415508776,-3.65931747216172,6.08711034630741));
#80244=CARTESIAN_POINT('Ctrl Pts',(8.69513139988357,-3.49375442873971,6.09017015153204));
#80245=CARTESIAN_POINT('Ctrl Pts',(8.73200308364739,-3.40055174197167,6.09189142017786));
#80246=CARTESIAN_POINT('Ctrl Pts',(8.87818120420275,-3.01298447179128,6.09904358072649));
#80247=CARTESIAN_POINT('Ctrl Pts',(8.97415229833049,-2.7138102195224,6.10455903332022));
#80248=CARTESIAN_POINT('Ctrl Pts',(9.11316904644161,-2.19157598664342,6.11406000186328));
#80249=CARTESIAN_POINT('Ctrl Pts',(9.1634651163244,-1.97072647352548,6.11803795897781));
#80250=CARTESIAN_POINT('Ctrl Pts',(9.21716623175992,-1.68795757367764,6.12300989367577));
#80251=CARTESIAN_POINT('Ctrl Pts',(9.22802765733316,-1.62753177992911,6.12406526133904));
#80252=CARTESIAN_POINT('Ctrl Pts',(9.24535277854114,-1.52539124957618,6.12583486318534));
#80253=CARTESIAN_POINT('Ctrl Pts',(9.2521298298479,-1.48373181188135,6.12655249295961));
#80254=CARTESIAN_POINT('Ctrl Pts',(9.26717202857151,-1.3871524800995,6.12820651012829));
#80255=CARTESIAN_POINT('Ctrl Pts',(9.27523082090141,-1.33220217993527,6.12914063691566));
#80256=CARTESIAN_POINT('Ctrl Pts',(9.30734094334531,-1.09881998767124,6.13308421471276));
#80257=CARTESIAN_POINT('Ctrl Pts',(9.32673551689654,-0.919785730008978,
6.13605122836288));
#80258=CARTESIAN_POINT('Ctrl Pts',(9.36110517231301,-0.486118346054322,
6.14319396722927));
#80259=CARTESIAN_POINT('Ctrl Pts',(9.37086654878271,-0.23121682214252,6.14735761199216));
#80260=CARTESIAN_POINT('Ctrl Pts',(9.36992485280812,0.140084800764607,6.15348879838844));
#80261=CARTESIAN_POINT('Ctrl Pts',(9.36746390813516,0.256389058886919,6.15541820411153));
#80262=CARTESIAN_POINT('Ctrl Pts',(9.35879843840504,0.474128364609442,6.15905592536975));
#80263=CARTESIAN_POINT('Ctrl Pts',(9.35310795757786,0.575567010995413,6.1607610334505));
#80264=CARTESIAN_POINT('Ctrl Pts',(9.34006485145293,0.755651429500956,6.1638101563054));
#80265=CARTESIAN_POINT('Ctrl Pts',(9.33336521440224,0.834334617044215,6.1651498692248));
#80266=CARTESIAN_POINT('Ctrl Pts',(9.31647616355166,1.00685918106568,6.16810487434907));
#80267=CARTESIAN_POINT('Ctrl Pts',(9.30586172229825,1.10065029206905,6.16972274481083));
#80268=CARTESIAN_POINT('Ctrl Pts',(9.24415484696524,1.58085645258049,6.17806514221114));
#80269=CARTESIAN_POINT('Ctrl Pts',(9.17040470885361,1.96397053843015,6.18493543586881));
#80270=CARTESIAN_POINT('Ctrl Pts',(9.02751260845457,2.51768919120335,6.19497591976177));
#80271=CARTESIAN_POINT('Ctrl Pts',(8.97688258804136,2.69264221034147,6.19816170903787));
#80272=CARTESIAN_POINT('Ctrl Pts',(8.90403957850057,2.91938474008857,6.20226775289852));
#80273=CARTESIAN_POINT('Ctrl Pts',(8.88641342281548,2.97260568770848,6.20322978455498));
#80274=CARTESIAN_POINT('Ctrl Pts',(8.85467119449909,3.06564305738611,6.20490658662642));
#80275=CARTESIAN_POINT('Ctrl Pts',(8.84076158880002,3.10552795067008,6.20562365861683));
#80276=CARTESIAN_POINT('Ctrl Pts',(8.80576343239858,3.20374191747348,6.20738551631121));
#80277=CARTESIAN_POINT('Ctrl Pts',(8.78436457079818,3.26195815636694,6.2084266982899));
#80278=CARTESIAN_POINT('Ctrl Pts',(8.64991813925135,3.61680362908467,6.21476486532073));
#80279=CARTESIAN_POINT('Ctrl Pts',(8.52243474113213,3.90774360523559,6.21993373757005));
#80280=CARTESIAN_POINT('Ctrl Pts',(8.30689683913583,4.33867169560046,6.22784173171171));
#80281=CARTESIAN_POINT('Ctrl Pts',(8.22950596118469,4.48373044069475,6.23054789652886));
#80282=CARTESIAN_POINT('Ctrl Pts',(8.08549781613653,4.73735243139542,6.23538890072163));
#80283=CARTESIAN_POINT('Ctrl Pts',(8.02040793978089,4.84673491668542,6.23751414641699));
#80284=CARTESIAN_POINT('Ctrl Pts',(7.9097753326328,5.02431643515025,6.2410346559183));
#80285=CARTESIAN_POINT('Ctrl Pts',(7.86552966502222,5.09330388890879,6.24242018847512));
#80286=CARTESIAN_POINT('Ctrl Pts',(7.77953288199946,5.22359578512762,6.24507261741535));
#80287=CARTESIAN_POINT('Ctrl Pts',(7.73794769652738,5.28500238471348,6.24633816674097));
#80288=CARTESIAN_POINT('Ctrl Pts',(7.62146209408408,5.4526878180565,6.24983747911631));
#80289=CARTESIAN_POINT('Ctrl Pts',(7.54507200662133,5.55791122351216,6.25208235871162));
#80290=CARTESIAN_POINT('Ctrl Pts',(7.25428179429235,5.94141136517929,6.26044358964722));
#80291=CARTESIAN_POINT('Ctrl Pts',(7.02647520775919,6.20915597284784,6.26665132712106));
#80292=CARTESIAN_POINT('Ctrl Pts',(6.68409099636591,6.56852845116939,6.27534631296114));
#80293=CARTESIAN_POINT('Ctrl Pts',(6.58157750046899,6.67124248291188,6.27787581403516));
#80294=CARTESIAN_POINT('Ctrl Pts',(6.43813779063008,6.80843721004593,6.28129415108693));
#80295=CARTESIAN_POINT('Ctrl Pts',(6.39924073447242,6.8450093859593,6.2822093666758));
#80296=CARTESIAN_POINT('Ctrl Pts',(6.32876291553775,6.91014892476682,6.28384501022444));
#80297=CARTESIAN_POINT('Ctrl Pts',(6.29729606227471,6.93883711491506,6.28456717303119));
#80298=CARTESIAN_POINT('Ctrl Pts',(6.22492724507355,7.00391769543092,6.28621039219053));
#80299=CARTESIAN_POINT('Ctrl Pts',(6.18389968847303,7.04016810531864,6.28712942377716));
#80300=CARTESIAN_POINT('Ctrl Pts',(5.87847339219256,7.30530141027337,6.29388843375093));
#80301=CARTESIAN_POINT('Ctrl Pts',(5.60176269398799,7.51958344087067,6.29956979912413));
#80302=CARTESIAN_POINT('Ctrl Pts',(5.13520482715964,7.84080554308283,6.30887825699849));
#80303=CARTESIAN_POINT('Ctrl Pts',(4.95247676866788,7.95748286948099,6.31245969834133));
#80304=CARTESIAN_POINT('Ctrl Pts',(4.68590103401696,8.11495797011017,6.31764236401883));
#80305=CARTESIAN_POINT('Ctrl Pts',(4.60523607126288,8.16100557731572,6.31920503690089));
#80306=CARTESIAN_POINT('Ctrl Pts',(4.45463507415977,8.24403221831331,6.3221147965681));
#80307=CARTESIAN_POINT('Ctrl Pts',(4.38488951279526,8.28133955270473,6.3234593300468));
#80308=CARTESIAN_POINT('Ctrl Pts',(4.30676807497231,8.32186356866996,6.32496243791178));
#80309=CARTESIAN_POINT('Ctrl Pts',(4.29885024370113,8.32595646683595,6.3251147489697));
#80310=CARTESIAN_POINT('Ctrl Pts',(4.2909266281297,8.33003803919931,6.32526713834515));
#80311=CARTESIAN_POINT('Origin',(0.,0.,2.15141010809499));
#80312=CARTESIAN_POINT('',(4.29124165107371,8.33064876708861,7.52288355898759));
#80313=CARTESIAN_POINT('',(4.2909265843892,8.3300380617307,7.32568828984052));
#80314=CARTESIAN_POINT('',(4.29092662815669,8.33003803918541,2.15141010809499));
#80315=CARTESIAN_POINT('',(-9.36967603564898,0.000162953396886864,6.84858989190502));
#80316=CARTESIAN_POINT('Ctrl Pts',(-9.36967603564898,0.000162953396886864,
6.84858989190502));
#80317=CARTESIAN_POINT('Ctrl Pts',(-9.36906102305612,-0.971808257735063,
6.8650963705856));
#80318=CARTESIAN_POINT('Ctrl Pts',(-8.97915541211587,-3.48971372166328,
6.90784845369182));
#80319=CARTESIAN_POINT('Ctrl Pts',(-6.75951736416114,-7.04192909134281,
6.97684614122372));
#80320=CARTESIAN_POINT('Ctrl Pts',(-2.6056775367071,-9.40692749512803,7.05558295450069));
#80321=CARTESIAN_POINT('Ctrl Pts',(2.17299000962536,-9.51619434133018,7.13431976777767));
#80322=CARTESIAN_POINT('Ctrl Pts',(6.43058602207351,-7.34352801700983,7.21305658105463));
#80323=CARTESIAN_POINT('Ctrl Pts',(9.14616145115302,-3.40992243802385,7.29179339433162));
#80324=CARTESIAN_POINT('Ctrl Pts',(9.6685356435055,1.34136454186004,7.37053020760858));
#80325=CARTESIAN_POINT('Ctrl Pts',(7.91137941483978,5.67497928827927,7.44756026249395));
#80326=CARTESIAN_POINT('Ctrl Pts',(5.57491667009454,7.66849856053472,7.49834471295364));
#80327=CARTESIAN_POINT('Ctrl Pts',(4.2912416510688,8.33064876709114,7.52288355898769));
#80328=CARTESIAN_POINT('Ctrl Pts',(-9.37024999848114,0.000168713661654052,
6.84892119005222));
#80329=CARTESIAN_POINT('Ctrl Pts',(-9.37024174247316,0.458702171958208,
6.84096250684365));
#80330=CARTESIAN_POINT('Ctrl Pts',(-9.33657615779602,0.916613734320751,
6.83280799835693));
#80331=CARTESIAN_POINT('Ctrl Pts',(-9.26117378581003,1.42671188575608,6.82386213762273));
#80332=CARTESIAN_POINT('Ctrl Pts',(-9.25230611491123,1.48313123801808,6.82287514079911));
#80333=CARTESIAN_POINT('Ctrl Pts',(-9.23619781542005,1.57984514384641,6.82118932015834));
#80334=CARTESIAN_POINT('Ctrl Pts',(-9.22920788916571,1.62017977724394,6.82048807311815));
#80335=CARTESIAN_POINT('Ctrl Pts',(-9.21446289039731,1.702070997951,6.81906891847766));
#80336=CARTESIAN_POINT('Ctrl Pts',(-9.20669049302843,1.74362329928961,6.81835139424002));
#80337=CARTESIAN_POINT('Ctrl Pts',(-9.18672196617001,1.84652005018696,6.81658040300009));
#80338=CARTESIAN_POINT('Ctrl Pts',(-9.17419234626702,1.90779757813584,6.8155306468891));
#80339=CARTESIAN_POINT('Ctrl Pts',(-9.12649736516666,2.12971138493879,6.81174003623811));
#80340=CARTESIAN_POINT('Ctrl Pts',(-9.08771855457536,2.28954067268794,6.80903053365417));
#80341=CARTESIAN_POINT('Ctrl Pts',(-9.03624107412047,2.47971648816626,6.80579543716441));
#80342=CARTESIAN_POINT('Ctrl Pts',(-9.02756419917994,2.51112151073629,6.80526085579008));
#80343=CARTESIAN_POINT('Ctrl Pts',(-9.00680286197389,2.58476642305526,6.80400596324978));
#80344=CARTESIAN_POINT('Ctrl Pts',(-8.99458477067406,2.62696784526347,6.80328585368802));
#80345=CARTESIAN_POINT('Ctrl Pts',(-8.92317946438855,2.86726302420927,6.79917710657475));
#80346=CARTESIAN_POINT('Ctrl Pts',(-8.85774573983435,3.06344075383916,6.79578848590553));
#80347=CARTESIAN_POINT('Ctrl Pts',(-8.74896410420198,3.35685681789658,6.79060979358623));
#80348=CARTESIAN_POINT('Ctrl Pts',(-8.71036184534189,3.45578602512267,6.7888445318475));
#80349=CARTESIAN_POINT('Ctrl Pts',(-8.63494860686427,3.63975687279058,6.78551937821395));
#80350=CARTESIAN_POINT('Ctrl Pts',(-8.59854136401997,3.72495018706322,6.78396221380906));
#80351=CARTESIAN_POINT('Ctrl Pts',(-8.52987155896806,3.87926438556947,6.78110724981502));
#80352=CARTESIAN_POINT('Ctrl Pts',(-8.49801683060932,3.94855807883894,6.77981238981641));
#80353=CARTESIAN_POINT('Ctrl Pts',(-8.42374798529678,4.10505255456956,6.77685776503906));
#80354=CARTESIAN_POINT('Ctrl Pts',(-8.38081906958307,4.19199931505509,6.77519450020538));
#80355=CARTESIAN_POINT('Ctrl Pts',(-8.22110539957664,4.50321451100649,6.76916211847607));
#80356=CARTESIAN_POINT('Ctrl Pts',(-8.09660496314985,4.72339942635138,6.76474130708951));
#80357=CARTESIAN_POINT('Ctrl Pts',(-7.85266114107542,5.11677757496733,6.75660984586563));
#80358=CARTESIAN_POINT('Ctrl Pts',(-7.73599886821021,5.29150463687477,6.7529087933557));
#80359=CARTESIAN_POINT('Ctrl Pts',(-7.56559312488128,5.52902865643566,6.74780295833642));
#80360=CARTESIAN_POINT('Ctrl Pts',(-7.51674348616794,5.59525911980468,6.74637103658131));
#80361=CARTESIAN_POINT('Ctrl Pts',(-7.43186477738892,5.70721987863468,6.74394137435124));
#80362=CARTESIAN_POINT('Ctrl Pts',(-7.39627038011127,5.75327361569894,6.74293929555495));
#80363=CARTESIAN_POINT('Ctrl Pts',(-7.35966877889239,5.79972942532535,6.74192694366899));
#80364=CARTESIAN_POINT('Ctrl Pts',(-7.35908828302135,5.8004659799611,6.74191089248809));
#80365=CARTESIAN_POINT('Ctrl Pts',(-7.35755458642954,5.80241139011471,6.74186849661121));
#80366=CARTESIAN_POINT('Ctrl Pts',(-7.35660119833329,5.80362009793067,6.74184215448131));
#80367=CARTESIAN_POINT('Ctrl Pts',(-7.35415656162453,5.80671784417866,6.74177464074576));
#80368=CARTESIAN_POINT('Ctrl Pts',(-7.35266488295041,5.80860654320961,6.74173347507072));
#80369=CARTESIAN_POINT('Ctrl Pts',(-7.34897529552922,5.81327444070427,6.74163172866638));
#80370=CARTESIAN_POINT('Ctrl Pts',(-7.3467765376102,5.81605296774968,6.74157115977476));
#80371=CARTESIAN_POINT('Ctrl Pts',(-7.34322220186211,5.82053928005766,6.7414733550675));
#80372=CARTESIAN_POINT('Ctrl Pts',(-7.34186760316945,5.8222478403231,6.74143610541152));
#80373=CARTESIAN_POINT('Ctrl Pts',(-7.31428791394129,5.85700927284497,6.74067820771852));
#80374=CARTESIAN_POINT('Ctrl Pts',(-7.28784050782147,5.8898850630803,6.73996086584397));
#80375=CARTESIAN_POINT('Ctrl Pts',(-7.22592419142597,5.96579537834134,6.73830331550946));
#80376=CARTESIAN_POINT('Ctrl Pts',(-7.19029143554791,6.00869403511289,6.73736541525924));
#80377=CARTESIAN_POINT('Ctrl Pts',(-7.04432670067132,6.1812647352471,6.73358219127143));
#80378=CARTESIAN_POINT('Ctrl Pts',(-6.9308527311781,6.30823692848806,6.7307742557749));
#80379=CARTESIAN_POINT('Ctrl Pts',(-6.63460323537928,6.62207772888062,6.72368494586477));
#80380=CARTESIAN_POINT('Ctrl Pts',(-6.44735336632636,6.80452115523511,6.71941962861559));
#80381=CARTESIAN_POINT('Ctrl Pts',(-6.16522885965651,7.05728974505148,6.71316611543111));
#80382=CARTESIAN_POINT('Ctrl Pts',(-6.0762679787279,7.13402781096093,6.71121801563212));
#80383=CARTESIAN_POINT('Ctrl Pts',(-5.90720839705525,7.27440255069153,6.70755043766786));
#80384=CARTESIAN_POINT('Ctrl Pts',(-5.82746473998336,7.33843976279926,6.70583428676418));
#80385=CARTESIAN_POINT('Ctrl Pts',(-5.68428987080573,7.4496090376287,6.70277355194577));
#80386=CARTESIAN_POINT('Ctrl Pts',(-5.62128058872318,7.4972682130247,6.70143340391258));
#80387=CARTESIAN_POINT('Ctrl Pts',(-5.48208747517783,7.59981029453659,6.6984866560835));
#80388=CARTESIAN_POINT('Ctrl Pts',(-5.40566616993475,7.6543564590344,6.69687757748631));
#80389=CARTESIAN_POINT('Ctrl Pts',(-4.99972262731092,7.93498913695198,6.68837552092417));
#80390=CARTESIAN_POINT('Ctrl Pts',(-4.65680760682547,8.14097159027103,6.68132764224587));
#80391=CARTESIAN_POINT('Ctrl Pts',(-4.14652522274127,8.40466899107092,6.67124621532479));
#80392=CARTESIAN_POINT('Ctrl Pts',(-3.98903967474142,8.48054803865381,6.66819039764238));
#80393=CARTESIAN_POINT('Ctrl Pts',(-3.77873692086913,8.57472033849949,6.66421830000596));
#80394=CARTESIAN_POINT('Ctrl Pts',(-3.7277481343934,8.59700968165085,6.66326355323828));
#80395=CARTESIAN_POINT('Ctrl Pts',(-3.63767886321769,8.63543077804461,6.66159346396252));
#80396=CARTESIAN_POINT('Ctrl Pts',(-3.59868232226685,8.65175460709144,6.66087590706295));
#80397=CARTESIAN_POINT('Ctrl Pts',(-3.51125278832007,8.68765894326536,6.65927898621263));
#80398=CARTESIAN_POINT('Ctrl Pts',(-3.46276394665995,8.70709939779863,6.65840121836173));
#80399=CARTESIAN_POINT('Ctrl Pts',(-3.12886272983523,8.83773883551723,6.65240319934048));
#80400=CARTESIAN_POINT('Ctrl Pts',(-2.83830833995859,8.93529054394326,6.64740935290815));
#80401=CARTESIAN_POINT('Ctrl Pts',(-2.29485172730786,9.08856333244864,6.63814782826857));
#80402=CARTESIAN_POINT('Ctrl Pts',(-2.04341195090278,9.14837662853422,6.63389389336607));
#80403=CARTESIAN_POINT('Ctrl Pts',(-1.69615718729479,9.2159503814685,6.62797725810729));
#80404=CARTESIAN_POINT('Ctrl Pts',(-1.60221820176393,9.23274538885601,6.62637301511406));
#80405=CARTESIAN_POINT('Ctrl Pts',(-1.43796624952718,9.25952908725064,6.62355893382753));
#80406=CARTESIAN_POINT('Ctrl Pts',(-1.36776573092296,9.27015872211614,6.62235335481336));
#80407=CARTESIAN_POINT('Ctrl Pts',(-1.20248569920118,9.29326680749097,6.61950748597603));
#80408=CARTESIAN_POINT('Ctrl Pts',(-1.10732207204248,9.30508557626445,6.6178631056096));
#80409=CARTESIAN_POINT('Ctrl Pts',(-0.777732754721942,9.34089090067309,
6.61214780552308));
#80410=CARTESIAN_POINT('Ctrl Pts',(-0.542595719124867,9.35749433550255,
6.60803304030991));
#80411=CARTESIAN_POINT('Ctrl Pts',(-0.0414449364577233,9.3739270047127,
6.59923027845724));
#80412=CARTESIAN_POINT('Ctrl Pts',(0.224444660868916,9.37133127361447,6.59453960626259));
#80413=CARTESIAN_POINT('Ctrl Pts',(0.581562626996471,9.35263608624222,6.58831647710312));
#80414=CARTESIAN_POINT('Ctrl Pts',(0.673186514475996,9.34648794124671,6.5867270922813));
#80415=CARTESIAN_POINT('Ctrl Pts',(0.81111981367436,9.33519354144149,6.58435203501646));
#80416=CARTESIAN_POINT('Ctrl Pts',(0.857505359061592,9.33104701412207,6.58355635303037));
#80417=CARTESIAN_POINT('Ctrl Pts',(0.943616297067151,9.32270180285456,6.5820860467029));
#80418=CARTESIAN_POINT('Ctrl Pts',(0.983349462781458,9.31859455392666,6.58141034315896));
#80419=CARTESIAN_POINT('Ctrl Pts',(1.10065906486532,9.30570952181116,6.5794219238715));
#80420=CARTESIAN_POINT('Ctrl Pts',(1.17815354946662,9.29621613030456,6.57811683437324));
#80421=CARTESIAN_POINT('Ctrl Pts',(1.60934123220643,9.23791554706517,6.57088242241443));
#80422=CARTESIAN_POINT('Ctrl Pts',(1.96013945505633,9.16989193264125,6.56508747683734));
#80423=CARTESIAN_POINT('Ctrl Pts',(2.43300685114192,9.04981655363189,6.55705140180732));
#80424=CARTESIAN_POINT('Ctrl Pts',(2.55912557962672,9.0149641240943,6.55488716664965));
#80425=CARTESIAN_POINT('Ctrl Pts',(2.78974850008086,8.946002587799,6.5508773383682));
#80426=CARTESIAN_POINT('Ctrl Pts',(2.89446202384925,8.91267347685104,6.54903657578847));
#80427=CARTESIAN_POINT('Ctrl Pts',(3.07402830222481,8.85202120897565,6.54584035820915));
#80428=CARTESIAN_POINT('Ctrl Pts',(3.14916347179829,8.82557073964811,6.54449086971189));
#80429=CARTESIAN_POINT('Ctrl Pts',(3.30800163769169,8.76736694218404,6.54161100474566));
#80430=CARTESIAN_POINT('Ctrl Pts',(3.39160532867814,8.73536554356725,6.54007905802973));
#80431=CARTESIAN_POINT('Ctrl Pts',(3.64423474391702,8.63449176354428,6.53540009955608));
#80432=CARTESIAN_POINT('Ctrl Pts',(3.81171791914635,8.56187485510295,6.53222890978592));
#80433=CARTESIAN_POINT('Ctrl Pts',(4.0825764503003,8.43491298136176,6.52699730798063));
#80434=CARTESIAN_POINT('Ctrl Pts',(4.18724592612468,8.38344551260659,6.52494983632478));
#80435=CARTESIAN_POINT('Ctrl Pts',(4.29092662818984,8.33003803916834,6.5228999581952));
#80436=CARTESIAN_POINT('Ctrl Pts',(4.2909266281297,8.33003803919931,6.32526713834515));
#80437=CARTESIAN_POINT('Ctrl Pts',(4.20824026393393,8.37263101659524,6.32685738755457));
#80438=CARTESIAN_POINT('Ctrl Pts',(4.12492400055656,8.41399063344705,6.32845622925807));
#80439=CARTESIAN_POINT('Ctrl Pts',(3.72134241221821,8.60689996893795,6.33618347881133));
#80440=CARTESIAN_POINT('Ctrl Pts',(3.3932713294365,8.74144289771762,6.34242481601055));
#80441=CARTESIAN_POINT('Ctrl Pts',(2.87651681075672,8.91987955999178,6.35202744607353));
#80442=CARTESIAN_POINT('Ctrl Pts',(2.69276846007288,8.97705957941376,6.35539642645059));
#80443=CARTESIAN_POINT('Ctrl Pts',(2.45288962748264,9.04367828578183,6.35968954079036));
#80444=CARTESIAN_POINT('Ctrl Pts',(2.3982530822198,9.05832029876584,6.36066033871355));
#80445=CARTESIAN_POINT('Ctrl Pts',(2.30262220965142,9.08302248135346,6.36234534204425));
#80446=CARTESIAN_POINT('Ctrl Pts',(2.26168648128923,9.09330196918904,6.36306195347132));
#80447=CARTESIAN_POINT('Ctrl Pts',(2.16104659776772,9.11785230962641,6.36481271171676));
#80448=CARTESIAN_POINT('Ctrl Pts',(2.10126909235884,9.13181369521687,6.36584338614031));
#80449=CARTESIAN_POINT('Ctrl Pts',(1.7288101627805,9.21495275809605,6.37221909341532));
#80450=CARTESIAN_POINT('Ctrl Pts',(1.4128894275344,9.26865061007484,6.37743276842286));
#80451=CARTESIAN_POINT('Ctrl Pts',(0.932333361058202,9.32518704685286,6.38537475168573));
#80452=CARTESIAN_POINT('Ctrl Pts',(0.76935417498574,9.34004566161037,6.38806870842036));
#80453=CARTESIAN_POINT('Ctrl Pts',(0.479428746746019,9.35883745518134,6.39289142743024));
#80454=CARTESIAN_POINT('Ctrl Pts',(0.35263413409879,9.36447219458713,6.39501071926421));
#80455=CARTESIAN_POINT('Ctrl Pts',(0.143887695419758,9.36950314043737,6.39852434619891));
#80456=CARTESIAN_POINT('Ctrl Pts',(0.0619886648817329,9.37040288012853,
6.39990903381663));
#80457=CARTESIAN_POINT('Ctrl Pts',(-0.0941224008508102,9.37007114797953,
6.40256151633704));
#80458=CARTESIAN_POINT('Ctrl Pts',(-0.168328701385573,9.36903184778882,
6.40382798079593));
#80459=CARTESIAN_POINT('Ctrl Pts',(-0.372867328048197,9.3637363381592,6.40733483900856));
#80460=CARTESIAN_POINT('Ctrl Pts',(-0.50313497886277,9.35764090503565,6.4095864368847));
#80461=CARTESIAN_POINT('Ctrl Pts',(-0.960429953277878,9.32666653321074,
6.41754968359261));
#80462=CARTESIAN_POINT('Ctrl Pts',(-1.28623767891919,9.28734222648609,6.42333788372226));
#80463=CARTESIAN_POINT('Ctrl Pts',(-1.77075907769906,9.20287213044927,6.4319649872657));
#80464=CARTESIAN_POINT('Ctrl Pts',(-1.93144257299956,9.17049469789188,6.4348274384152));
#80465=CARTESIAN_POINT('Ctrl Pts',(-2.14473741065076,9.12166123210943,6.43859828039155));
#80466=CARTESIAN_POINT('Ctrl Pts',(-2.19817172710813,9.10893205984011,6.43954045247104));
#80467=CARTESIAN_POINT('Ctrl Pts',(-2.29259999103672,9.08555798128995,6.4411992058699));
#80468=CARTESIAN_POINT('Ctrl Pts',(-2.33363923979937,9.07510366062315,6.44191785002316));
#80469=CARTESIAN_POINT('Ctrl Pts',(-2.43612903831635,9.04825426077827,6.44370754459808));
#80470=CARTESIAN_POINT('Ctrl Pts',(-2.49748609012978,9.03151112028137,6.44477466704706));
#80471=CARTESIAN_POINT('Ctrl Pts',(-2.73366320524356,8.9644721657767,6.44887322371298));
#80472=CARTESIAN_POINT('Ctrl Pts',(-2.90717534258993,8.90971422774936,6.45186578918107));
#80473=CARTESIAN_POINT('Ctrl Pts',(-3.18788479722213,8.81205257097316,6.45674217652053));
#80474=CARTESIAN_POINT('Ctrl Pts',(-3.29607728271606,8.77215791843709,6.45863016648515));
#80475=CARTESIAN_POINT('Ctrl Pts',(-3.56501848524114,8.66731095973559,6.46336515421568));
#80476=CARTESIAN_POINT('Ctrl Pts',(-3.72475240996275,8.59987531305519,6.46621594881002));
#80477=CARTESIAN_POINT('Ctrl Pts',(-3.93902149984893,8.50232605457052,6.47012079239418));
#80478=CARTESIAN_POINT('Ctrl Pts',(-3.99526265433698,8.47604359499193,6.47115336904407));
#80479=CARTESIAN_POINT('Ctrl Pts',(-4.14366428661825,8.40488773471997,6.47390008629846));
#80480=CARTESIAN_POINT('Ctrl Pts',(-4.23535657858824,8.3590577302389,6.47562007556154));
#80481=CARTESIAN_POINT('Ctrl Pts',(-4.39636673767234,8.27525152679643,6.47868487060906));
#80482=CARTESIAN_POINT('Ctrl Pts',(-4.46599078959337,8.23788532072609,6.48002519394716));
#80483=CARTESIAN_POINT('Ctrl Pts',(-4.61714414592048,8.15428403568982,6.48296920031215));
#80484=CARTESIAN_POINT('Ctrl Pts',(-4.69846921875761,8.10769727751822,6.48457532857659));
#80485=CARTESIAN_POINT('Ctrl Pts',(-5.12550919225414,7.85448579046357,6.49312796643928));
#80486=CARTESIAN_POINT('Ctrl Pts',(-5.45833183394866,7.62695231257382,6.50023235948535));
#80487=CARTESIAN_POINT('Ctrl Pts',(-5.91131825881639,7.27239020338144,6.5103276591376));
#80488=CARTESIAN_POINT('Ctrl Pts',(-6.04419722406677,7.16233362996991,6.51334310653496));
#80489=CARTESIAN_POINT('Ctrl Pts',(-6.21571679698328,7.01209888397556,6.51727338736357));
#80490=CARTESIAN_POINT('Ctrl Pts',(-6.25714541854583,6.97515571792162,6.5182256857719));
#80491=CARTESIAN_POINT('Ctrl Pts',(-6.32955403462572,6.90942248458571,6.51989354515226));
#80492=CARTESIAN_POINT('Ctrl Pts',(-6.3606717625331,6.88078687945077,6.52061129108964));
#80493=CARTESIAN_POINT('Ctrl Pts',(-6.43749596167262,6.80912410331586,6.52238629887018));
#80494=CARTESIAN_POINT('Ctrl Pts',(-6.48296585722228,6.7658465125396,6.5234398030005));
#80495=CARTESIAN_POINT('Ctrl Pts',(-6.71016004486372,6.54521311962335,6.52872824975175));
#80496=CARTESIAN_POINT('Ctrl Pts',(-6.88505713637971,6.36097883502184,6.53288252106733));
#80497=CARTESIAN_POINT('Ctrl Pts',(-7.22621487569311,5.97103024232393,6.54137494910345));
#80498=CARTESIAN_POINT('Ctrl Pts',(-7.39168681102954,5.7649240447985,6.5457105629208));
#80499=CARTESIAN_POINT('Ctrl Pts',(-7.61292421675052,5.46414603557416,6.55193142581384));
#80500=CARTESIAN_POINT('Ctrl Pts',(-7.67607818208552,5.37506564516312,6.55376083588463));
#80501=CARTESIAN_POINT('Ctrl Pts',(-7.78254362240083,5.21918887593585,6.55694445207441));
#80502=CARTESIAN_POINT('Ctrl Pts',(-7.8265874254669,5.15290665493554,6.55829283325664));
#80503=CARTESIAN_POINT('Ctrl Pts',(-7.91854415724771,5.01062014153191,6.56117721864386));
#80504=CARTESIAN_POINT('Ctrl Pts',(-7.96621910439647,4.93447149192677,6.56271486322442));
#80505=CARTESIAN_POINT('Ctrl Pts',(-8.1051545293239,4.70529467012887,6.56732522604309));
#80506=CARTESIAN_POINT('Ctrl Pts',(-8.19315310824621,4.55033731634271,6.57042050558338));
#80507=CARTESIAN_POINT('Ctrl Pts',(-8.30265755532397,4.3440226589768,6.57450460622988));
#80508=CARTESIAN_POINT('Ctrl Pts',(-8.32820029713551,4.29484983992455,6.57547524030563));
#80509=CARTESIAN_POINT('Ctrl Pts',(-8.4624976702542,4.03060786958886,6.58067430231056));
#80510=CARTESIAN_POINT('Ctrl Pts',(-8.56336057146384,3.81162987168666,6.58492594136708));
#80511=CARTESIAN_POINT('Ctrl Pts',(-8.68919922298438,3.50814271958098,6.59066975704457));
#80512=CARTESIAN_POINT('Ctrl Pts',(-8.72159448101979,3.4268116714448,6.59219457370145));
#80513=CARTESIAN_POINT('Ctrl Pts',(-8.77701592261415,3.28179232405076,6.59488159768706));
#80514=CARTESIAN_POINT('Ctrl Pts',(-8.80050030155519,3.2182858540113,6.5960475993619));
#80515=CARTESIAN_POINT('Ctrl Pts',(-8.83769088598625,3.11426292908294,6.59793708464703));
#80516=CARTESIAN_POINT('Ctrl Pts',(-8.85181160523465,3.07389738191817,6.59866524703378));
#80517=CARTESIAN_POINT('Ctrl Pts',(-8.88265658544073,2.98374847660182,6.60027964150398));
#80518=CARTESIAN_POINT('Ctrl Pts',(-8.89923961049517,2.93391843071666,6.60116427426703));
#80519=CARTESIAN_POINT('Ctrl Pts',(-8.95186257493057,2.77124061841614,6.60403089765138));
#80520=CARTESIAN_POINT('Ctrl Pts',(-8.98618170022141,2.6578481346027,6.60599580352137));
#80521=CARTESIAN_POINT('Ctrl Pts',(-9.0461723918034,2.44517062483138,6.60964168680928));
#80522=CARTESIAN_POINT('Ctrl Pts',(-9.07238208013147,2.34605578698333,6.61132501026122));
#80523=CARTESIAN_POINT('Ctrl Pts',(-9.1529821868891,2.0196788000834,6.61683843514445));
#80524=CARTESIAN_POINT('Ctrl Pts',(-9.20049903656893,1.79081063880487,6.62065987325839));
#80525=CARTESIAN_POINT('Ctrl Pts',(-9.25172869110868,1.4874718417392,6.62574405826794));
#80526=CARTESIAN_POINT('Ctrl Pts',(-9.26318228279751,1.41439394421316,6.62697014179774));
#80527=CARTESIAN_POINT('Ctrl Pts',(-9.29022982107847,1.22737124525593,6.63011435924624));
#80528=CARTESIAN_POINT('Ctrl Pts',(-9.30459347820935,1.1132611619497,6.63203890163003));
#80529=CARTESIAN_POINT('Ctrl Pts',(-9.32540890492238,0.919116408501615,
6.63532923704868));
#80530=CARTESIAN_POINT('Ctrl Pts',(-9.33293908699647,0.839210450188303,
6.63668800124707));
#80531=CARTESIAN_POINT('Ctrl Pts',(-9.34652946062281,0.672029815884449,
6.63954153538251));
#80532=CARTESIAN_POINT('Ctrl Pts',(-9.35239583542012,0.584747059711993,
6.6410374130638));
#80533=CARTESIAN_POINT('Ctrl Pts',(-9.36584853270982,0.331673772450509,
6.64539283026322));
#80534=CARTESIAN_POINT('Ctrl Pts',(-9.37025365261961,0.165748127334882,
6.64827145372313));
#80535=CARTESIAN_POINT('Ctrl Pts',(-9.37024411107238,-0.267496655689389,
6.65583566090191));
#80536=CARTESIAN_POINT('Ctrl Pts',(-9.35880136501872,-0.534664099895355,
6.66055035175185));
#80537=CARTESIAN_POINT('Ctrl Pts',(-9.32190719239578,-0.964692744892784,
6.66812158653535));
#80538=CARTESIAN_POINT('Ctrl Pts',(-9.30355699977813,-1.12801294492445,
6.67099194262106));
#80539=CARTESIAN_POINT('Ctrl Pts',(-9.27339214416323,-1.34490555949817,
6.67476612574503));
#80540=CARTESIAN_POINT('Ctrl Pts',(-9.26538899607317,-1.3989780531286,6.6757038546749));
#80541=CARTESIAN_POINT('Ctrl Pts',(-9.25101802354444,-1.49053545540155,
6.67728451737122));
#80542=CARTESIAN_POINT('Ctrl Pts',(-9.24489437543979,-1.52805706938749,
6.67793014740305));
#80543=CARTESIAN_POINT('Ctrl Pts',(-9.22870856086925,-1.62357253562602,
6.67956846566657));
#80544=CARTESIAN_POINT('Ctrl Pts',(-9.21832801407941,-1.68151066811122,
6.68055755853936));
#80545=CARTESIAN_POINT('Ctrl Pts',(-9.19407233098427,-1.80991046540066,
6.68274262716521));
#80546=CARTESIAN_POINT('Ctrl Pts',(-9.17993165798706,-1.88031824547836,
6.68393616856785));
#80547=CARTESIAN_POINT('Ctrl Pts',(-9.13174724951051,-2.10671992351238,
6.6877677277722));
#80548=CARTESIAN_POINT('Ctrl Pts',(-9.09452550754735,-2.26200853588946,
6.69038639023632));
#80549=CARTESIAN_POINT('Ctrl Pts',(-8.9722266583208,-2.72024154516597,6.69816078213647));
#80550=CARTESIAN_POINT('Ctrl Pts',(-8.87584161743937,-3.01993382881891,
6.70331344426076));
#80551=CARTESIAN_POINT('Ctrl Pts',(-8.72914153835272,-3.40788848839428,
6.71023805630158));
#80552=CARTESIAN_POINT('Ctrl Pts',(-8.6922178724756,-3.50099476428026,6.71191909911516));
#80553=CARTESIAN_POINT('Ctrl Pts',(-8.62351997479047,-3.66643234666547,
6.71494403657693));
#80554=CARTESIAN_POINT('Ctrl Pts',(-8.59231017433845,-3.73898766280242,
6.71628393186724));
#80555=CARTESIAN_POINT('Ctrl Pts',(-8.52188798483405,-3.89716268693931,
6.71923526735081));
#80556=CARTESIAN_POINT('Ctrl Pts',(-8.48229462132644,-3.98260338665169,
6.7208492417781));
#80557=CARTESIAN_POINT('Ctrl Pts',(-8.33964061557356,-4.27866297031005,
6.72651149998721));
#80558=CARTESIAN_POINT('Ctrl Pts',(-8.22996871619734,-4.48599784199792,
6.73060372285002));
#80559=CARTESIAN_POINT('Ctrl Pts',(-7.99124605928136,-4.89902198805559,
6.73897662866561));
#80560=CARTESIAN_POINT('Ctrl Pts',(-7.86174600062069,-5.10425115443418,
6.74325582356164));
#80561=CARTESIAN_POINT('Ctrl Pts',(-7.66329096277337,-5.39325703853608,
6.74937581354169));
#80562=CARTESIAN_POINT('Ctrl Pts',(-7.6006183271226,-5.4812271443114,6.75125145799657));
#80563=CARTESIAN_POINT('Ctrl Pts',(-7.50609528106919,-5.60916448234785,
6.75398799496152));
#80564=CARTESIAN_POINT('Ctrl Pts',(-7.47541641059412,-5.64998602318732,
6.75486247957521));
#80565=CARTESIAN_POINT('Ctrl Pts',(-7.41818798621652,-5.7248524647942,6.75646720631707));
#80566=CARTESIAN_POINT('Ctrl Pts',(-7.39173394995275,-5.75896847993369,
6.75719866677571));
#80567=CARTESIAN_POINT('Ctrl Pts',(-7.32123968676158,-5.84859429466323,
6.75912210074726));
#80568=CARTESIAN_POINT('Ctrl Pts',(-7.27680389508847,-5.9037895357871,6.76030863794319));
#80569=CARTESIAN_POINT('Ctrl Pts',(-7.17230964560699,-6.03061323333406,
6.7630459445076));
#80570=CARTESIAN_POINT('Ctrl Pts',(-7.11179686280728,-6.10185767273908,
6.76459198180125));
#80571=CARTESIAN_POINT('Ctrl Pts',(-6.86398704101554,-6.38492045084358,
6.77079127370103));
#80572=CARTESIAN_POINT('Ctrl Pts',(-6.66821250212998,-6.58911751679026,
6.77539837018513));
#80573=CARTESIAN_POINT('Ctrl Pts',(-6.33207159013447,-6.90937115017145,
6.78304898417604));
#80574=CARTESIAN_POINT('Ctrl Pts',(-6.19702705033104,-7.03074645840779,
6.78605910316685));
#80575=CARTESIAN_POINT('Ctrl Pts',(-5.99034192139613,-7.20592682846436,
6.79060033235791));
#80576=CARTESIAN_POINT('Ctrl Pts',(-5.9213176254947,-7.26275259962494,6.79210632935388));
#80577=CARTESIAN_POINT('Ctrl Pts',(-5.78925777866192,-7.36833958383894,
6.79497002433603));
#80578=CARTESIAN_POINT('Ctrl Pts',(-5.72639267547684,-7.41730144608719,
6.79632591308752));
#80579=CARTESIAN_POINT('Ctrl Pts',(-5.57516702464599,-7.5320134527295,6.79957115904164));
#80580=CARTESIAN_POINT('Ctrl Pts',(-5.48625677808336,-7.59701918400953,
6.80146615713298));
#80581=CARTESIAN_POINT('Ctrl Pts',(-5.28889509188134,-7.73604605996295,
6.80564378570293));
#80582=CARTESIAN_POINT('Ctrl Pts',(-5.17999185345099,-7.80938564894754,
6.80793057915229));
#80583=CARTESIAN_POINT('Ctrl Pts',(-4.76568183430128,-8.07591730049529,
6.81654959844975));
#80584=CARTESIAN_POINT('Ctrl Pts',(-4.45072574246145,-8.25367816709756,
6.82295252042373));
#80585=CARTESIAN_POINT('Ctrl Pts',(-4.05894037752644,-8.44584014711669,
6.83051973501605));
#80586=CARTESIAN_POINT('Ctrl Pts',(-3.99119314048399,-8.47806523539099,
6.83181392379026));
#80587=CARTESIAN_POINT('Ctrl Pts',(-3.88719491010502,-8.52601085077349,
6.83377506317719));
#80588=CARTESIAN_POINT('Ctrl Pts',(-3.85121938346786,-8.54232138067351,
6.83444884426768));
#80589=CARTESIAN_POINT('Ctrl Pts',(-3.77185744820174,-8.57769912527549,
6.83592422271375));
#80590=CARTESIAN_POINT('Ctrl Pts',(-3.72842735553502,-8.59666565364904,
6.83672452647371));
#80591=CARTESIAN_POINT('Ctrl Pts',(-3.59577947189541,-8.65340054786662,
6.83914995720847));
#80592=CARTESIAN_POINT('Ctrl Pts',(-3.50611803014959,-8.6901155050585,6.84076354239898));
#80593=CARTESIAN_POINT('Ctrl Pts',(-3.17405114999465,-8.82011573141159,
6.84666964571213));
#80594=CARTESIAN_POINT('Ctrl Pts',(-2.92836656533185,-8.90470168302863,
6.8509066761065));
#80595=CARTESIAN_POINT('Ctrl Pts',(-2.55894849871085,-9.01494263754395,
6.85723461668853));
#80596=CARTESIAN_POINT('Ctrl Pts',(-2.43769923618985,-9.04848222343519,
6.85930423678493));
#80597=CARTESIAN_POINT('Ctrl Pts',(-2.17296332295374,-9.11600507887425,
6.86382446354094));
#80598=CARTESIAN_POINT('Ctrl Pts',(-2.02927535180065,-9.14906331664298,
6.86627886565215));
#80599=CARTESIAN_POINT('Ctrl Pts',(-1.80168774660806,-9.1957988772824,6.87018116784542));
#80600=CARTESIAN_POINT('Ctrl Pts',(-1.71827961100136,-9.21174852377251,
6.87161432072911));
#80601=CARTESIAN_POINT('Ctrl Pts',(-1.55442491328724,-9.24077859510195,
6.87443732298519));
#80602=CARTESIAN_POINT('Ctrl Pts',(-1.47400156303259,-9.25394754739045,
6.8758264642474));
#80603=CARTESIAN_POINT('Ctrl Pts',(-1.27072721898639,-9.28451563240686,
6.87934730439972));
#80604=CARTESIAN_POINT('Ctrl Pts',(-1.14768358519643,-9.30052689150229,
6.88148751923919));
#80605=CARTESIAN_POINT('Ctrl Pts',(-0.941650831733427,-9.32318626282142,
6.8850846845736));
#80606=CARTESIAN_POINT('Ctrl Pts',(-0.858825653195946,-9.33118035664859,
6.88653430504898));
#80607=CARTESIAN_POINT('Ctrl Pts',(-0.479909591704592,-9.36266468880521,
6.89317829524937));
#80608=CARTESIAN_POINT('Ctrl Pts',(-0.182912844519505,-9.37317158931048,
6.89842552408248));
#80609=CARTESIAN_POINT('Ctrl Pts',(0.24299964819959,-9.36798585782343,6.90587752519452));
#80610=CARTESIAN_POINT('Ctrl Pts',(0.371873723630866,-9.36375554708974,
6.90812183222999));
#80611=CARTESIAN_POINT('Ctrl Pts',(0.553381355308638,-9.35404436110688,
6.91125145093967));
#80612=CARTESIAN_POINT('Ctrl Pts',(0.606118372661325,-9.35077522824464,
6.91215700200157));
#80613=CARTESIAN_POINT('Ctrl Pts',(0.697093125253195,-9.34436289766654,
6.91371106324044));
#80614=CARTESIAN_POINT('Ctrl Pts',(0.735344259706685,-9.34143059753206,
6.9143618910544));
#80615=CARTESIAN_POINT('Ctrl Pts',(0.836137512132898,-9.33308094233698,
6.91607065001953));
#80616=CARTESIAN_POINT('Ctrl Pts',(0.898645087838587,-9.32726984962665,
6.91712422029971));
#80617=CARTESIAN_POINT('Ctrl Pts',(1.03929038806274,-9.31276762991967,6.91948527949529));
#80618=CARTESIAN_POINT('Ctrl Pts',(1.11738669302317,-9.30372035554436,6.92078967664173));
#80619=CARTESIAN_POINT('Ctrl Pts',(1.38466822944068,-9.26934244925843,6.92524301788084));
#80620=CARTESIAN_POINT('Ctrl Pts',(1.57318859254317,-9.23921497825125,6.92836612083579));
#80621=CARTESIAN_POINT('Ctrl Pts',(1.90277358341188,-9.17616335895287,6.93386709901732));
#80622=CARTESIAN_POINT('Ctrl Pts',(2.04424103698314,-9.14568749830089,6.93624151186545));
#80623=CARTESIAN_POINT('Ctrl Pts',(2.34674941250458,-9.07314928903009,6.94137589001569));
#80624=CARTESIAN_POINT('Ctrl Pts',(2.50749050614896,-9.03004772700305,6.94413953779842));
#80625=CARTESIAN_POINT('Ctrl Pts',(2.75091014398372,-8.95777541339391,6.94839897024734));
#80626=CARTESIAN_POINT('Ctrl Pts',(2.83446874477871,-8.93168706726343,6.94987455007341));
#80627=CARTESIAN_POINT('Ctrl Pts',(2.99389692452198,-8.87944841323074,6.95271776789886));
#80628=CARTESIAN_POINT('Ctrl Pts',(3.06982027395367,-8.85348667859727,6.954084027142));
#80629=CARTESIAN_POINT('Ctrl Pts',(3.25357576202563,-8.7880041922735,6.95742149962108));
#80630=CARTESIAN_POINT('Ctrl Pts',(3.36103278337511,-8.74747000299489,6.95939929650354));
#80631=CARTESIAN_POINT('Ctrl Pts',(3.53628416320187,-8.67765676063081,6.96266717501181));
#80632=CARTESIAN_POINT('Ctrl Pts',(3.60452576168345,-8.64953331398509,6.96395033874386));
#80633=CARTESIAN_POINT('Ctrl Pts',(3.8865367723986,-8.52939500478843,6.9692954103017));
#80634=CARTESIAN_POINT('Ctrl Pts',(4.09717290202295,-8.43023849353389,6.97339175267438));
#80635=CARTESIAN_POINT('Ctrl Pts',(4.42356175811659,-8.26146685409431,6.97984933135097));
#80636=CARTESIAN_POINT('Ctrl Pts',(4.54187739601849,-8.19701671408261,6.98221346224923));
#80637=CARTESIAN_POINT('Ctrl Pts',(4.74597502743253,-8.0800624820426,6.98631299854088));
#80638=CARTESIAN_POINT('Ctrl Pts',(4.83237813562274,-8.02868671168288,6.98805532770705));
#80639=CARTESIAN_POINT('Ctrl Pts',(4.95875878869117,-7.95076073072815,6.99060546671732));
#80640=CARTESIAN_POINT('Ctrl Pts',(4.99938575423751,-7.92527772480189,6.99142549233828));
#80641=CARTESIAN_POINT('Ctrl Pts',(5.07746044682174,-7.87546661841097,6.99300050630066));
#80642=CARTESIAN_POINT('Ctrl Pts',(5.11493337697594,-7.85118052249396,6.99375596452528));
#80643=CARTESIAN_POINT('Ctrl Pts',(5.21942339510289,-7.78239524545958,6.99586302392873));
#80644=CARTESIAN_POINT('Ctrl Pts',(5.28604325525921,-7.73729946991745,6.99720709272916));
#80645=CARTESIAN_POINT('Ctrl Pts',(5.68943589982201,-7.45659621182798,7.00537358316229));
#80646=CARTESIAN_POINT('Ctrl Pts',(6.01098747014009,-7.19989863398696,7.01202482010297));
#80647=CARTESIAN_POINT('Ctrl Pts',(6.42387333014739,-6.82329049339524,7.02127026093402));
#80648=CARTESIAN_POINT('Ctrl Pts',(6.53072688329048,-6.72108978648761,7.02373148963341));
#80649=CARTESIAN_POINT('Ctrl Pts',(6.69511957194784,-6.55623214210041,7.02764170698326));
#80650=CARTESIAN_POINT('Ctrl Pts',(6.75430037471817,-6.49524690761594,7.02907583600945));
#80651=CARTESIAN_POINT('Ctrl Pts',(6.86856800093705,-6.37424453053456,7.03189915001919));
#80652=CARTESIAN_POINT('Ctrl Pts',(6.92371796196137,-6.31429721067544,7.03328761009658));
#80653=CARTESIAN_POINT('Ctrl Pts',(7.06070612409384,-6.16143991978158,7.03680318679329));
#80654=CARTESIAN_POINT('Ctrl Pts',(7.14149743609768,-6.06761296595567,7.03893876246352));
#80655=CARTESIAN_POINT('Ctrl Pts',(7.27326137161348,-5.90831036327752,7.04252636774702));
#80656=CARTESIAN_POINT('Ctrl Pts',(7.32526637198046,-5.84370900020765,7.04397107732937));
#80657=CARTESIAN_POINT('Ctrl Pts',(7.55819068929469,-5.54637118333083,7.05057077721524));
#80658=CARTESIAN_POINT('Ctrl Pts',(7.72892242561306,-5.30586820443467,7.05577791298135));
#80659=CARTESIAN_POINT('Ctrl Pts',(7.95834876750401,-4.94805422640624,7.06321600005997));
#80660=CARTESIAN_POINT('Ctrl Pts',(8.02637016214393,-4.83693476344721,7.06548437821871));
#80661=CARTESIAN_POINT('Ctrl Pts',(8.11902851726629,-4.67822867553789,7.06864948910207));
#80662=CARTESIAN_POINT('Ctrl Pts',(8.14560814460253,-4.63179399118876,7.06956669535995));
#80663=CARTESIAN_POINT('Ctrl Pts',(8.19241668858898,-4.54837014446286,7.07119709045023));
#80664=CARTESIAN_POINT('Ctrl Pts',(8.21279634348789,-4.51146743210387,7.07191210741618));
#80665=CARTESIAN_POINT('Ctrl Pts',(8.26418950128087,-4.41690427309674,7.07372942580617));
#80666=CARTESIAN_POINT('Ctrl Pts',(8.29484899126454,-4.35905399279979,7.0748273572166));
#80667=CARTESIAN_POINT('Ctrl Pts',(8.41997977847145,-4.11684785274186,7.07937580197943));
#80668=CARTESIAN_POINT('Ctrl Pts',(8.50893112498655,-3.92970575533234,7.08277578363099));
#80669=CARTESIAN_POINT('Ctrl Pts',(8.72248789516042,-3.43908837073114,7.09154828466975));
#80670=CARTESIAN_POINT('Ctrl Pts',(8.83749408574656,-3.13174419156877,7.09691498034088));
#80671=CARTESIAN_POINT('Ctrl Pts',(8.96628318117,-2.72348724385437,7.1040642157495));
#80672=CARTESIAN_POINT('Ctrl Pts',(8.99488210780268,-2.62749170408588,7.10574588558639));
#80673=CARTESIAN_POINT('Ctrl Pts',(9.043249995996,-2.45508462859423,7.10877064023812));
#80674=CARTESIAN_POINT('Ctrl Pts',(9.0636029571511,-2.37884686879552,7.11010970740197));
#80675=CARTESIAN_POINT('Ctrl Pts',(9.1064612874211,-2.20976749098957,7.11308388486321));
#80676=CARTESIAN_POINT('Ctrl Pts',(9.12851471293581,-2.11682040351344,7.11472179836349));
#80677=CARTESIAN_POINT('Ctrl Pts',(9.20545767216222,-1.76893611265383,7.12086327856555));
#80678=CARTESIAN_POINT('Ctrl Pts',(9.251118673416,-1.51208077544671,7.12542316841205));
#80679=CARTESIAN_POINT('Ctrl Pts',(9.3265428172602,-0.953404045537311,7.13532760134473));
#80680=CARTESIAN_POINT('Ctrl Pts',(9.35249213363519,-0.65136124541213,7.14067520388304));
#80681=CARTESIAN_POINT('Ctrl Pts',(9.36571616415753,-0.296142938690236,
7.14680846368754));
#80682=CARTESIAN_POINT('Ctrl Pts',(9.36722805303101,-0.243677093503678,
7.14771018482407));
#80683=CARTESIAN_POINT('Ctrl Pts',(9.36916215981244,-0.148911549578908,
7.14932979358075));
#80684=CARTESIAN_POINT('Ctrl Pts',(9.36973890572044,-0.106616515382582,
7.15004926455041));
#80685=CARTESIAN_POINT('Ctrl Pts',(9.37040951820078,-0.00892101066067758,
7.15170307109131));
#80686=CARTESIAN_POINT('Ctrl Pts',(9.37029849203117,0.0464791618998744,
7.15263518081541));
#80687=CARTESIAN_POINT('Ctrl Pts',(9.36783909579904,0.272675564747029,7.15642301810922));
#80688=CARTESIAN_POINT('Ctrl Pts',(9.36131206417663,0.443393806085254,7.15924063211639));
#80689=CARTESIAN_POINT('Ctrl Pts',(9.32358430163558,1.01807143864961,7.1687017247207));
#80690=CARTESIAN_POINT('Ctrl Pts',(9.27086014771178,1.42015699321713,7.17530005573792));
#80691=CARTESIAN_POINT('Ctrl Pts',(9.17412768401483,1.90937825200955,7.18364564360164));
#80692=CARTESIAN_POINT('Ctrl Pts',(9.15459945514986,2.00091300018584,7.18521993623567));
#80693=CARTESIAN_POINT('Ctrl Pts',(9.11605900845249,2.16916993297434,7.18814004570542));
#80694=CARTESIAN_POINT('Ctrl Pts',(9.09744094893623,2.24597377333545,7.18948316243218));
#80695=CARTESIAN_POINT('Ctrl Pts',(9.05240222169807,2.42201218012098,7.19258606800701));
#80696=CARTESIAN_POINT('Ctrl Pts',(9.02531737331991,2.52106628692512,7.19435004691618));
#80697=CARTESIAN_POINT('Ctrl Pts',(8.9635674239314,2.73313245972967,7.19816522765187));
#80698=CARTESIAN_POINT('Ctrl Pts',(8.92838080980068,2.84597435489088,7.20021927321259));
#80699=CARTESIAN_POINT('Ctrl Pts',(8.80729820765775,3.20990608009049,7.20691534830602));
#80700=CARTESIAN_POINT('Ctrl Pts',(8.71286968855318,3.45801967668251,7.21159540621311));
#80701=CARTESIAN_POINT('Ctrl Pts',(8.54214442014896,3.85501949070504,7.21917725123089));
#80702=CARTESIAN_POINT('Ctrl Pts',(8.47216981388657,4.00646296343008,7.22209155546404));
#80703=CARTESIAN_POINT('Ctrl Pts',(8.37389306850937,4.20505659358886,7.22591073862778));
#80704=CARTESIAN_POINT('Ctrl Pts',(8.34916584597256,4.2539412046895,7.2268505885105));
#80705=CARTESIAN_POINT('Ctrl Pts',(8.30655843588268,4.33637137507222,7.22843322686966));
#80706=CARTESIAN_POINT('Ctrl Pts',(8.28890031029224,4.37002990860614,7.22907873592303));
#80707=CARTESIAN_POINT('Ctrl Pts',(8.24344661195211,4.45540345403634,7.23071445338078));
#80708=CARTESIAN_POINT('Ctrl Pts',(8.21536893371334,4.50696630644274,7.23170109548439));
#80709=CARTESIAN_POINT('Ctrl Pts',(8.15199867269176,4.62078165902737,7.23387954894929));
#80710=CARTESIAN_POINT('Ctrl Pts',(8.1164737920253,4.6829006729324,7.23506894932531));
#80711=CARTESIAN_POINT('Ctrl Pts',(7.99994097880888,4.88136036543957,7.23887877248502));
#80712=CARTESIAN_POINT('Ctrl Pts',(7.91618221466055,5.01605362639661,7.24148005582004));
#80713=CARTESIAN_POINT('Ctrl Pts',(7.65488875594652,5.41338410937503,7.24927550520336));
#80714=CARTESIAN_POINT('Ctrl Pts',(7.46740711201449,5.66920451927245,7.25446603737995));
#80715=CARTESIAN_POINT('Ctrl Pts',(7.20426399547315,5.99250736618144,7.26142608067284));
#80716=CARTESIAN_POINT('Ctrl Pts',(7.13996925883983,6.0689705197547,7.26310289678615));
#80717=CARTESIAN_POINT('Ctrl Pts',(7.02268353417167,6.20400972765649,7.26612339065504));
#80718=CARTESIAN_POINT('Ctrl Pts',(6.9701512277802,6.26297154314259,7.26746311932829));
#80719=CARTESIAN_POINT('Ctrl Pts',(6.85322076775757,6.39091971759516,7.27041779050818));
#80720=CARTESIAN_POINT('Ctrl Pts',(6.78851303041146,6.45961148272738,7.2720353072796));
#80721=CARTESIAN_POINT('Ctrl Pts',(6.5572011618538,6.69785014332778,7.27775692048023));
#80722=CARTESIAN_POINT('Ctrl Pts',(6.38519499485934,6.86202359131373,7.28190638246082));
#80723=CARTESIAN_POINT('Ctrl Pts',(5.9681271086905,7.23082537403374,7.291679412853));
#80724=CARTESIAN_POINT('Ctrl Pts',(5.71848225455219,7.42982756564254,7.29731836284638));
#80725=CARTESIAN_POINT('Ctrl Pts',(5.40800898609829,7.6523843975673,7.30392053059611));
#80726=CARTESIAN_POINT('Ctrl Pts',(5.35647515706879,7.68854486102214,7.30500323169772));
#80727=CARTESIAN_POINT('Ctrl Pts',(5.26971096723597,7.74813014467398,7.30680173562611));
#80728=CARTESIAN_POINT('Ctrl Pts',(5.23467942270256,7.77184056545524,7.30752125051269));
#80729=CARTESIAN_POINT('Ctrl Pts',(5.15341940515213,7.82604114853768,7.30917472462255));
#80730=CARTESIAN_POINT('Ctrl Pts',(5.10707889812488,7.85636027504752,7.31010646280213));
#80731=CARTESIAN_POINT('Ctrl Pts',(4.9170074215257,7.97832564293945,7.31388810734709));
#80732=CARTESIAN_POINT('Ctrl Pts',(4.77105673647798,8.06645275232094,7.31670005968695));
#80733=CARTESIAN_POINT('Ctrl Pts',(4.51335545110058,8.21261432760951,7.32156719322873));
#80734=CARTESIAN_POINT('Ctrl Pts',(4.40271363731969,8.27245488700144,7.32362653531074));
#80735=CARTESIAN_POINT('Ctrl Pts',(4.29092658438921,8.33003806173069,7.32568828984052));
#80736=CARTESIAN_POINT('Origin',(0.,0.,2.15141010809499));
#80737=CARTESIAN_POINT('',(4.2909266557441,8.33003802497472,8.52320208943219));
#80738=CARTESIAN_POINT('',(4.29124604933685,8.33065733261336,8.3257038672742));
#80739=CARTESIAN_POINT('',(4.29092662815669,8.33003803918541,2.15141010809499));
#80740=CARTESIAN_POINT('',(-9.37091712982845,0.000108538499879093,7.84858856853279));
#80741=CARTESIAN_POINT('Ctrl Pts',(4.2909266557441,8.33003802497472,8.52320208943219));
#80742=CARTESIAN_POINT('Ctrl Pts',(4.36344197094789,8.29268430605715,8.52184882563512));
#80743=CARTESIAN_POINT('Ctrl Pts',(4.43547931258882,8.25437864654634,8.52049018201438));
#80744=CARTESIAN_POINT('Ctrl Pts',(4.58991690527409,8.16965043141316,8.5175432457802));
#80745=CARTESIAN_POINT('Ctrl Pts',(4.67212074926457,8.12291899616669,8.51595321555757));
#80746=CARTESIAN_POINT('Ctrl Pts',(4.82164273272179,8.03489764252445,8.51301871480337));
#80747=CARTESIAN_POINT('Ctrl Pts',(4.88917329138468,7.99398544287827,8.51167714122255));
#80748=CARTESIAN_POINT('Ctrl Pts',(5.04220741846923,7.89860779762343,8.50859865202764));
#80749=CARTESIAN_POINT('Ctrl Pts',(5.12736031653314,7.84359846669364,8.50685779957073));
#80750=CARTESIAN_POINT('Ctrl Pts',(5.3079575713716,7.72273357330122,8.50310550189753));
#80751=CARTESIAN_POINT('Ctrl Pts',(5.40310608046931,7.65646602675577,8.50109142123788));
#80752=CARTESIAN_POINT('Ctrl Pts',(5.70184795087703,7.44006029150815,8.4946539704502));
#80753=CARTESIAN_POINT('Ctrl Pts',(5.90060290481796,7.28343683428866,8.49019599922936));
#80754=CARTESIAN_POINT('Ctrl Pts',(6.2258919485955,7.00503773270286,8.4826782468142));
#80755=CARTESIAN_POINT('Ctrl Pts',(6.35578617798489,6.8873991117217,8.47961215822225));
#80756=CARTESIAN_POINT('Ctrl Pts',(6.52118828560187,6.72893661015646,8.47565778645712));
#80757=CARTESIAN_POINT('Ctrl Pts',(6.55974902551487,6.69135093226922,8.47473223207736));
#80758=CARTESIAN_POINT('Ctrl Pts',(6.62812929513128,6.62354055920766,8.47308603464598));
#80759=CARTESIAN_POINT('Ctrl Pts',(6.65807138177038,6.59344166474343,8.47236357658209));
#80760=CARTESIAN_POINT('Ctrl Pts',(6.72572691118265,6.52450100814893,8.47072783629683));
#80761=CARTESIAN_POINT('Ctrl Pts',(6.76331028640827,6.4855338929692,8.46981650914498));
#80762=CARTESIAN_POINT('Ctrl Pts',(6.9062406769936,6.33474749016277,8.46633567537435));
#80763=CARTESIAN_POINT('Ctrl Pts',(7.00916981038996,6.22066916677316,8.46379682500955));
#80764=CARTESIAN_POINT('Ctrl Pts',(7.37902952436973,5.78990634753019,8.45445844636285));
#80765=CARTESIAN_POINT('Ctrl Pts',(7.6276837256657,5.45816211997136,8.44772407548045));
#80766=CARTESIAN_POINT('Ctrl Pts',(7.90667951235207,5.0294614370168,8.4391748526069));
#80767=CARTESIAN_POINT('Ctrl Pts',(7.95850792929903,4.94704100826315,8.43753901755185));
#80768=CARTESIAN_POINT('Ctrl Pts',(8.04997800265542,4.7964214357382,8.43456057440645));
#80769=CARTESIAN_POINT('Ctrl Pts',(8.09006084931744,4.72850080397772,8.4332214269191));
#80770=CARTESIAN_POINT('Ctrl Pts',(8.17807955769171,4.57495655410679,8.43020191499276));
#80771=CARTESIAN_POINT('Ctrl Pts',(8.22553745318002,4.48906964382114,8.42851824058472));
#80772=CARTESIAN_POINT('Ctrl Pts',(8.32352900955655,4.30495624848496,8.42492024954387));
#80773=CARTESIAN_POINT('Ctrl Pts',(8.37369245513698,4.20654942477857,8.42300378453386));
#80774=CARTESIAN_POINT('Ctrl Pts',(8.52100077415318,3.90448909675622,8.41714562724172));
#80775=CARTESIAN_POINT('Ctrl Pts',(8.61254039109112,3.69819374111411,8.41317634492159));
#80776=CARTESIAN_POINT('Ctrl Pts',(8.75561028093878,3.34156255193806,8.40642185749983));
#80777=CARTESIAN_POINT('Ctrl Pts',(8.81092770248506,3.19285214677145,8.40363659706919));
#80778=CARTESIAN_POINT('Ctrl Pts',(8.89232045407592,2.95578876156814,8.39927466166068));
#80779=CARTESIAN_POINT('Ctrl Pts',(8.92091457168261,2.8683328841694,8.39768208076638));
#80780=CARTESIAN_POINT('Ctrl Pts',(8.96204389721282,2.73596889592536,8.39530334269566));
#80781=CARTESIAN_POINT('Ctrl Pts',(8.97553952944504,2.69136522655317,8.39450713169773));
#80782=CARTESIAN_POINT('Ctrl Pts',(9.00161047138237,2.60282204866018,8.39293844633724));
#80783=CARTESIAN_POINT('Ctrl Pts',(9.01419815601723,2.55888751369075,8.3921658634987));
#80784=CARTESIAN_POINT('Ctrl Pts',(9.04972695784281,2.43136585640224,8.38993794903868));
#80785=CARTESIAN_POINT('Ctrl Pts',(9.07183037012952,2.34755015603192,8.38849160001895));
#80786=CARTESIAN_POINT('Ctrl Pts',(9.15516214312644,2.01278689871448,8.3827668432091));
#80787=CARTESIAN_POINT('Ctrl Pts',(9.20716567911062,1.75966070518796,8.37855084839455));
#80788=CARTESIAN_POINT('Ctrl Pts',(9.28851398988429,1.25965616908904,8.37024058491939));
#80789=CARTESIAN_POINT('Ctrl Pts',(9.31862770210545,1.01311551308332,8.36615123785798));
#80790=CARTESIAN_POINT('Ctrl Pts',(9.34683353284748,0.669088163298444,8.36038095390027));
#80791=CARTESIAN_POINT('Ctrl Pts',(9.35325332384938,0.572388209463317,8.35875245665025));
#80792=CARTESIAN_POINT('Ctrl Pts',(9.36217511024265,0.396840452050202,8.35578123035131));
#80793=CARTESIAN_POINT('Ctrl Pts',(9.36518359141979,0.318027364628808,8.3544418722678));
#80794=CARTESIAN_POINT('Ctrl Pts',(9.36971341789963,0.140626475176787,8.35141395236109));
#80795=CARTESIAN_POINT('Ctrl Pts',(9.37067438553663,0.0420337402154264,
8.34972198944694));
#80796=CARTESIAN_POINT('Ctrl Pts',(9.36840230577147,-0.334402311027361,
8.34322705920681));
#80797=CARTESIAN_POINT('Ctrl Pts',(9.35436783476926,-0.612035926906702,
8.33835992751789));
#80798=CARTESIAN_POINT('Ctrl Pts',(9.30239725441764,-1.15757302214544,8.32872695647232));
#80799=CARTESIAN_POINT('Ctrl Pts',(9.26515783328865,-1.42527917465293,8.32396711170294));
#80800=CARTESIAN_POINT('Ctrl Pts',(9.20535084655738,-1.75124300259456,8.31824260680378));
#80801=CARTESIAN_POINT('Ctrl Pts',(9.19370751294297,-1.8113747412928,8.31718978853459));
#80802=CARTESIAN_POINT('Ctrl Pts',(9.17304752706486,-1.9127375505105,8.31542285344433));
#80803=CARTESIAN_POINT('Ctrl Pts',(9.16434036909686,-1.95402955044761,8.31470537056174));
#80804=CARTESIAN_POINT('Ctrl Pts',(9.14328656651823,-2.05063594667606,8.31303228415601));
#80805=CARTESIAN_POINT('Ctrl Pts',(9.13071645508904,-2.10589982197977,8.31207917613357));
#80806=CARTESIAN_POINT('Ctrl Pts',(9.07267616193807,-2.35077695590852,8.30786735201178));
#80807=CARTESIAN_POINT('Ctrl Pts',(9.02179517913297,-2.53905834164524,8.30465860065171));
#80808=CARTESIAN_POINT('Ctrl Pts',(8.85652030319598,-3.0826794403061,8.29533564212096));
#80809=CARTESIAN_POINT('Ctrl Pts',(8.72672904118709,-3.43293814656882,8.28924287155239));
#80810=CARTESIAN_POINT('Ctrl Pts',(8.5380804245009,-3.86158197994939,8.28140962055638));
#80811=CARTESIAN_POINT('Ctrl Pts',(8.49844117525268,-3.94805398369551,8.27981034378085));
#80812=CARTESIAN_POINT('Ctrl Pts',(8.42384128408788,-4.10446015662358,8.27687997532733));
#80813=CARTESIAN_POINT('Ctrl Pts',(8.38930876311664,-4.17458903380878,8.27555201410437));
#80814=CARTESIAN_POINT('Ctrl Pts',(8.30851876247877,-4.33360592558777,8.27250767373788));
#80815=CARTESIAN_POINT('Ctrl Pts',(8.26170486233959,-4.4222004754789,8.27078746473928));
#80816=CARTESIAN_POINT('Ctrl Pts',(8.07599428318759,-4.76040908811691,8.26412730852763));
#80817=CARTESIAN_POINT('Ctrl Pts',(7.9271326481714,-5.00437260267519,8.25911956003787));
#80818=CARTESIAN_POINT('Ctrl Pts',(7.62473444566546,-5.45252510732725,8.24961490153297));
#80819=CARTESIAN_POINT('Ctrl Pts',(7.47353908490545,-5.657987218979,8.24512594071311));
#80820=CARTESIAN_POINT('Ctrl Pts',(7.27497461600892,-5.90595105868186,8.23963611495651));
#80821=CARTESIAN_POINT('Ctrl Pts',(7.23530686270483,-5.95448135438398,8.23855823669244));
#80822=CARTESIAN_POINT('Ctrl Pts',(7.16806947125792,-6.03507687142065,8.23676487614228));
#80823=CARTESIAN_POINT('Ctrl Pts',(7.14076439062226,-6.06735994665542,8.23604573758916));
#80824=CARTESIAN_POINT('Ctrl Pts',(7.07706629952926,-6.14164522997826,8.23438934499278));
#80825=CARTESIAN_POINT('Ctrl Pts',(7.0405163356843,-6.18351059552723,8.23345435403023));
#80826=CARTESIAN_POINT('Ctrl Pts',(6.88827333928311,-6.35479415544751,8.22961733414545));
#80827=CARTESIAN_POINT('Ctrl Pts',(6.7693670927049,-6.48131066029187,8.22675469946));
#80828=CARTESIAN_POINT('Ctrl Pts',(6.36420265300372,-6.88908626361945,8.21731285399485));
#80829=CARTESIAN_POINT('Ctrl Pts',(6.0634004440858,-7.15526100348339,8.21077548697879));
#80830=CARTESIAN_POINT('Ctrl Pts',(5.67237492260607,-7.45885688571624,8.20249151435682));
#80831=CARTESIAN_POINT('Ctrl Pts',(5.5974259745648,-7.51526484628704,8.20091380304));
#80832=CARTESIAN_POINT('Ctrl Pts',(5.45781014933223,-7.61709495893508,8.19799060660632));
#80833=CARTESIAN_POINT('Ctrl Pts',(5.39339120674733,-7.66284271643219,8.19664786457746));
#80834=CARTESIAN_POINT('Ctrl Pts',(5.24417981113299,-7.76599294025426,8.19355048836432));
#80835=CARTESIAN_POINT('Ctrl Pts',(5.15900963674238,-7.82283118418899,8.1917917211806));
#80836=CARTESIAN_POINT('Ctrl Pts',(5.02081980004225,-7.91181358980023,8.18895292658103));
#80837=CARTESIAN_POINT('Ctrl Pts',(4.9683827972286,-7.9448472679103,8.1878790989168));
#80838=CARTESIAN_POINT('Ctrl Pts',(4.76843333232829,-8.06805547216641,8.18379800555763));
#80839=CARTESIAN_POINT('Ctrl Pts',(4.61876299063875,-8.15466147443709,8.1807701591455));
#80840=CARTESIAN_POINT('Ctrl Pts',(4.40725426485434,-8.26935793309367,8.17654377344696));
#80841=CARTESIAN_POINT('Ctrl Pts',(4.34737749094334,-8.30099269539958,8.17535310312928));
#80842=CARTESIAN_POINT('Ctrl Pts',(4.22203950750026,-8.3654845279821,8.17287486611625));
#80843=CARTESIAN_POINT('Ctrl Pts',(4.15652528157499,-8.39822877633345,8.17158739559903));
#80844=CARTESIAN_POINT('Ctrl Pts',(3.93729722771659,-8.50460603218191,8.16731058557016));
#80845=CARTESIAN_POINT('Ctrl Pts',(3.78195867013653,-8.5748132403217,8.16433048423798));
#80846=CARTESIAN_POINT('Ctrl Pts',(3.57694454729628,-8.66081664725144,8.16049542308772));
#80847=CARTESIAN_POINT('Ctrl Pts',(3.52893143876956,-8.68049078148484,8.15960421196886));
#80848=CARTESIAN_POINT('Ctrl Pts',(3.44153601469506,-8.71545750289904,8.15799608526108));
#80849=CARTESIAN_POINT('Ctrl Pts',(3.40220906028954,-8.73088444262237,8.15727768980722));
#80850=CARTESIAN_POINT('Ctrl Pts',(3.31049794657761,-8.76614657546564,8.15561473079433));
#80851=CARTESIAN_POINT('Ctrl Pts',(3.2580376927825,-8.78577901206424,8.15467252319907));
#80852=CARTESIAN_POINT('Ctrl Pts',(3.03517493625877,-8.86691134095931,8.15070214284174));
#80853=CARTESIAN_POINT('Ctrl Pts',(2.86318342954323,-8.92393325100653,8.14771695942125));
#80854=CARTESIAN_POINT('Ctrl Pts',(2.31509453134558,-9.08816860317451,8.13832288761082));
#80855=CARTESIAN_POINT('Ctrl Pts',(1.93388536658853,-9.1768490510491,8.1319476455794));
#80856=CARTESIAN_POINT('Ctrl Pts',(1.45522563313312,-9.25704058909419,8.12382771717759));
#80857=CARTESIAN_POINT('Ctrl Pts',(1.3619680911812,-9.27122025278297,8.1222414279016));
#80858=CARTESIAN_POINT('Ctrl Pts',(1.19027088630096,-9.29468000106789,8.11931038611918));
#80859=CARTESIAN_POINT('Ctrl Pts',(1.11189733835005,-9.30438097781153,8.11796848397056));
#80860=CARTESIAN_POINT('Ctrl Pts',(0.932359803220728,-9.32430304440704,
8.1148844139126));
#80861=CARTESIAN_POINT('Ctrl Pts',(0.831133342483466,-9.33387054569329,
8.11313825102579));
#80862=CARTESIAN_POINT('Ctrl Pts',(0.442755711045977,-9.36421022784628,
8.10641114208985));
#80863=CARTESIAN_POINT('Ctrl Pts',(0.154860154632144,-9.37339228622713,
8.10136181471848));
#80864=CARTESIAN_POINT('Ctrl Pts',(-0.381054647071033,-9.36578488169506,
8.09193879344202));
#80865=CARTESIAN_POINT('Ctrl Pts',(-0.628873094677841,-9.35241402688368,
8.08757324481115));
#80866=CARTESIAN_POINT('Ctrl Pts',(-0.938642045194109,-9.32333156281816,
8.08219577092791));
#80867=CARTESIAN_POINT('Ctrl Pts',(-1.00135466709883,-9.31680466557163,
8.08111137969538));
#80868=CARTESIAN_POINT('Ctrl Pts',(-1.10603066796173,-9.30484127513795,
8.07931107214876));
#80869=CARTESIAN_POINT('Ctrl Pts',(-1.14803156983099,-9.29975260558561,
8.07859142419867));
#80870=CARTESIAN_POINT('Ctrl Pts',(-1.24485672754942,-9.28735569145919,
8.07693896429046));
#80871=CARTESIAN_POINT('Ctrl Pts',(-1.299653499173,-9.2798461632101,8.07600835875151));
#80872=CARTESIAN_POINT('Ctrl Pts',(-1.52201076864112,-9.24736544799571,
8.07224537313422));
#80873=CARTESIAN_POINT('Ctrl Pts',(-1.68894655055455,-9.21833739850408,
8.0694504687491));
#80874=CARTESIAN_POINT('Ctrl Pts',(-2.25401499833203,-9.10421361344375,
8.05997930775724));
#80875=CARTESIAN_POINT('Ctrl Pts',(-2.64734984596758,-8.99771237805869,
8.05334992761102));
#80876=CARTESIAN_POINT('Ctrl Pts',(-3.12095994443126,-8.83571913568714,
8.04497297683809));
#80877=CARTESIAN_POINT('Ctrl Pts',(-3.20895155063616,-8.80414411013471,
8.04340046948753));
#80878=CARTESIAN_POINT('Ctrl Pts',(-3.37043804657536,-8.74345348753124,
8.04048197126432));
#80879=CARTESIAN_POINT('Ctrl Pts',(-3.44406542247971,-8.71471427221091,
8.03913865808122));
#80880=CARTESIAN_POINT('Ctrl Pts',(-3.61263947844372,-8.64644418200136,
8.03603284573427));
#80881=CARTESIAN_POINT('Ctrl Pts',(-3.70731651126421,-8.60627475780529,
8.03426612644284));
#80882=CARTESIAN_POINT('Ctrl Pts',(-4.03045477290982,-8.46285228669809,
8.02815917910937));
#80883=CARTESIAN_POINT('Ctrl Pts',(-4.2554219813586,-8.3519948198441,8.02377066006185));
#80884=CARTESIAN_POINT('Ctrl Pts',(-4.72690093961701,-8.09566332968275,
8.01433991910639));
#80885=CARTESIAN_POINT('Ctrl Pts',(-4.97174627405936,-7.94764723766363,
8.00929659191953));
#80886=CARTESIAN_POINT('Ctrl Pts',(-5.26037647699285,-7.7545973298444,8.00329849319699));
#80887=CARTESIAN_POINT('Ctrl Pts',(-5.31097866911419,-7.72002888780753,
8.00224507953479));
#80888=CARTESIAN_POINT('Ctrl Pts',(-5.39584930750706,-7.66082086038846,
8.00047752265552));
#80889=CARTESIAN_POINT('Ctrl Pts',(-5.43029686549057,-7.63644170872416,
7.99976000647542));
#80890=CARTESIAN_POINT('Ctrl Pts',(-5.51059499199026,-7.57879520286504,
7.99808734753222));
#80891=CARTESIAN_POINT('Ctrl Pts',(-5.55631081479998,-7.54534320241335,
7.99713469446265));
#80892=CARTESIAN_POINT('Ctrl Pts',(-5.75750040289201,-7.39530512082562,
7.99293430486887));
#80893=CARTESIAN_POINT('Ctrl Pts',(-5.90962912229764,-7.27431322069525,
7.98973618890659));
#80894=CARTESIAN_POINT('Ctrl Pts',(-6.34323369383115,-6.90687090415995,
7.98041028633625));
#80895=CARTESIAN_POINT('Ctrl Pts',(-6.6138467242539,-6.64819603811661,7.97430444251095));
#80896=CARTESIAN_POINT('Ctrl Pts',(-6.93295524357736,-6.30434437472377,
7.96645789512514));
#80897=CARTESIAN_POINT('Ctrl Pts',(-6.99657200333878,-6.23366718320731,
7.96485916110048));
#80898=CARTESIAN_POINT('Ctrl Pts',(-7.11050704185395,-6.1031455026004,7.96192930296934));
#80899=CARTESIAN_POINT('Ctrl Pts',(-7.1611731543421,-6.04361600691027,7.96060130260048));
#80900=CARTESIAN_POINT('Ctrl Pts',(-7.26947812978644,-5.91309005670211,
7.95770636707091));
#80901=CARTESIAN_POINT('Ctrl Pts',(-7.32683457061386,-5.84186968545867,
7.95613728428783));
#80902=CARTESIAN_POINT('Ctrl Pts',(-7.4500513148117,-5.68419991882513,7.95268636796294));
#80903=CARTESIAN_POINT('Ctrl Pts',(-7.51546870559611,-5.59742113574193,
7.95080153032853));
#80904=CARTESIAN_POINT('Ctrl Pts',(-7.70725783249856,-5.3335799961464,7.94511784689496));
#80905=CARTESIAN_POINT('Ctrl Pts',(-7.82898836062203,-5.15323585511615,
7.94129335474755));
#80906=CARTESIAN_POINT('Ctrl Pts',(-8.0615447779394,-4.78141608851392,7.93358325209606));
#80907=CARTESIAN_POINT('Ctrl Pts',(-8.17208970304495,-4.58992312252395,
7.92970012495918));
#80908=CARTESIAN_POINT('Ctrl Pts',(-8.30562602027414,-4.33845787224488,
7.92477811090807));
#80909=CARTESIAN_POINT('Ctrl Pts',(-8.33491858038175,-4.28191225779835,
7.92368266465286));
#80910=CARTESIAN_POINT('Ctrl Pts',(-8.38132928579615,-4.19004114871298,
7.92192362156729));
#80911=CARTESIAN_POINT('Ctrl Pts',(-8.39880581361861,-4.15489907766306,
7.92125567970066));
#80912=CARTESIAN_POINT('Ctrl Pts',(-8.43796284742283,-4.07490486873738,
7.91974675409031));
#80913=CARTESIAN_POINT('Ctrl Pts',(-8.45950745328853,-4.02998763840995,
7.91890742129331));
#80914=CARTESIAN_POINT('Ctrl Pts',(-8.50614349197759,-3.93073650210613,
7.91706806703292));
#80915=CARTESIAN_POINT('Ctrl Pts',(-8.53107466250537,-3.87632966567911,
7.9160697544822));
#80916=CARTESIAN_POINT('Ctrl Pts',(-8.58000542909778,-3.76679001329679,
7.91407652877246));
#80917=CARTESIAN_POINT('Ctrl Pts',(-8.60399898131218,-3.71165754226315,
7.913081699358));
#80918=CARTESIAN_POINT('Ctrl Pts',(-8.7177206039368,-3.44331814532167,7.90827286668289));
#80919=CARTESIAN_POINT('Ctrl Pts',(-8.80006357837955,-3.22706889901276,
7.90449637741208));
#80920=CARTESIAN_POINT('Ctrl Pts',(-8.89542184456499,-2.94573867605372,
7.89961916779074));
#80921=CARTESIAN_POINT('Ctrl Pts',(-8.91586805364957,-2.88326255864508,
7.89853845417325));
#80922=CARTESIAN_POINT('Ctrl Pts',(-8.99045642810158,-2.64696477003479,
7.89445543032018));
#80923=CARTESIAN_POINT('Ctrl Pts',(-9.04018623481913,-2.47179324152747,
7.89143686062912));
#80924=CARTESIAN_POINT('Ctrl Pts',(-9.10669552311684,-2.2085482092304,7.88688602457657));
#80925=CARTESIAN_POINT('Ctrl Pts',(-9.12736635162331,-2.12150229303535,
7.88537904888074));
#80926=CARTESIAN_POINT('Ctrl Pts',(-9.16345501551127,-1.95922740405079,
7.88256353634716));
#80927=CARTESIAN_POINT('Ctrl Pts',(-9.1792007313458,-1.88407901763928,7.88125727615615));
#80928=CARTESIAN_POINT('Ctrl Pts',(-9.20907837175296,-1.73220821967822,
7.87861186992756));
#80929=CARTESIAN_POINT('Ctrl Pts',(-9.22317930783414,-1.65548578893449,
7.87727263446506));
#80930=CARTESIAN_POINT('Ctrl Pts',(-9.25443140584141,-1.47263068696262,
7.87407416891602));
#80931=CARTESIAN_POINT('Ctrl Pts',(-9.27071724724699,-1.36636138497699,
7.87220999662095));
#80932=CARTESIAN_POINT('Ctrl Pts',(-9.34183065442542,-0.842245272326605,
7.86299607335696));
#80933=CARTESIAN_POINT('Ctrl Pts',(-9.3702545781991,-0.421311037842885,
7.85551027891911));
#80934=CARTESIAN_POINT('Ctrl Pts',(-9.37024999944691,0.000101810025349425,
7.84820354462752));
#80935=CARTESIAN_POINT('Ctrl Pts',(4.2912416510688,8.33064876709114,7.52288355898769));
#80936=CARTESIAN_POINT('Ctrl Pts',(4.20195778222728,8.37670351717924,7.5245903173793));
#80937=CARTESIAN_POINT('Ctrl Pts',(2.72745792095632,9.10710664797032,7.55254268019657));
#80938=CARTESIAN_POINT('Ctrl Pts',(-0.499675883778941,9.74834161973542,
7.60674064743951));
#80939=CARTESIAN_POINT('Ctrl Pts',(-5.06811753411523,8.34230333806495,7.68547746071647));
#80940=CARTESIAN_POINT('Ctrl Pts',(-8.42125135251966,4.93582475191143,7.76421427399345));
#80941=CARTESIAN_POINT('Ctrl Pts',(-9.34226565951642,1.76620876927797,7.81858508438964));
#80942=CARTESIAN_POINT('Ctrl Pts',(-9.37098492218543,0.110745121527537,
7.84671029036016));
#80943=CARTESIAN_POINT('Ctrl Pts',(-9.37091942283365,0.000108561626433589,
7.84858989190502));
#80944=CARTESIAN_POINT('',(-9.36966470910927,0.000159076414697548,7.65141010809498));
#80945=CARTESIAN_POINT('Ctrl Pts',(4.2909265843892,8.33003806173069,7.32568828984052));
#80946=CARTESIAN_POINT('Ctrl Pts',(4.04231038249422,8.45810396756635,7.33027366504272));
#80947=CARTESIAN_POINT('Ctrl Pts',(3.78802961208239,8.57500427684227,7.33487502092718));
#80948=CARTESIAN_POINT('Ctrl Pts',(3.44216616747705,8.71560847533341,7.34112308215479));
#80949=CARTESIAN_POINT('Ctrl Pts',(3.35496931930943,8.74954397857682,7.34269693401101));
#80950=CARTESIAN_POINT('Ctrl Pts',(3.1932113224947,8.80972371093231,7.34561664634709));
#80951=CARTESIAN_POINT('Ctrl Pts',(3.11879807584541,8.83634137759264,7.34695981226159));
#80952=CARTESIAN_POINT('Ctrl Pts',(2.94690660549949,8.89538522789968,7.35006343717151));
#80953=CARTESIAN_POINT('Ctrl Pts',(2.84921408072378,8.9271560950038,7.35182809365274));
#80954=CARTESIAN_POINT('Ctrl Pts',(2.41202984221905,9.06142649974026,7.35972785094122));
#80955=CARTESIAN_POINT('Ctrl Pts',(2.0674046928293,9.14621089955978,7.36597449147862));
#80956=CARTESIAN_POINT('Ctrl Pts',(1.54373572909195,9.24392679224437,7.37533158121962));
#80957=CARTESIAN_POINT('Ctrl Pts',(1.36776737729832,9.27159723060213,7.37845092257349));
#80958=CARTESIAN_POINT('Ctrl Pts',(1.1283029973751,9.30228616297731,7.38262395395606));
#80959=CARTESIAN_POINT('Ctrl Pts',(1.06540851654924,9.30969925569383,7.38371322311891));
#80960=CARTESIAN_POINT('Ctrl Pts',(0.960358146850123,9.32100257412341,7.38551875525336));
#80961=CARTESIAN_POINT('Ctrl Pts',(0.918242476432774,9.32524570873777,7.38623880628932));
#80962=CARTESIAN_POINT('Ctrl Pts',(0.82122710244084,9.3343563580369,7.38788843042142));
#80963=CARTESIAN_POINT('Ctrl Pts',(0.766310433441146,9.33902515849433,7.3888158385484));
#80964=CARTESIAN_POINT('Ctrl Pts',(0.545313274224173,9.3558510248116,7.39252754668975));
#80965=CARTESIAN_POINT('Ctrl Pts',(0.378962827235572,9.364064419969,7.3952756680047));
#80966=CARTESIAN_POINT('Ctrl Pts',(-0.115911456643848,9.37528917672946,
7.403409727051));
#80967=CARTESIAN_POINT('Ctrl Pts',(-0.444468673421632,9.36546476760892,
7.40876317643165));
#80968=CARTESIAN_POINT('Ctrl Pts',(-0.899869561346608,9.32782535748185,
7.4163462339333));
#80969=CARTESIAN_POINT('Ctrl Pts',(-1.02767742426524,9.31461057237031,7.41849117757631));
#80970=CARTESIAN_POINT('Ctrl Pts',(-1.22856400102596,9.28965472692301,7.42189694485045));
#80971=CARTESIAN_POINT('Ctrl Pts',(-1.30184455291793,9.27966891558475,7.42314651584613));
#80972=CARTESIAN_POINT('Ctrl Pts',(-1.45628643463555,9.2567579597057,7.42579638976125));
#80973=CARTESIAN_POINT('Ctrl Pts',(-1.53741148303551,9.24363045551501,7.42719789851145));
#80974=CARTESIAN_POINT('Ctrl Pts',(-1.74521668542947,9.2071924583808,7.43081332670424));
#80975=CARTESIAN_POINT('Ctrl Pts',(-1.87160770360422,9.18233405583594,7.43303680161501));
#80976=CARTESIAN_POINT('Ctrl Pts',(-2.0836941816202,9.13606022976917,7.43680724505908));
#80977=CARTESIAN_POINT('Ctrl Pts',(-2.16967223638292,9.11602437016743,7.43834672457213));
#80978=CARTESIAN_POINT('Ctrl Pts',(-2.58880252693475,9.01208698865118,7.44589965795934));
#80979=CARTESIAN_POINT('Ctrl Pts',(-2.91745012382002,8.91112195831109,7.45198223345832));
#80980=CARTESIAN_POINT('Ctrl Pts',(-3.32265275109734,8.76181252309734,7.45949218176258));
#80981=CARTESIAN_POINT('Ctrl Pts',(-3.40506103552275,8.73011680338023,7.46101940279675));
#80982=CARTESIAN_POINT('Ctrl Pts',(-3.52968224276099,8.68015218954677,7.46332269446726));
#80983=CARTESIAN_POINT('Ctrl Pts',(-3.57222886162526,8.66272934715109,7.46410792884781));
#80984=CARTESIAN_POINT('Ctrl Pts',(-3.65736738427479,8.6271312214192,7.46567572799275));
#80985=CARTESIAN_POINT('Ctrl Pts',(-3.69995624188434,8.60895191735874,7.46645822350026));
#80986=CARTESIAN_POINT('Ctrl Pts',(-3.82514246705008,8.55441489141405,7.46875540663353));
#80987=CARTESIAN_POINT('Ctrl Pts',(-3.90735146798894,8.51717873477945,7.47026024603327));
#80988=CARTESIAN_POINT('Ctrl Pts',(-4.22743914431247,8.36658681106154,7.47612619328647));
#80989=CARTESIAN_POINT('Ctrl Pts',(-4.46103118718842,8.24440525488119,7.48042496285821));
#80990=CARTESIAN_POINT('Ctrl Pts',(-4.89511597159933,7.99349814615369,7.48865284328449));
#80991=CARTESIAN_POINT('Ctrl Pts',(-5.09646033428096,7.86665523414928,7.49257390672609));
#80992=CARTESIAN_POINT('Ctrl Pts',(-5.3725946549927,7.67764103538125,7.49816806471463));
#80993=CARTESIAN_POINT('Ctrl Pts',(-5.45157920589582,7.62176024934758,7.49979395664641));
#80994=CARTESIAN_POINT('Ctrl Pts',(-5.59335651221209,7.5181226706588,7.50276263987606));
#80995=CARTESIAN_POINT('Ctrl Pts',(-5.6564386459398,7.47077689232608,7.50410209212282));
#80996=CARTESIAN_POINT('Ctrl Pts',(-5.79715090731655,7.36236243650978,7.50713310109671));
#80997=CARTESIAN_POINT('Ctrl Pts',(-5.87442832954561,7.30085139044931,7.50882809213423));
#80998=CARTESIAN_POINT('Ctrl Pts',(-6.03686868546358,7.16730352242169,7.51245649857238));
#80999=CARTESIAN_POINT('Ctrl Pts',(-6.12174706937035,7.09494440054348,7.51439215570155));
#81000=CARTESIAN_POINT('Ctrl Pts',(-6.37817604354789,6.86830968935955,7.52035906903658));
#81001=CARTESIAN_POINT('Ctrl Pts',(-6.54533726029579,6.70920020582771,7.52441916490341));
#81002=CARTESIAN_POINT('Ctrl Pts',(-6.72675217328434,6.5232840568858,7.52898462028908));
#81003=CARTESIAN_POINT('Ctrl Pts',(-6.74695219512636,6.50238923509666,7.52949526148573));
#81004=CARTESIAN_POINT('Ctrl Pts',(-6.89592684480622,6.34684884561467,7.53327754072286));
#81005=CARTESIAN_POINT('Ctrl Pts',(-7.02075765590993,6.2084828725395,7.53653863198782));
#81006=CARTESIAN_POINT('Ctrl Pts',(-7.17769709367798,6.02373605563979,7.5407189900927));
#81007=CARTESIAN_POINT('Ctrl Pts',(-7.21362912281673,5.98065937289526,7.54168182995705));
#81008=CARTESIAN_POINT('Ctrl Pts',(-7.27589665129806,5.90463308437941,7.54335860006113));
#81009=CARTESIAN_POINT('Ctrl Pts',(-7.30240036867556,5.87182363525381,7.54407484151696));
#81010=CARTESIAN_POINT('Ctrl Pts',(-7.33053103196896,5.8365151125376,7.54483794075264));
#81011=CARTESIAN_POINT('Ctrl Pts',(-7.33237915578109,5.8341931563336,7.54488808880286));
#81012=CARTESIAN_POINT('Ctrl Pts',(-7.33639729808852,5.82913989505332,7.54499715047581));
#81013=CARTESIAN_POINT('Ctrl Pts',(-7.33856689512836,5.82640825528336,7.54505605811935));
#81014=CARTESIAN_POINT('Ctrl Pts',(-7.34219185163393,5.82183900251341,7.54515451446979));
#81015=CARTESIAN_POINT('Ctrl Pts',(-7.34364804774374,5.8200020539736,7.5451940748616));
#81016=CARTESIAN_POINT('Ctrl Pts',(-7.34601991394989,5.81700770709245,7.54525852619065));
#81017=CARTESIAN_POINT('Ctrl Pts',(-7.34693600013598,5.81585063859342,7.54528342288178));
#81018=CARTESIAN_POINT('Ctrl Pts',(-7.34839882210075,5.81400211479826,7.54532318420669));
#81019=CARTESIAN_POINT('Ctrl Pts',(-7.34894573370705,5.81331079872384,7.54533805125667));
#81020=CARTESIAN_POINT('Ctrl Pts',(-7.38547755100022,5.76711986478796,7.5463312070787));
#81021=CARTESIAN_POINT('Ctrl Pts',(-7.42103931452482,5.72128706704285,7.54730369962533));
#81022=CARTESIAN_POINT('Ctrl Pts',(-7.5059559935398,5.60972066953171,7.54964344589641));
#81023=CARTESIAN_POINT('Ctrl Pts',(-7.5548760579241,5.54366207093679,7.55100614761297));
#81024=CARTESIAN_POINT('Ctrl Pts',(-7.72537946250415,5.30697567989573,7.55582296682178));
#81025=CARTESIAN_POINT('Ctrl Pts',(-7.84210267372028,5.1329235927607,7.55924721209016));
#81026=CARTESIAN_POINT('Ctrl Pts',(-8.08698111497736,4.73989620406924,7.56684259534743));
#81027=CARTESIAN_POINT('Ctrl Pts',(-8.21227767944174,4.5193333985128,7.57101747848766));
#81028=CARTESIAN_POINT('Ctrl Pts',(-8.37290870071318,4.20777699009645,7.57687702529179));
#81029=CARTESIAN_POINT('Ctrl Pts',(-8.41600291666158,4.12090792871133,7.5785064710362));
#81030=CARTESIAN_POINT('Ctrl Pts',(-8.49057025217792,3.96454520034833,7.58143469815022));
#81031=CARTESIAN_POINT('Ctrl Pts',(-8.52255770216196,3.89530641101939,7.58272969404166));
#81032=CARTESIAN_POINT('Ctrl Pts',(-8.59152353711384,3.74110845307417,7.58561096833774));
#81033=CARTESIAN_POINT('Ctrl Pts',(-8.62809425907516,3.65597573154188,7.58719992463265));
#81034=CARTESIAN_POINT('Ctrl Pts',(-8.70385797463682,3.47213449309127,7.5906274480045));
#81035=CARTESIAN_POINT('Ctrl Pts',(-8.74264757763201,3.37327360933953,7.59246833312108));
#81036=CARTESIAN_POINT('Ctrl Pts',(-8.85198807294151,3.08003963825092,7.59791848456092));
#81037=CARTESIAN_POINT('Ctrl Pts',(-8.9177953093454,2.88396663022594,7.60155090967412));
#81038=CARTESIAN_POINT('Ctrl Pts',(-8.98972656973892,2.64354938814965,7.60596299562891));
#81039=CARTESIAN_POINT('Ctrl Pts',(-9.00209148657416,2.60113168335239,7.60673981165297));
#81040=CARTESIAN_POINT('Ctrl Pts',(-9.03704354801635,2.47799408069812,7.60898924156054));
#81041=CARTESIAN_POINT('Ctrl Pts',(-9.05884820454744,2.39705652330416,7.61046080176516));
#81042=CARTESIAN_POINT('Ctrl Pts',(-9.1109329989659,2.19285080281186,7.61414954394344));
#81043=CARTESIAN_POINT('Ctrl Pts',(-9.13979996608033,2.06923934640825,7.61636072737865));
#81044=CARTESIAN_POINT('Ctrl Pts',(-9.17768809670054,1.89069231410202,7.61950774854431));
#81045=CARTESIAN_POINT('Ctrl Pts',(-9.1887449292979,1.83620338479388,7.62046190085535));
#81046=CARTESIAN_POINT('Ctrl Pts',(-9.2073404579694,1.74018615122084,7.62213041069662));
#81047=CARTESIAN_POINT('Ctrl Pts',(-9.21508470499457,1.6986995128911,7.62284697773679));
#81048=CARTESIAN_POINT('Ctrl Pts',(-9.23010239968762,1.61512202475682,7.62428213940653));
#81049=CARTESIAN_POINT('Ctrl Pts',(-9.23736881828136,1.57303108274252,7.62500075387933));
#81050=CARTESIAN_POINT('Ctrl Pts',(-9.25454643839661,1.46930338917469,7.62676296202449));
#81051=CARTESIAN_POINT('Ctrl Pts',(-9.26412995946588,1.40761441638011,7.62780342632758));
#81052=CARTESIAN_POINT('Ctrl Pts',(-9.33777378647577,0.900192111112405,
7.63631450621329));
#81053=CARTESIAN_POINT('Ctrl Pts',(-9.37024262317214,0.450467170292491,
7.64359007600784));
#81054=CARTESIAN_POINT('Ctrl Pts',(-9.37024999874316,0.0001534728895565,
7.65107226318331));
#81055=CARTESIAN_POINT('Ctrl Pts',(-9.36966470910927,0.000159076414697548,
7.65141010809498));
#81056=CARTESIAN_POINT('Ctrl Pts',(-9.36906894256188,-0.965940399241459,
7.66781681340257));
#81057=CARTESIAN_POINT('Ctrl Pts',(-8.98250254660737,-3.47796327412567,
7.71046912313581));
#81058=CARTESIAN_POINT('Ctrl Pts',(-6.77274903485361,-7.02920412114798,
7.77936703729473));
#81059=CARTESIAN_POINT('Ctrl Pts',(-2.62336437052269,-9.40201039381186,
7.8581038505717));
#81060=CARTESIAN_POINT('Ctrl Pts',(2.15508922207328,-9.52026420383269,7.93684066384868));
#81061=CARTESIAN_POINT('Ctrl Pts',(6.41676379514821,-7.35560891178627,8.01557747712564));
#81062=CARTESIAN_POINT('Ctrl Pts',(9.13973228190865,-3.42711743027742,8.09431429040262));
#81063=CARTESIAN_POINT('Ctrl Pts',(9.67104121278963,1.32317872050558,8.17305110367959));
#81064=CARTESIAN_POINT('Ctrl Pts',(7.91977215059093,5.66570957463458,8.25018096263681));
#81065=CARTESIAN_POINT('Ctrl Pts',(5.58015555167917,7.66584979211291,8.30106521716837));
#81066=CARTESIAN_POINT('Ctrl Pts',(4.29124604933307,8.33065733261531,8.32570386727427));
#81067=CARTESIAN_POINT('Origin',(0.,0.,2.15141010809499));
#81068=CARTESIAN_POINT('',(4.29092667702531,8.33003801401246,9.52315240206829));
#81069=CARTESIAN_POINT('',(4.29092661458801,8.33003804617484,9.32538978630507));
#81070=CARTESIAN_POINT('',(4.29092662815669,8.33003803918541,2.15141010809499));
#81071=CARTESIAN_POINT('Ctrl Pts',(4.29092667702531,8.33003801401246,9.52315240206829));
#81072=CARTESIAN_POINT('Ctrl Pts',(4.53655035743086,8.20351359707842,9.51833436278683));
#81073=CARTESIAN_POINT('Ctrl Pts',(4.77651276604139,8.0661588380477,9.51346043102322));
#81074=CARTESIAN_POINT('Ctrl Pts',(5.15459381020808,7.82693962096863,9.50560935836044));
#81075=CARTESIAN_POINT('Ctrl Pts',(5.29655681628916,7.73157858064885,9.50262087595));
#81076=CARTESIAN_POINT('Ctrl Pts',(5.48096469357036,7.60024219273754,9.49871858682182));
#81077=CARTESIAN_POINT('Ctrl Pts',(5.52581229919439,7.56769805248282,9.49776797732741));
#81078=CARTESIAN_POINT('Ctrl Pts',(5.60438058801465,7.50961332908845,9.4961016538837));
#81079=CARTESIAN_POINT('Ctrl Pts',(5.63822172271278,7.48423876800121,9.49538377525311));
#81080=CARTESIAN_POINT('Ctrl Pts',(5.7219620913717,7.42055873632359,9.49360640368073));
#81081=CARTESIAN_POINT('Ctrl Pts',(5.77164950557834,7.38197833547766,9.49255069601179));
#81082=CARTESIAN_POINT('Ctrl Pts',(6.06694834477417,7.14788579571534,9.48625836594702));
#81083=CARTESIAN_POINT('Ctrl Pts',(6.30299734301444,6.94063107224696,9.48114574855487));
#81084=CARTESIAN_POINT('Ctrl Pts',(6.64674984012617,6.60678530211221,9.4732815543103));
#81085=CARTESIAN_POINT('Ctrl Pts',(6.76223432132835,6.48853468046768,9.47056128196258));
#81086=CARTESIAN_POINT('Ctrl Pts',(6.96129923039886,6.27361163007989,9.46569917405322));
#81087=CARTESIAN_POINT('Ctrl Pts',(7.04614340965096,6.17816742966272,9.46356707552349));
#81088=CARTESIAN_POINT('Ctrl Pts',(7.18223538320132,6.01862163160117,9.46003864499625));
#81089=CARTESIAN_POINT('Ctrl Pts',(7.23463882411581,5.95552789360259,9.45865214098032));
#81090=CARTESIAN_POINT('Ctrl Pts',(7.33280058411274,5.8341333372522,9.45599976231085));
#81091=CARTESIAN_POINT('Ctrl Pts',(7.37870879379131,5.77596162658633,9.45473525371776));
#81092=CARTESIAN_POINT('Ctrl Pts',(7.50298628873414,5.61458575766365,9.45124450731841));
#81093=CARTESIAN_POINT('Ctrl Pts',(7.57991212246916,5.51029114991421,9.44900725204018));
#81094=CARTESIAN_POINT('Ctrl Pts',(7.84393413441098,5.13633973768745,9.44105517721986));
#81095=CARTESIAN_POINT('Ctrl Pts',(8.01900261473456,4.8584858071132,9.43526318669941));
#81096=CARTESIAN_POINT('Ctrl Pts',(8.25963368823789,4.42800826986699,9.42661203351528));
#81097=CARTESIAN_POINT('Ctrl Pts',(8.33631847964263,4.28189214804586,9.42373001321036));
#81098=CARTESIAN_POINT('Ctrl Pts',(8.43337251481296,4.08446310033048,9.41993869383379));
#81099=CARTESIAN_POINT('Ctrl Pts',(8.45720441038539,4.03488591799286,9.41899515228053));
#81100=CARTESIAN_POINT('Ctrl Pts',(8.49860547716727,3.94678131045373,9.4173351826119));
#81101=CARTESIAN_POINT('Ctrl Pts',(8.51635252066377,3.90833948311989,9.41661667506771));
#81102=CARTESIAN_POINT('Ctrl Pts',(8.56005614033439,3.81196196892723,9.41482904241899));
#81103=CARTESIAN_POINT('Ctrl Pts',(8.58568559739771,3.75388039605313,9.41376382152321));
#81104=CARTESIAN_POINT('Ctrl Pts',(8.68184900646131,3.52981683746638,9.40969315287613));
#81105=CARTESIAN_POINT('Ctrl Pts',(8.74817605744322,3.36207154880467,9.40672588775671));
#81106=CARTESIAN_POINT('Ctrl Pts',(8.89273712931841,2.96316108957192,9.39976399701432));
#81107=CARTESIAN_POINT('Ctrl Pts',(8.96686474473988,2.73064715455162,9.39577739382965));
#81108=CARTESIAN_POINT('Ctrl Pts',(9.06225290468573,2.38541461162855,9.38986060591404));
#81109=CARTESIAN_POINT('Ctrl Pts',(9.09065591924087,2.27477591423973,9.38796526118295));
#81110=CARTESIAN_POINT('Ctrl Pts',(9.14020187420241,2.06600241434345,9.38438203727956));
#81111=CARTESIAN_POINT('Ctrl Pts',(9.16180435576896,1.96799318074359,9.38269715138645));
#81112=CARTESIAN_POINT('Ctrl Pts',(9.19742641111772,1.79305426802685,9.37968154163352));
#81113=CARTESIAN_POINT('Ctrl Pts',(9.21206526222652,1.71626040210631,9.37835498994969));
#81114=CARTESIAN_POINT('Ctrl Pts',(9.24235958490316,1.54576758662341,9.37540272357384));
#81115=CARTESIAN_POINT('Ctrl Pts',(9.25755458509737,1.45199558362127,9.37377418846392));
#81116=CARTESIAN_POINT('Ctrl Pts',(9.29560300523196,1.19223357970133,9.36924960925944));
#81117=CARTESIAN_POINT('Ctrl Pts',(9.31543417348264,1.02583723526141,9.36633589613563));
#81118=CARTESIAN_POINT('Ctrl Pts',(9.35639340952671,0.580921644502694,9.35852038266875));
#81119=CARTESIAN_POINT('Ctrl Pts',(9.36954963341063,0.301839177342059,9.35358915406841));
#81120=CARTESIAN_POINT('Ctrl Pts',(9.37044699854996,-0.0704308501302653,
9.34707510341973));
#81121=CARTESIAN_POINT('Ctrl Pts',(9.36928612722907,-0.163447161744229,
9.34545327309791));
#81122=CARTESIAN_POINT('Ctrl Pts',(9.36480789685254,-0.327025070621559,
9.34261875581561));
#81123=CARTESIAN_POINT('Ctrl Pts',(9.36207724474583,-0.397595322602507,
9.34140168813984));
#81124=CARTESIAN_POINT('Ctrl Pts',(9.35639398578417,-0.511211793718479,
9.33945495319131));
#81125=CARTESIAN_POINT('Ctrl Pts',(9.35394138236341,-0.554280212197695,
9.33872000764582));
#81126=CARTESIAN_POINT('Ctrl Pts',(9.34792994862151,-0.648389055888332,
9.33712141256178));
#81127=CARTESIAN_POINT('Ctrl Pts',(9.34425031656819,-0.699420280653494,
9.33625905632767));
#81128=CARTESIAN_POINT('Ctrl Pts',(9.33145772012152,-0.858644430268895,
9.33357914529558));
#81129=CARTESIAN_POINT('Ctrl Pts',(9.3208821198359,-0.9667109456824,9.3317757186527));
#81130=CARTESIAN_POINT('Ctrl Pts',(9.30401212629843,-1.11284684644981,9.32934543124297));
#81131=CARTESIAN_POINT('Ctrl Pts',(9.29935729966201,-1.15109667967718,9.32871012117066));
#81132=CARTESIAN_POINT('Ctrl Pts',(9.26443491950193,-1.42401380191301,9.32418010830899));
#81133=CARTESIAN_POINT('Ctrl Pts',(9.22552433555031,-1.65748924902257,9.32031827007886));
#81134=CARTESIAN_POINT('Ctrl Pts',(9.13595634008771,-2.09260510684001,9.31301364505869));
#81135=CARTESIAN_POINT('Ctrl Pts',(9.08734657670621,-2.29452090664058,9.30957984551121));
#81136=CARTESIAN_POINT('Ctrl Pts',(9.00755067226226,-2.58342753083447,9.30456132642562));
#81137=CARTESIAN_POINT('Ctrl Pts',(8.98172415534935,-2.67183421391164,9.30301139706521));
#81138=CARTESIAN_POINT('Ctrl Pts',(8.93127584265924,-2.83551887206895,9.30011268701998));
#81139=CARTESIAN_POINT('Ctrl Pts',(8.90699476095773,-2.91089328999987,9.29876629690617));
#81140=CARTESIAN_POINT('Ctrl Pts',(8.84890288132995,-3.08368857217402,9.29565205285586));
#81141=CARTESIAN_POINT('Ctrl Pts',(8.81443349841996,-3.18087714990394,9.29387995360391));
#81142=CARTESIAN_POINT('Ctrl Pts',(8.67896695350965,-3.54370963719546,9.28718743234917));
#81143=CARTESIAN_POINT('Ctrl Pts',(8.5675069263532,-3.80528176575947,9.2822017180191));
#81144=CARTESIAN_POINT('Ctrl Pts',(8.36861799256515,-4.2188071011161,9.27413412590122));
#81145=CARTESIAN_POINT('Ctrl Pts',(8.28851544384235,-4.37408416826252,9.27106175304408));
#81146=CARTESIAN_POINT('Ctrl Pts',(8.16777757532142,-4.59289155616682,9.26670327874903));
#81147=CARTESIAN_POINT('Ctrl Pts',(8.13064405627935,-4.6583119935548,9.26539643963388));
#81148=CARTESIAN_POINT('Ctrl Pts',(8.06205954814954,-4.77582268297343,9.26304652122073));
#81149=CARTESIAN_POINT('Ctrl Pts',(8.03088121694346,-4.82806724897704,9.26200084765485));
#81150=CARTESIAN_POINT('Ctrl Pts',(7.97722788383948,-4.91601461416808,9.26024134918533));
#81151=CARTESIAN_POINT('Ctrl Pts',(7.95501663813909,-4.95187587661961,9.25952424108078));
#81152=CARTESIAN_POINT('Ctrl Pts',(7.902769861629,-5.03497236498125,9.25786344988203));
#81153=CARTESIAN_POINT('Ctrl Pts',(7.87255178934908,-5.08209076517123,9.25692211816725));
#81154=CARTESIAN_POINT('Ctrl Pts',(7.74318500037833,-5.27988680221872,9.25296645397048));
#81155=CARTESIAN_POINT('Ctrl Pts',(7.64011840087408,-5.42795631934355,9.24999445273794));
#81156=CARTESIAN_POINT('Ctrl Pts',(7.51077716053704,-5.60278394269041,9.24642399614157));
#81157=CARTESIAN_POINT('Ctrl Pts',(7.4885350553743,-5.63247762437499,9.24581540170336));
#81158=CARTESIAN_POINT('Ctrl Pts',(7.32742010786547,-5.8449281566664,9.24144326797074));
#81159=CARTESIAN_POINT('Ctrl Pts',(7.18204980015554,-6.0226598065445,9.23768824680844));
#81160=CARTESIAN_POINT('Ctrl Pts',(6.95673023654192,-6.27836546937115,9.23205466590245));
#81161=CARTESIAN_POINT('Ctrl Pts',(6.88167852858946,-6.36054000133931,9.2302068695419));
#81162=CARTESIAN_POINT('Ctrl Pts',(6.73738896231142,-6.51297938112824,9.22669991103106));
#81163=CARTESIAN_POINT('Ctrl Pts',(6.66847044716011,-6.58352582454055,9.22504345183941));
#81164=CARTESIAN_POINT('Ctrl Pts',(6.54245442012927,-6.70850917518572,9.22204441711765));
#81165=CARTESIAN_POINT('Ctrl Pts',(6.4857586256957,-6.76333794872587,9.22070555330623));
#81166=CARTESIAN_POINT('Ctrl Pts',(6.35788910450053,-6.88391004436583,9.21770787794153));
#81167=CARTESIAN_POINT('Ctrl Pts',(6.28637424503067,-6.94927839092255,9.21604599682086));
#81168=CARTESIAN_POINT('Ctrl Pts',(6.02948753800526,-7.17687542740149,9.21012753209563));
#81169=CARTESIAN_POINT('Ctrl Pts',(5.8387475392438,-7.33289078417603,9.20582242655031));
#81170=CARTESIAN_POINT('Ctrl Pts',(5.50115396283354,-7.58749283641007,9.19839581687746));
#81171=CARTESIAN_POINT('Ctrl Pts',(5.35724960377537,-7.68977367399845,9.19528693947165));
#81172=CARTESIAN_POINT('Ctrl Pts',(5.08796162469178,-7.8699417889886,9.18961019070575));
#81173=CARTESIAN_POINT('Ctrl Pts',(4.96346131076589,-7.94904958337707,9.18703839956719));
#81174=CARTESIAN_POINT('Ctrl Pts',(4.79123360275638,-8.05285907872073,9.18357484853085));
#81175=CARTESIAN_POINT('Ctrl Pts',(4.74508494056717,-8.08013785168453,9.18265581543761));
#81176=CARTESIAN_POINT('Ctrl Pts',(4.66189838538814,-8.12835151058474,9.18101701259624));
#81177=CARTESIAN_POINT('Ctrl Pts',(4.62494733022896,-8.14943292677324,9.18029546081728));
#81178=CARTESIAN_POINT('Ctrl Pts',(4.54035388409291,-8.19693475373523,9.17865734960211));
#81179=CARTESIAN_POINT('Ctrl Pts',(4.49262208188251,-8.22319278604103,9.17774276906602));
#81180=CARTESIAN_POINT('Ctrl Pts',(4.19453131861664,-8.38380715774307,9.17208350968724));
#81181=CARTESIAN_POINT('Ctrl Pts',(3.93839708150444,-8.50713495504286,9.16744448817043));
#81182=CARTESIAN_POINT('Ctrl Pts',(3.44263854538389,-8.71864544135651,9.15860726727459));
#81183=CARTESIAN_POINT('Ctrl Pts',(3.20423974175878,-8.8090513500388,9.15441704631916));
#81184=CARTESIAN_POINT('Ctrl Pts',(2.86494923647387,-8.92211935581875,9.14844879939828));
#81185=CARTESIAN_POINT('Ctrl Pts',(2.76691725996314,-8.95300601669009,9.14672431696656));
#81186=CARTESIAN_POINT('Ctrl Pts',(2.59263891609513,-9.00477952789019,9.14365476592094));
#81187=CARTESIAN_POINT('Ctrl Pts',(2.51659902380786,-9.02632595327815,9.14231423436405));
#81188=CARTESIAN_POINT('Ctrl Pts',(2.34999857392712,-9.07126444299362,9.13937339891728));
#81189=CARTESIAN_POINT('Ctrl Pts',(2.25934193176152,-9.0942677480084,9.13777068866701));
#81190=CARTESIAN_POINT('Ctrl Pts',(1.77310745676169,-9.20992593034401,9.12916118171145));
#81191=CARTESIAN_POINT('Ctrl Pts',(1.37216367968342,-9.2781360682612,9.12199309533682));
#81192=CARTESIAN_POINT('Ctrl Pts',(0.799001641982031,-9.33766953932976,
9.11188168263922));
#81193=CARTESIAN_POINT('Ctrl Pts',(0.629490727653586,-9.35062659657888,
9.10891117063052));
#81194=CARTESIAN_POINT('Ctrl Pts',(0.404443021924749,-9.36168114953993,
9.10502756096534));
#81195=CARTESIAN_POINT('Ctrl Pts',(0.349141860416359,-9.36390666783527,
9.10407809876825));
#81196=CARTESIAN_POINT('Ctrl Pts',(0.251541049242236,-9.36696865500938,
9.10241281362844));
#81197=CARTESIAN_POINT('Ctrl Pts',(0.209249627321041,-9.36800882151119,
9.10169483981409));
#81198=CARTESIAN_POINT('Ctrl Pts',(0.114419571983502,-9.36969870369127,
9.10009248913521));
#81199=CARTESIAN_POINT('Ctrl Pts',(0.0618797252813041,-9.3701929836948,
9.09920976079177));
#81200=CARTESIAN_POINT('Ctrl Pts',(-0.294255055835618,-9.37054790958427,
9.09325286770774));
#81201=CARTESIAN_POINT('Ctrl Pts',(-0.597685142130283,-9.35609577851258,
9.08830240290459));
#81202=CARTESIAN_POINT('Ctrl Pts',(-1.07531902166894,-9.3100128939096,9.08043226456062));
#81203=CARTESIAN_POINT('Ctrl Pts',(-1.25024713984585,-9.28813937303063,
9.07753466725273));
#81204=CARTESIAN_POINT('Ctrl Pts',(-1.555726937633,-9.24115463964584,9.07240955003862));
#81205=CARTESIAN_POINT('Ctrl Pts',(-1.68655571299866,-9.21817525708584,
9.07019365337112));
#81206=CARTESIAN_POINT('Ctrl Pts',(-1.89804940717955,-9.17637423860968,
9.06656815380644));
#81207=CARTESIAN_POINT('Ctrl Pts',(-1.97903099948778,-9.1592506234975,9.06516958693894));
#81208=CARTESIAN_POINT('Ctrl Pts',(-2.14099090091565,-9.12275583160073,
9.06235018572201));
#81209=CARTESIAN_POINT('Ctrl Pts',(-2.22195920245591,-9.10337372977637,
9.06092939412982));
#81210=CARTESIAN_POINT('Ctrl Pts',(-2.43456898125982,-9.04947388979151,
9.05716807084339));
#81211=CARTESIAN_POINT('Ctrl Pts',(-2.56573514857004,-9.01316297400307,
9.05481631093867));
#81212=CARTESIAN_POINT('Ctrl Pts',(-3.00824289621076,-8.88022026009241,
9.04678124313245));
#81213=CARTESIAN_POINT('Ctrl Pts',(-3.31531523609645,-8.77020643205332,
9.04102587809431));
#81214=CARTESIAN_POINT('Ctrl Pts',(-3.76064999033695,-8.58391940228398,
9.0325623314531));
#81215=CARTESIAN_POINT('Ctrl Pts',(-3.90373212527148,-8.51980260235047,
9.02982611835058));
#81216=CARTESIAN_POINT('Ctrl Pts',(-4.09420059841487,-8.42864550009434,
9.02618800970519));
#81217=CARTESIAN_POINT('Ctrl Pts',(-4.14305743641789,-8.40473786640785,
9.02525523816701));
#81218=CARTESIAN_POINT('Ctrl Pts',(-4.2296407228366,-8.36143072241235,9.02360474481637));
#81219=CARTESIAN_POINT('Ctrl Pts',(-4.26744865942165,-8.34219793043387,
9.02288507267542));
#81220=CARTESIAN_POINT('Ctrl Pts',(-4.35269498263181,-8.29810218482182,
9.0212641201556));
#81221=CARTESIAN_POINT('Ctrl Pts',(-4.40005339633608,-8.27308791246818,
9.02036466200209));
#81222=CARTESIAN_POINT('Ctrl Pts',(-4.71992563628664,-8.10061079552707,
9.01428864104597));
#81223=CARTESIAN_POINT('Ctrl Pts',(-4.98519543132521,-7.94011469892821,
9.00923917339297));
#81224=CARTESIAN_POINT('Ctrl Pts',(-5.38420151980779,-7.67081357029556,
9.00134200093529));
#81225=CARTESIAN_POINT('Ctrl Pts',(-5.52371483394541,-7.57096962837416,
8.99852062308063));
#81226=CARTESIAN_POINT('Ctrl Pts',(-5.70955103074617,-7.43010193071963,
8.99465231770901));
#81227=CARTESIAN_POINT('Ctrl Pts',(-5.75832447725486,-7.39236679793993,
8.993626458969));
#81228=CARTESIAN_POINT('Ctrl Pts',(-5.88681654913273,-7.29091150882686,
8.99089378213007));
#81229=CARTESIAN_POINT('Ctrl Pts',(-5.96587261084626,-7.22636586649598,
8.98918113876672));
#81230=CARTESIAN_POINT('Ctrl Pts',(-6.10421984257092,-7.10959382680616,
8.98612410231501));
#81231=CARTESIAN_POINT('Ctrl Pts',(-6.16393453174081,-7.05788462099976,
8.98478410253716));
#81232=CARTESIAN_POINT('Ctrl Pts',(-6.29329596295239,-6.9429716117047,8.98183478794692));
#81233=CARTESIAN_POINT('Ctrl Pts',(-6.36265939710194,-6.8794617681,8.98022296319369));
#81234=CARTESIAN_POINT('Ctrl Pts',(-6.71952225635856,-6.54269991373574,
8.97176921967462));
#81235=CARTESIAN_POINT('Ctrl Pts',(-6.99041353231866,-6.25244086853392,
8.96477520895331));
#81236=CARTESIAN_POINT('Ctrl Pts',(-7.35438901821969,-5.80911913994624,
8.95470662886602));
#81237=CARTESIAN_POINT('Ctrl Pts',(-7.46278760415433,-5.66918905010321,
8.95161188861302));
#81238=CARTESIAN_POINT('Ctrl Pts',(-7.60005385784144,-5.48122955615698,
8.94759956921163));
#81239=CARTESIAN_POINT('Ctrl Pts',(-7.63254631137156,-5.43589301895453,
8.94664254552966));
#81240=CARTESIAN_POINT('Ctrl Pts',(-7.68894429827777,-5.35569853915122,
8.94497036964128));
#81241=CARTESIAN_POINT('Ctrl Pts',(-7.71302224522151,-5.32096411497662,
8.9442529757433));
#81242=CARTESIAN_POINT('Ctrl Pts',(-7.76626302693181,-5.24303913760968,
8.94265833093854));
#81243=CARTESIAN_POINT('Ctrl Pts',(-7.79530213182425,-5.19976590731973,
8.94178265397177));
#81244=CARTESIAN_POINT('Ctrl Pts',(-7.99202140965166,-4.90126861409037,
8.93580201065583));
#81245=CARTESIAN_POINT('Ctrl Pts',(-8.14749938200692,-4.63822117625748,
8.930822900853));
#81246=CARTESIAN_POINT('Ctrl Pts',(-8.40268299762345,-4.15392395794922,
8.92184448933034));
#81247=CARTESIAN_POINT('Ctrl Pts',(-8.50717124373083,-3.93550540418218,
8.91786084378229));
#81248=CARTESIAN_POINT('Ctrl Pts',(-8.64340597654639,-3.61987161047319,
8.91212218162982));
#81249=CARTESIAN_POINT('Ctrl Pts',(-8.68220217287086,-3.52580525756368,
8.9104145444596));
#81250=CARTESIAN_POINT('Ctrl Pts',(-8.74837621495052,-3.35763835336013,
8.90736277249834));
#81251=CARTESIAN_POINT('Ctrl Pts',(-8.7763635092829,-3.28378824371271,8.90602297027732));
#81252=CARTESIAN_POINT('Ctrl Pts',(-8.83570347310056,-3.12102797649012,
8.9030699097792));
#81253=CARTESIAN_POINT('Ctrl Pts',(-8.86665467245573,-3.03198059981565,
8.90145409643289));
#81254=CARTESIAN_POINT('Ctrl Pts',(-9.01940183949125,-2.57016698236896,
8.89307300459722));
#81255=CARTESIAN_POINT('Ctrl Pts',(-9.11905242678053,-2.19049023604211,
8.88615978438924));
#81256=CARTESIAN_POINT('Ctrl Pts',(-9.22936587530118,-1.62877216532722,
8.87610977621629));
#81257=CARTESIAN_POINT('Ctrl Pts',(-9.25899705466085,-1.45088492859274,
8.87295584223503));
#81258=CARTESIAN_POINT('Ctrl Pts',(-9.29107632182573,-1.21680646084682,
8.86888253320462));
#81259=CARTESIAN_POINT('Ctrl Pts',(-9.29817817201224,-1.1612923327927,8.86792220440896));
#81260=CARTESIAN_POINT('Ctrl Pts',(-9.30976764725163,-1.0637651521011,8.86624698229964));
#81261=CARTESIAN_POINT('Ctrl Pts',(-9.31446921792621,-1.02177939750383,
8.865529807736));
#81262=CARTESIAN_POINT('Ctrl Pts',(-9.32538519108151,-0.917953563784677,
8.86376572573016));
#81263=CARTESIAN_POINT('Ctrl Pts',(-9.33126858183865,-0.856080829411509,
8.86272244821995));
#81264=CARTESIAN_POINT('Ctrl Pts',(-9.35899521502701,-0.530110439331893,
8.85725832551379));
#81265=CARTESIAN_POINT('Ctrl Pts',(-9.37024340926094,-0.265231948612504,
8.85292626627514));
#81266=CARTESIAN_POINT('Ctrl Pts',(-9.37025268437787,0.107863849306275,
8.84681041898646));
#81267=CARTESIAN_POINT('Ctrl Pts',(-9.36838483711979,0.215952541891298,
8.84503746952965));
#81268=CARTESIAN_POINT('Ctrl Pts',(-9.35805287421797,0.514593863841188,
8.84011970950323));
#81269=CARTESIAN_POINT('Ctrl Pts',(-9.34564047711994,0.70495687852041,8.83696255375387));
#81270=CARTESIAN_POINT('Ctrl Pts',(-9.31858177038158,0.987015371593162,
8.83221905460276));
#81271=CARTESIAN_POINT('Ctrl Pts',(-9.30836922471958,1.07908659499721,8.83066041181346));
#81272=CARTESIAN_POINT('Ctrl Pts',(-9.28699981374936,1.24874373085893,8.82776693649957));
#81273=CARTESIAN_POINT('Ctrl Pts',(-9.27623135574785,1.32637032822497,8.82643472508075));
#81274=CARTESIAN_POINT('Ctrl Pts',(-9.24896706100079,1.50629648236639,8.82332666186428));
#81275=CARTESIAN_POINT('Ctrl Pts',(-9.23174559910193,1.60847564732476,8.82154632488248));
#81276=CARTESIAN_POINT('Ctrl Pts',(-9.16591337043864,1.96308263203714,8.815314961699));
#81277=CARTESIAN_POINT('Ctrl Pts',(-9.10861374643787,2.21377869414352,8.81081285321358));
#81278=CARTESIAN_POINT('Ctrl Pts',(-8.96757869368305,2.73173674989091,8.80137773342682));
#81279=CARTESIAN_POINT('Ctrl Pts',(-8.88202516743433,2.99824659482927,8.79644607764688));
#81280=CARTESIAN_POINT('Ctrl Pts',(-8.76571321950822,3.31161995711214,8.79067409615914));
#81281=CARTESIAN_POINT('Ctrl Pts',(-8.7463047242291,3.36254496998548,8.78973715264741));
#81282=CARTESIAN_POINT('Ctrl Pts',(-8.71095547586105,3.45291902218372,8.78807800945795));
#81283=CARTESIAN_POINT('Ctrl Pts',(-8.69518822609136,3.49243422396195,8.78735388533094));
#81284=CARTESIAN_POINT('Ctrl Pts',(-8.65895304607231,3.58147862292254,8.78572560255436));
#81285=CARTESIAN_POINT('Ctrl Pts',(-8.63832826958899,3.63094226129281,8.78482328010475));
#81286=CARTESIAN_POINT('Ctrl Pts',(-8.55942728271194,3.81568957318128,8.78145678281294));
#81287=CARTESIAN_POINT('Ctrl Pts',(-8.49838794363135,3.94977023643038,8.77902071717173));
#81288=CARTESIAN_POINT('Ctrl Pts',(-8.3490870545859,4.25822824305022,8.77338125894572));
#81289=CARTESIAN_POINT('Ctrl Pts',(-8.25848078896065,4.43139454157599,8.77018785547254));
#81290=CARTESIAN_POINT('Ctrl Pts',(-8.14459213335217,4.63341535357859,8.76638071203237));
#81291=CARTESIAN_POINT('Ctrl Pts',(-8.12647125538625,4.66512419894607,8.76578074295402));
#81292=CARTESIAN_POINT('Ctrl Pts',(-8.00653210231113,4.87218044198863,8.76184577427303));
#81293=CARTESIAN_POINT('Ctrl Pts',(-7.89923074998114,5.0442890245467,8.75849231976839));
#81294=CARTESIAN_POINT('Ctrl Pts',(-7.73467287586928,5.29009230476958,8.75354114846756));
#81295=CARTESIAN_POINT('Ctrl Pts',(-7.68176637577617,5.36662895915337,8.75197586510107));
#81296=CARTESIAN_POINT('Ctrl Pts',(-7.58180019025184,5.50673624388029,8.74906380736425));
#81297=CARTESIAN_POINT('Ctrl Pts',(-7.53505846102861,5.57052350677772,8.74771961945226));
#81298=CARTESIAN_POINT('Ctrl Pts',(-7.4252933693707,5.71640740366725,8.74460161172465));
#81299=CARTESIAN_POINT('Ctrl Pts',(-7.36170611254615,5.79806676962057,8.74282344627031));
#81300=CARTESIAN_POINT('Ctrl Pts',(-7.25726145635692,5.92770688216262,8.73994721918224));
#81301=CARTESIAN_POINT('Ctrl Pts',(-7.21724995715422,5.97635806893226,8.73885542658812));
#81302=CARTESIAN_POINT('Ctrl Pts',(-7.06266816843614,6.16050218218445,8.73467621288963));
#81303=CARTESIAN_POINT('Ctrl Pts',(-6.9447484415149,6.29313416713875,8.73156725799665));
#81304=CARTESIAN_POINT('Ctrl Pts',(-6.61916881284147,6.63903214181431,8.72322126585896));
#81305=CARTESIAN_POINT('Ctrl Pts',(-6.40499584022498,6.84588724794792,8.71796969001007));
#81306=CARTESIAN_POINT('Ctrl Pts',(-6.14067002705748,7.07790121621837,8.71189733168689));
#81307=CARTESIAN_POINT('Ctrl Pts',(-6.09968780999389,7.11324979494781,8.71096699855222));
#81308=CARTESIAN_POINT('Ctrl Pts',(-6.02598635861062,7.17571452818762,8.70931538650168));
#81309=CARTESIAN_POINT('Ctrl Pts',(-5.99338460022587,7.20296686352822,8.70859224656729));
#81310=CARTESIAN_POINT('Ctrl Pts',(-5.91900693847331,7.2642857543988,8.70695972052593));
#81311=CARTESIAN_POINT('Ctrl Pts',(-5.87712026633571,7.29821540186579,8.70605223885133));
#81312=CARTESIAN_POINT('Ctrl Pts',(-5.71690315241531,7.42572298086308,8.70262132886636));
#81313=CARTESIAN_POINT('Ctrl Pts',(-5.59661140932683,7.51680014530366,8.70012742959838));
#81314=CARTESIAN_POINT('Ctrl Pts',(-5.12897549253816,7.85341320761312,8.69064833319487));
#81315=CARTESIAN_POINT('Ctrl Pts',(-4.76726099745434,8.07810075660881,8.6837346824621));
#81316=CARTESIAN_POINT('Ctrl Pts',(-4.30789064341698,8.32181646966828,8.67503548251408));
#81317=CARTESIAN_POINT('Ctrl Pts',(-4.22357670241305,8.36492384509776,8.67344322681352));
#81318=CARTESIAN_POINT('Ctrl Pts',(-4.06779610322451,8.44161432035405,8.67050665793764));
#81319=CARTESIAN_POINT('Ctrl Pts',(-3.99653042713863,8.47558623236571,8.66916526938074));
#81320=CARTESIAN_POINT('Ctrl Pts',(-3.83295609984953,8.55103926757147,8.66609003884345));
#81321=CARTESIAN_POINT('Ctrl Pts',(-3.74038771363289,8.59193369979667,8.66435229403882));
#81322=CARTESIAN_POINT('Ctrl Pts',(-3.54065440162147,8.67633125956585,8.66060842470857));
#81323=CARTESIAN_POINT('Ctrl Pts',(-3.43330958231042,8.71936597133163,8.65859969221885));
#81324=CARTESIAN_POINT('Ctrl Pts',(-3.09020852552795,8.84959722763654,8.65219580415127));
#81325=CARTESIAN_POINT('Ctrl Pts',(-2.85172765751044,8.92930057492297,8.64776647826332));
#81326=CARTESIAN_POINT('Ctrl Pts',(-2.43413672260732,9.05042652684473,8.64013135673377));
#81327=CARTESIAN_POINT('Ctrl Pts',(-2.25647770286536,9.09634820085321,8.63692072725445));
#81328=CARTESIAN_POINT('Ctrl Pts',(-2.02262624886551,9.14952155925395,8.6327845502938));
#81329=CARTESIAN_POINT('Ctrl Pts',(-1.96755564824971,9.16152206222707,8.63181702790354));
#81330=CARTESIAN_POINT('Ctrl Pts',(-1.87110188287424,9.18163061503288,8.63013575518547));
#81331=CARTESIAN_POINT('Ctrl Pts',(-1.82976623019635,9.18995748394981,8.62941963901196));
#81332=CARTESIAN_POINT('Ctrl Pts',(-1.72911548642306,9.20952708937885,8.62768629425005));
#81333=CARTESIAN_POINT('Ctrl Pts',(-1.6697453413667,9.22047613163792,8.62667232903793));
#81334=CARTESIAN_POINT('Ctrl Pts',(-1.57184460688778,9.23755440094811,8.62501143381089));
#81335=CARTESIAN_POINT('Ctrl Pts',(-1.53337423738643,9.24401807829263,8.62436159870206));
#81336=CARTESIAN_POINT('Ctrl Pts',(-1.43559707673912,9.25981913804211,8.62271600745567));
#81337=CARTESIAN_POINT('Ctrl Pts',(-1.37623881255984,9.26882712000772,8.62172263441406));
#81338=CARTESIAN_POINT('Ctrl Pts',(-1.08842890310867,9.30967833675424,8.61692603914));
#81339=CARTESIAN_POINT('Ctrl Pts',(-0.858940535065887,9.33364932121365,
8.61316018367611));
#81340=CARTESIAN_POINT('Ctrl Pts',(-0.563496147272652,9.35352026102381,
8.60829858381005));
#81341=CARTESIAN_POINT('Ctrl Pts',(-0.498146311825352,9.35722819136987,
8.60722256040794));
#81342=CARTESIAN_POINT('Ctrl Pts',(-0.250080797523833,9.36869728378259,
8.60313095678301));
#81343=CARTESIAN_POINT('Ctrl Pts',(-0.0671909225601672,9.37179354697312,
8.60009902462655));
#81344=CARTESIAN_POINT('Ctrl Pts',(0.205221869031554,9.36843047139318,8.59553300048761));
#81345=CARTESIAN_POINT('Ctrl Pts',(0.294751411040575,9.36604116322681,8.59402448099187));
#81346=CARTESIAN_POINT('Ctrl Pts',(0.463807694672769,9.35910307217614,8.5911589339721));
#81347=CARTESIAN_POINT('Ctrl Pts',(0.543337609215069,9.35482293263922,8.58980375019918));
#81348=CARTESIAN_POINT('Ctrl Pts',(0.732349121603673,9.34223224885276,8.58656517048775));
#81349=CARTESIAN_POINT('Ctrl Pts',(0.841758138276836,9.33301032771867,8.58467620134214));
#81350=CARTESIAN_POINT('Ctrl Pts',(1.01952946797695,9.31487480947402,8.58158415975769));
#81351=CARTESIAN_POINT('Ctrl Pts',(1.08800004555837,9.30712570747342,8.58038773265554));
#81352=CARTESIAN_POINT('Ctrl Pts',(1.36071115732413,9.27321128911757,8.57560209269231));
#81353=CARTESIAN_POINT('Ctrl Pts',(1.56415000423328,9.24107228193029,8.57198501153264));
#81354=CARTESIAN_POINT('Ctrl Pts',(1.79910806723469,9.19597231952212,8.56777863886149));
#81355=CARTESIAN_POINT('Ctrl Pts',(1.83181834033569,9.18951240856489,8.56719242032351));
#81356=CARTESIAN_POINT('Ctrl Pts',(2.06511807065275,9.14214318361481,8.56300790403777));
#81357=CARTESIAN_POINT('Ctrl Pts',(2.26435430636634,9.09484439319207,8.55941494560655));
#81358=CARTESIAN_POINT('Ctrl Pts',(2.52425635911401,9.02407302886399,8.55475701333782));
#81359=CARTESIAN_POINT('Ctrl Pts',(2.58645412892499,9.00644320828199,8.55364465287884));
#81360=CARTESIAN_POINT('Ctrl Pts',(2.68917311007708,8.97617591837421,8.55181419076773));
#81361=CARTESIAN_POINT('Ctrl Pts',(2.72979969582687,8.96390427061243,8.55109203371547));
#81362=CARTESIAN_POINT('Ctrl Pts',(2.82216184314708,8.93531925161914,8.54945479215524));
#81363=CARTESIAN_POINT('Ctrl Pts',(2.87384181467495,8.91883180912912,8.54854168608087));
#81364=CARTESIAN_POINT('Ctrl Pts',(3.07257372937519,8.85352375627285,8.54503715444029));
#81365=CARTESIAN_POINT('Ctrl Pts',(3.21854968678172,8.80150728031443,8.54247692843226));
#81366=CARTESIAN_POINT('Ctrl Pts',(3.67977565580826,8.62414626538968,8.5343500946697));
#81367=CARTESIAN_POINT('Ctrl Pts',(3.98948105651241,8.48531714292376,8.52882759647274));
#81368=CARTESIAN_POINT('Ctrl Pts',(4.2909266557441,8.33003802497472,8.52320208943219));
#81369=CARTESIAN_POINT('',(-9.37090856232268,0.000113764305748557,8.65141010809498));
#81370=CARTESIAN_POINT('Ctrl Pts',(4.29124604933307,8.33065733261531,8.32570386727427));
#81371=CARTESIAN_POINT('Ctrl Pts',(4.20718224374021,8.37401666214134,8.32731082159403));
#81372=CARTESIAN_POINT('Ctrl Pts',(2.73864022413988,9.10315303786724,8.35516338033944));
#81373=CARTESIAN_POINT('Ctrl Pts',(-0.481341462362255,9.74926409850946,
8.40926154351051));
#81374=CARTESIAN_POINT('Ctrl Pts',(-5.05241933911021,8.35182009430635,8.48799835678748));
#81375=CARTESIAN_POINT('Ctrl Pts',(-8.41195372822347,4.95165371770902,8.56673517006447));
#81376=CARTESIAN_POINT('Ctrl Pts',(-9.34062849382632,1.77796225280113,8.62120575383362));
#81377=CARTESIAN_POINT('Ctrl Pts',(-9.37098027739613,0.11662354713027,8.64943073317713));
#81378=CARTESIAN_POINT('Ctrl Pts',(-9.37090856232268,0.000113764305748557,
8.65141010809498));
#81379=CARTESIAN_POINT('Ctrl Pts',(-9.37024999923123,0.000120029827953283,
8.65179019859247));
#81380=CARTESIAN_POINT('Ctrl Pts',(-9.37025649351159,-0.506862539567674,
8.66022018103747));
#81381=CARTESIAN_POINT('Ctrl Pts',(-9.32911740577704,-1.01301141890215,
8.66838655607132));
#81382=CARTESIAN_POINT('Ctrl Pts',(-9.23415704073925,-1.59326290303693,
8.67820000093685));
#81383=CARTESIAN_POINT('Ctrl Pts',(-9.22004279010089,-1.67300742574552,
8.67955740785975));
#81384=CARTESIAN_POINT('Ctrl Pts',(-9.19091374104503,-1.82600079619343,
8.68218056154493));
#81385=CARTESIAN_POINT('Ctrl Pts',(-9.17605240004904,-1.8992726571765,8.6834452427055));
#81386=CARTESIAN_POINT('Ctrl Pts',(-9.1425183203875,-2.05501651736957,8.68615242586457));
#81387=CARTESIAN_POINT('Ctrl Pts',(-9.1236028633992,-2.13742950176123,8.68759640972734));
#81388=CARTESIAN_POINT('Ctrl Pts',(-9.06924779594286,-2.36036650616878,
8.69153441147084));
#81389=CARTESIAN_POINT('Ctrl Pts',(-9.03165952283508,-2.50034231722196,
8.69404180889817));
#81390=CARTESIAN_POINT('Ctrl Pts',(-8.89818534630605,-2.95500993066266,
8.70229312028935));
#81391=CARTESIAN_POINT('Ctrl Pts',(-8.78897519415825,-3.26553212579828,
8.70810559910809));
#81392=CARTESIAN_POINT('Ctrl Pts',(-8.62602421719554,-3.66101807210239,
8.71559638661592));
#81393=CARTESIAN_POINT('Ctrl Pts',(-8.58694185550096,-3.75176981543268,
8.71732073550425));
#81394=CARTESIAN_POINT('Ctrl Pts',(-8.52387012760105,-3.89207541651779,
8.71998739585848));
#81395=CARTESIAN_POINT('Ctrl Pts',(-8.50086699364746,-3.9420646078181,8.72093763028548));
#81396=CARTESIAN_POINT('Ctrl Pts',(-8.46489474930453,-4.01845829131022,
8.72238849431909));
#81397=CARTESIAN_POINT('Ctrl Pts',(-8.45223942401119,-4.04500913199401,
8.72289250407785));
#81398=CARTESIAN_POINT('Ctrl Pts',(-8.42210804684026,-4.10746585137936,
8.72407716398779));
#81399=CARTESIAN_POINT('Ctrl Pts',(-8.40452708144422,-4.14332043467043,
8.72475641937645));
#81400=CARTESIAN_POINT('Ctrl Pts',(-8.36243547271856,-4.22779165106396,
8.7263544926167));
#81401=CARTESIAN_POINT('Ctrl Pts',(-8.33772928665667,-4.27630911427389,
8.72727088393162));
#81402=CARTESIAN_POINT('Ctrl Pts',(-8.24302551963114,-4.45834517063397,
8.73070826573865));
#81403=CARTESIAN_POINT('Ctrl Pts',(-8.17023191687614,-4.59038364940285,
8.73320003919488));
#81404=CARTESIAN_POINT('Ctrl Pts',(-7.97092248808497,-4.93213348267305,
8.73970804781442));
#81405=CARTESIAN_POINT('Ctrl Pts',(-7.83931645284388,-5.13874145147038,
8.74370413828197));
#81406=CARTESIAN_POINT('Ctrl Pts',(-7.62300846940553,-5.45063939024056,
8.74995271346713));
#81407=CARTESIAN_POINT('Ctrl Pts',(-7.54387025056358,-5.5596537142795,8.75217942520501));
#81408=CARTESIAN_POINT('Ctrl Pts',(-7.39887450017957,-5.75058934533885,
8.75617124492425));
#81409=CARTESIAN_POINT('Ctrl Pts',(-7.33393688583391,-5.83318021079825,
8.75792975967393));
#81410=CARTESIAN_POINT('Ctrl Pts',(-7.2603462110113,-5.92360455365559,8.7598935915555));
#81411=CARTESIAN_POINT('Ctrl Pts',(-7.25305154821531,-5.93253413396541,
8.76008794645715));
#81412=CARTESIAN_POINT('Ctrl Pts',(-7.19716777405375,-6.00068573098142,
8.76157453942852));
#81413=CARTESIAN_POINT('Ctrl Pts',(-7.14787062688023,-6.05932328570263,
8.76287244827627));
#81414=CARTESIAN_POINT('Ctrl Pts',(-7.0397092725749,-6.18482112374989,8.76569250652734));
#81415=CARTESIAN_POINT('Ctrl Pts',(-6.98059944490879,-6.25145985486362,
8.76721663869678));
#81416=CARTESIAN_POINT('Ctrl Pts',(-6.80004969288245,-6.44925228181714,
8.77182222273557));
#81417=CARTESIAN_POINT('Ctrl Pts',(-6.67579884112476,-6.57778384554991,
8.7749266421142));
#81418=CARTESIAN_POINT('Ctrl Pts',(-6.50794149452138,-6.74176613693223,
8.77902915899157));
#81419=CARTESIAN_POINT('Ctrl Pts',(-6.46758536447351,-6.78049059347675,
8.78000878000278));
#81420=CARTESIAN_POINT('Ctrl Pts',(-6.25058012645332,-6.98502177091228,
8.78523884335845));
#81421=CARTESIAN_POINT('Ctrl Pts',(-6.06789709761703,-7.1442918334176,8.78951308171902));
#81422=CARTESIAN_POINT('Ctrl Pts',(-5.81092756514548,-7.35135389984565,
8.79528279649356));
#81423=CARTESIAN_POINT('Ctrl Pts',(-5.74183756484015,-7.40544291400544,
8.79681113376359));
#81424=CARTESIAN_POINT('Ctrl Pts',(-5.61801874114108,-7.49960327764675,
8.79950353717946));
#81425=CARTESIAN_POINT('Ctrl Pts',(-5.56359528717286,-7.54006574310596,
8.80067141840661));
#81426=CARTESIAN_POINT('Ctrl Pts',(-5.47413396201793,-7.60508200134966,
8.80256299492667));
#81427=CARTESIAN_POINT('Ctrl Pts',(-5.43935876060615,-7.6299928686922,8.80329139093743));
#81428=CARTESIAN_POINT('Ctrl Pts',(-5.36155757113156,-7.68492275115254,
8.80490511187983));
#81429=CARTESIAN_POINT('Ctrl Pts',(-5.31844768359039,-7.71482025281318,
8.80578884960698));
#81430=CARTESIAN_POINT('Ctrl Pts',(-5.17589242883806,-7.81192217115338,
8.80868080996282));
#81431=CARTESIAN_POINT('Ctrl Pts',(-5.07540661178859,-7.8775782003973,8.81067136628687));
#81432=CARTESIAN_POINT('Ctrl Pts',(-4.71574411320661,-8.10283753209318,
8.81767229039129));
#81433=CARTESIAN_POINT('Ctrl Pts',(-4.45008302409401,-8.25172589465102,
8.82262681961192));
#81434=CARTESIAN_POINT('Ctrl Pts',(-4.10237482544841,-8.4249141011128,8.82903181691401));
#81435=CARTESIAN_POINT('Ctrl Pts',(-4.02660029643606,-8.46139154308939,
8.83042250700612));
#81436=CARTESIAN_POINT('Ctrl Pts',(-3.83707872366889,-8.5495037431181,8.8338931352177));
#81437=CARTESIAN_POINT('Ctrl Pts',(-3.72277093542957,-8.59989324540736,
8.83597976144523));
#81438=CARTESIAN_POINT('Ctrl Pts',(-3.53216935808484,-8.67940234897603,
8.83945566758665));
#81439=CARTESIAN_POINT('Ctrl Pts',(-3.45644133667225,-8.70983689623617,
8.84083575548635));
#81440=CARTESIAN_POINT('Ctrl Pts',(-3.31083666003457,-8.76615633024836,
8.84348883802847));
#81441=CARTESIAN_POINT('Ctrl Pts',(-3.24102979006502,-8.79220461928763,
8.84476059539537));
#81442=CARTESIAN_POINT('Ctrl Pts',(-3.04614320967676,-8.86228973316891,
8.84831103785598));
#81443=CARTESIAN_POINT('Ctrl Pts',(-2.92042849819513,-8.90450812838076,
8.85060143761581));
#81444=CARTESIAN_POINT('Ctrl Pts',(-2.48150036838146,-9.04161657027524,
8.85859371404788));
#81445=CARTESIAN_POINT('Ctrl Pts',(-2.16424369987789,-9.12275847598576,
8.86437043201816));
#81446=CARTESIAN_POINT('Ctrl Pts',(-1.68553094623397,-9.21881202350778,
8.87293328401931));
#81447=CARTESIAN_POINT('Ctrl Pts',(-1.5268755165505,-9.24641341817009,8.87574477115394));
#81448=CARTESIAN_POINT('Ctrl Pts',(-1.31345513209849,-9.27789926544446,
8.87946215863326));
#81449=CARTESIAN_POINT('Ctrl Pts',(-1.25925367298145,-9.28541110394687,
8.8804006527585));
#81450=CARTESIAN_POINT('Ctrl Pts',(-1.16296617978838,-9.29789709440801,
8.88205615227625));
#81451=CARTESIAN_POINT('Ctrl Pts',(-1.12090661431731,-9.30306127451821,
8.88277517591812));
#81452=CARTESIAN_POINT('Ctrl Pts',(-1.01532586045348,-9.31529834487063,
8.88457047768975));
#81453=CARTESIAN_POINT('Ctrl Pts',(-0.951764730674192,-9.32200696104571,
8.88564276325307));
#81454=CARTESIAN_POINT('Ctrl Pts',(-0.674168104554508,-9.34843737650498,
8.89029750645207));
#81455=CARTESIAN_POINT('Ctrl Pts',(-0.459558030535231,-9.3614417157428,
8.89382407419309));
#81456=CARTESIAN_POINT('Ctrl Pts',(-0.0237327382236607,-9.37282654862851,
8.90097120743279));
#81457=CARTESIAN_POINT('Ctrl Pts',(0.197360061906829,-9.37077849600656,
8.90458961010421));
#81458=CARTESIAN_POINT('Ctrl Pts',(0.527511108743546,-9.35602991781153,
8.91005457984867));
#81459=CARTESIAN_POINT('Ctrl Pts',(0.636755304105967,-9.34923025744096,
8.91187267288838));
#81460=CARTESIAN_POINT('Ctrl Pts',(0.843070483548437,-9.33275566558614,
8.91533188743398));
#81461=CARTESIAN_POINT('Ctrl Pts',(0.940158572698511,-9.32347563692473,
8.91697048231726));
#81462=CARTESIAN_POINT('Ctrl Pts',(1.11546184711251,-9.30395341845594,8.91995165965995));
#81463=CARTESIAN_POINT('Ctrl Pts',(1.1937263356886,-9.29423594208151,8.92129074788899));
#81464=CARTESIAN_POINT('Ctrl Pts',(1.36890081031289,-9.27023675847889,8.92430720448221));
#81465=CARTESIAN_POINT('Ctrl Pts',(1.46572830498296,-9.25542108495653,8.92598784943448));
#81466=CARTESIAN_POINT('Ctrl Pts',(1.96930571665265,-9.17026748581176,8.93479795188238));
#81467=CARTESIAN_POINT('Ctrl Pts',(2.37131248951925,-9.07462639303872,8.94209108834571));
#81468=CARTESIAN_POINT('Ctrl Pts',(2.91222676684544,-8.90752718030262,8.95201464584753));
#81469=CARTESIAN_POINT('Ctrl Pts',(3.05762405374741,-8.85867036180168,8.95469053969041));
#81470=CARTESIAN_POINT('Ctrl Pts',(3.25261505000611,-8.78777610492714,8.95826483745553));
#81471=CARTESIAN_POINT('Ctrl Pts',(3.30331221492835,-8.76884496170915,8.9591927718682));
#81472=CARTESIAN_POINT('Ctrl Pts',(3.39348834589402,-8.7342787132902,8.96083909884673));
#81473=CARTESIAN_POINT('Ctrl Pts',(3.43303024272975,-8.71881248499707,8.96155938269754));
#81474=CARTESIAN_POINT('Ctrl Pts',(3.52250252080767,-8.68311368722409,8.96318618392866));
#81475=CARTESIAN_POINT('Ctrl Pts',(3.57236626219022,-8.66271820041673,8.96409082525554));
#81476=CARTESIAN_POINT('Ctrl Pts',(3.9065566415305,-8.52264997470714,8.97014846811936));
#81477=CARTESIAN_POINT('Ctrl Pts',(4.18500092408065,-8.38942884047758,8.97517599875433));
#81478=CARTESIAN_POINT('Ctrl Pts',(4.60754088934357,-8.16098557584915,8.98305592539259));
#81479=CARTESIAN_POINT('Ctrl Pts',(4.75643757903536,-8.07511114579943,8.98588255202885));
#81480=CARTESIAN_POINT('Ctrl Pts',(4.95550129770197,-7.95288649967249,8.98975738093278));
#81481=CARTESIAN_POINT('Ctrl Pts',(5.00779391868184,-7.92006293177221,8.99078444265306));
#81482=CARTESIAN_POINT('Ctrl Pts',(5.1457210626929,-7.83157525036053,8.99351963598093));
#81483=CARTESIAN_POINT('Ctrl Pts',(5.23077626667062,-7.77502384161036,8.99523359707421));
#81484=CARTESIAN_POINT('Ctrl Pts',(5.37994666454844,-7.67228772205651,8.99829202600943));
#81485=CARTESIAN_POINT('Ctrl Pts',(5.44443420080633,-7.62666120939076,8.99963208458573));
#81486=CARTESIAN_POINT('Ctrl Pts',(5.58436646907857,-7.52497635037023,9.00258044368349));
#81487=CARTESIAN_POINT('Ctrl Pts',(5.65956027510835,-7.46858724064621,9.00419124247521));
#81488=CARTESIAN_POINT('Ctrl Pts',(6.06783623525312,-7.15270727278511,9.01308473621582));
#81489=CARTESIAN_POINT('Ctrl Pts',(6.38393357032377,-6.87206271680478,9.02054351403957));
#81490=CARTESIAN_POINT('Ctrl Pts',(6.78887792386997,-6.46040376722805,9.03066664266109));
#81491=CARTESIAN_POINT('Ctrl Pts',(6.89496706837064,-6.34705519562832,9.03337556447927));
#81492=CARTESIAN_POINT('Ctrl Pts',(7.03427944987019,-6.19059308379712,9.03698483476996));
#81493=CARTESIAN_POINT('Ctrl Pts',(7.070014591424,-6.14974989760854,9.03791544704441));
#81494=CARTESIAN_POINT('Ctrl Pts',(7.13305754462955,-6.07641966428299,9.0395640752394));
#81495=CARTESIAN_POINT('Ctrl Pts',(7.16050315276846,-6.04405331477298,9.04028401514766));
#81496=CARTESIAN_POINT('Ctrl Pts',(7.2221776112587,-5.97031146692123,9.04190755788627));
#81497=CARTESIAN_POINT('Ctrl Pts',(7.25627255293997,-5.9288259474065,9.04280931461069));
#81498=CARTESIAN_POINT('Ctrl Pts',(7.4842753167746,-5.6464871995492,9.04887656295522));
#81499=CARTESIAN_POINT('Ctrl Pts',(7.66651586119667,-5.39645540114406,9.05391571170361));
#81500=CARTESIAN_POINT('Ctrl Pts',(7.93020307887804,-4.99429096450534,9.06180493938049));
#81501=CARTESIAN_POINT('Ctrl Pts',(8.02038047081523,-4.84815016867082,9.06462896093072));
#81502=CARTESIAN_POINT('Ctrl Pts',(8.13743829024166,-4.64623399533749,9.06850055257106));
#81503=CARTESIAN_POINT('Ctrl Pts',(8.16785693122783,-4.59254890066005,9.06952701774821));
#81504=CARTESIAN_POINT('Ctrl Pts',(8.24719269307496,-4.44924945286953,9.07226096398601));
#81505=CARTESIAN_POINT('Ctrl Pts',(8.29517917683794,-4.35912954238198,9.07397427244909));
#81506=CARTESIAN_POINT('Ctrl Pts',(8.37766459330117,-4.19792336978694,9.07703201357378));
#81507=CARTESIAN_POINT('Ctrl Pts',(8.41275514733286,-4.12715100932985,9.07837204489025));
#81508=CARTESIAN_POINT('Ctrl Pts',(8.4876402074263,-3.97119467049436,9.08132088348316));
#81509=CARTESIAN_POINT('Ctrl Pts',(8.52705598745204,-3.88583833073623,9.08293219483968));
#81510=CARTESIAN_POINT('Ctrl Pts',(8.64790506360248,-3.61343821167718,9.08806641989808));
#81511=CARTESIAN_POINT('Ctrl Pts',(8.72451814475009,-3.42432188459326,9.09162026154793));
#81512=CARTESIAN_POINT('Ctrl Pts',(8.88220447016806,-2.99534058677072,9.0996306532592));
#81513=CARTESIAN_POINT('Ctrl Pts',(8.95985390916496,-2.75438546126452,9.10409650664386));
#81514=CARTESIAN_POINT('Ctrl Pts',(9.05160193300469,-2.42447433270116,9.11008498225815));
#81515=CARTESIAN_POINT('Ctrl Pts',(9.07431567654206,-2.33802660233176,9.11164231616266));
#81516=CARTESIAN_POINT('Ctrl Pts',(9.11229333738226,-2.18458554615929,9.11437894841737));
#81517=CARTESIAN_POINT('Ctrl Pts',(9.12806371592651,-2.11772441690329,9.11556223420342));
#81518=CARTESIAN_POINT('Ctrl Pts',(9.15248277653463,-2.00885120021582,9.117470999953));
#81519=CARTESIAN_POINT('Ctrl Pts',(9.1615807070791,-1.96694257393415,9.1182013607875));
#81520=CARTESIAN_POINT('Ctrl Pts',(9.18107941320792,-1.87405255775308,9.1198098440302));
#81521=CARTESIAN_POINT('Ctrl Pts',(9.19134388215054,-1.82304411277993,9.12068647592737));
#81522=CARTESIAN_POINT('Ctrl Pts',(9.22481840108056,-1.64922166023898,9.12365502975451));
#81523=CARTESIAN_POINT('Ctrl Pts',(9.24599590988204,-1.5260296210376,9.1257272832381));
#81524=CARTESIAN_POINT('Ctrl Pts',(9.30053058112563,-1.16576916000017,9.13173605406027));
#81525=CARTESIAN_POINT('Ctrl Pts',(9.32727567616135,-0.927801470194707,
9.13564266026207));
#81526=CARTESIAN_POINT('Ctrl Pts',(9.3611353018873,-0.468612158267803,9.14320709225622));
#81527=CARTESIAN_POINT('Ctrl Pts',(9.36958493038416,-0.247647516424963,
9.14685849954795));
#81528=CARTESIAN_POINT('Ctrl Pts',(9.37047681472042,0.0666270813668387,
9.15211856129269));
#81529=CARTESIAN_POINT('Ctrl Pts',(9.36935027356958,0.159844617067774,9.15368680849294));
#81530=CARTESIAN_POINT('Ctrl Pts',(9.36469816193931,0.332059817509742,9.15660150176988));
#81531=CARTESIAN_POINT('Ctrl Pts',(9.3615631865161,0.411059676493539,9.15794532393824));
#81532=CARTESIAN_POINT('Ctrl Pts',(9.35212443510981,0.591305782787501,9.16102777307061));
#81533=CARTESIAN_POINT('Ctrl Pts',(9.34517555676523,0.692508283373146,9.16277032763103));
#81534=CARTESIAN_POINT('Ctrl Pts',(9.31082330089939,1.09666872352164,9.16977631634854));
#81535=CARTESIAN_POINT('Ctrl Pts',(9.27031824432144,1.39832438656474,9.1751175447742));
#81536=CARTESIAN_POINT('Ctrl Pts',(9.17326469454376,1.92520712561603,9.18453673277341));
#81537=CARTESIAN_POINT('Ctrl Pts',(9.12288771495009,2.15130838613727,9.18860673414977));
#81538=CARTESIAN_POINT('Ctrl Pts',(9.04844451971082,2.4353836196773,9.19368081484227));
#81539=CARTESIAN_POINT('Ctrl Pts',(9.03210538794984,2.49529835645666,9.19474859042465));
#81540=CARTESIAN_POINT('Ctrl Pts',(9.00473109297531,2.59188524460918,9.19646367090862));
#81541=CARTESIAN_POINT('Ctrl Pts',(8.99406463776188,2.6286598264887,9.19711512974104));
#81542=CARTESIAN_POINT('Ctrl Pts',(8.96802301510867,2.71642871540583,9.19866594246824));
#81543=CARTESIAN_POINT('Ctrl Pts',(8.95243791102571,2.76735925239995,9.19956283808722));
#81544=CARTESIAN_POINT('Ctrl Pts',(8.8952639406108,2.9486589758543,9.20274900353141));
#81545=CARTESIAN_POINT('Ctrl Pts',(8.85125451149005,3.07824691894899,9.20501443844159));
#81546=CARTESIAN_POINT('Ctrl Pts',(8.72323401710809,3.42973060140032,9.21117552840955));
#81547=CARTESIAN_POINT('Ctrl Pts',(8.63360938319676,3.6494729682151,9.21504734074808));
#81548=CARTESIAN_POINT('Ctrl Pts',(8.47548134842539,3.99864210870136,9.22134864994204));
#81549=CARTESIAN_POINT('Ctrl Pts',(8.41211698584192,4.13027971127311,9.2237592546705));
#81550=CARTESIAN_POINT('Ctrl Pts',(8.29200584046233,4.36556654079858,9.22815188300912));
#81551=CARTESIAN_POINT('Ctrl Pts',(8.23632670163978,4.46972643959692,9.23012708931915));
#81552=CARTESIAN_POINT('Ctrl Pts',(8.13933018087235,4.64320960663476,9.2334750543598));
#81553=CARTESIAN_POINT('Ctrl Pts',(8.09905921990877,4.71310205292105,9.23484012451003));
#81554=CARTESIAN_POINT('Ctrl Pts',(8.01375454898479,4.85683036681564,9.23768249641162));
#81555=CARTESIAN_POINT('Ctrl Pts',(7.96859089034378,4.9305803270714,9.23916066369751));
#81556=CARTESIAN_POINT('Ctrl Pts',(7.83777723630174,5.13769924641422,9.24336877141393));
#81557=CARTESIAN_POINT('Ctrl Pts',(7.74975542007111,5.26953472718861,9.24611567679825));
#81558=CARTESIAN_POINT('Ctrl Pts',(7.56971670678642,5.5249145167292,9.25156635365711));
#81559=CARTESIAN_POINT('Ctrl Pts',(7.47791291009582,5.64854935561786,9.25426825172031));
#81560=CARTESIAN_POINT('Ctrl Pts',(7.2643258184405,5.92185482634075,9.26036499693299));
#81561=CARTESIAN_POINT('Ctrl Pts',(7.14088190719151,6.07014002019938,9.26376124258444));
#81562=CARTESIAN_POINT('Ctrl Pts',(6.96054091037085,6.27365122676355,9.2685074930826));
#81563=CARTESIAN_POINT('Ctrl Pts',(6.90738629903688,6.33212792291947,9.26988153380585));
#81564=CARTESIAN_POINT('Ctrl Pts',(6.81053289056493,6.43600780235583,9.27233623655947));
#81565=CARTESIAN_POINT('Ctrl Pts',(6.76710368660461,6.48165583833664,9.2734198448776));
#81566=CARTESIAN_POINT('Ctrl Pts',(6.69647746403019,6.55440678838525,9.27515241146473));
#81567=CARTESIAN_POINT('Ctrl Pts',(6.66956855385851,6.58178654270764,9.2758056986922));
#81568=CARTESIAN_POINT('Ctrl Pts',(6.60532326079376,6.64635740498306,9.27734895453715));
#81569=CARTESIAN_POINT('Ctrl Pts',(6.56783995378636,6.68340036901566,9.27823658371734));
#81570=CARTESIAN_POINT('Ctrl Pts',(6.43789364531425,6.80967113921202,9.28127420167015));
#81571=CARTESIAN_POINT('Ctrl Pts',(6.34390877490551,6.8973123193857,9.28340344119814));
#81572=CARTESIAN_POINT('Ctrl Pts',(6.07034234467736,7.14209050971353,9.28945438486384));
#81573=CARTESIAN_POINT('Ctrl Pts',(5.88652160832528,7.29433867066382,9.29334826993278));
#81574=CARTESIAN_POINT('Ctrl Pts',(5.52441899195938,7.57163659008751,9.30084280293973));
#81575=CARTESIAN_POINT('Ctrl Pts',(5.34719633922741,7.697816361735,9.30443639328988));
#81576=CARTESIAN_POINT('Ctrl Pts',(5.08820500229021,7.86895116726165,9.30963251603522));
#81577=CARTESIAN_POINT('Ctrl Pts',(5.00990745746512,7.91903086453169,9.31119617815515));
#81578=CARTESIAN_POINT('Ctrl Pts',(4.86362667830771,8.0095552550443,9.31410680898949));
#81579=CARTESIAN_POINT('Ctrl Pts',(4.79585122892441,8.05031991946148,9.31545121184316));
#81580=CARTESIAN_POINT('Ctrl Pts',(4.63964198338355,8.14160169837309,9.31854126168806));
#81581=CARTESIAN_POINT('Ctrl Pts',(4.55088441073539,8.19154484569427,9.32029091250437));
#81582=CARTESIAN_POINT('Ctrl Pts',(4.40483248759764,8.27062050622593,9.32315990405494));
#81583=CARTESIAN_POINT('Ctrl Pts',(4.34802808787325,8.30062422716301,9.32427328759775));
#81584=CARTESIAN_POINT('Ctrl Pts',(4.29092661458802,8.33003804617484,9.32538978630507));
#81585=CARTESIAN_POINT('Origin',(0.,0.,2.15141010809499));
#81586=CARTESIAN_POINT('',(4.29126860009405,8.33070247396426,10.522886232912));
#81587=CARTESIAN_POINT('',(4.29092662690317,8.33003803983112,10.3254369059772));
#81588=CARTESIAN_POINT('',(4.29092662815669,8.33003803918541,2.15141010809499));
#81589=CARTESIAN_POINT('',(-9.36953457099031,3.84033400625157E-5,9.84861910993532));
#81590=CARTESIAN_POINT('Ctrl Pts',(-9.36948395328014,3.79045209737E-5,9.84858989190502));
#81591=CARTESIAN_POINT('Ctrl Pts',(-9.36936718066919,-0.814935059669627,
9.86242933876059));
#81592=CARTESIAN_POINT('Ctrl Pts',(-9.06438402558837,-3.17553663979636,
9.90251439004182));
#81593=CARTESIAN_POINT('Ctrl Pts',(-7.1048427973132,-6.69335858514711,9.9688450457487));
#81594=CARTESIAN_POINT('Ctrl Pts',(-3.07509487664221,-9.26410448038798,
10.0475818590257));
#81595=CARTESIAN_POINT('Ctrl Pts',(1.69204456314026,-9.61336702306967,10.1263186723027));
#81596=CARTESIAN_POINT('Ctrl Pts',(6.05344064836948,-7.65739489908703,10.2050554855796));
#81597=CARTESIAN_POINT('Ctrl Pts',(8.96325362003102,-3.8652198989057,10.2837922988566));
#81598=CARTESIAN_POINT('Ctrl Pts',(9.72372568736471,0.853814429943271,10.3625291121336));
#81599=CARTESIAN_POINT('Ctrl Pts',(8.15249966287939,5.36810856546769,10.4412659254106));
#81600=CARTESIAN_POINT('Ctrl Pts',(5.75868655187378,7.55886885973291,10.4947182990034));
#81601=CARTESIAN_POINT('Ctrl Pts',(4.34157152446891,8.30481265751835,10.5219250681705));
#81602=CARTESIAN_POINT('Ctrl Pts',(4.29126860009441,8.33070247396408,10.522886232912));
#81603=CARTESIAN_POINT('Ctrl Pts',(-9.37024999988976,4.54536311663567E-5,
9.84903207652725));
#81604=CARTESIAN_POINT('Ctrl Pts',(-9.37024974762411,0.0520499281900485,
9.84814461163007));
#81605=CARTESIAN_POINT('Ctrl Pts',(-9.36981656158823,0.104053458913103,
9.84725444355175));
#81606=CARTESIAN_POINT('Ctrl Pts',(-9.36789957813314,0.219145087514164,
9.84527828613022));
#81607=CARTESIAN_POINT('Ctrl Pts',(-9.36621133906909,0.282227233061156,
9.84419109651768));
#81608=CARTESIAN_POINT('Ctrl Pts',(-9.35520247250146,0.580777832043862,
9.8390270125095));
#81609=CARTESIAN_POINT('Ctrl Pts',(-9.33763858581784,0.815856103645878,
9.83490326508495));
#81610=CARTESIAN_POINT('Ctrl Pts',(-9.27856332103884,1.33971565203357,9.82564089655357));
#81611=CARTESIAN_POINT('Ctrl Pts',(-9.23239279194585,1.62772817421331,9.82049684806399));
#81612=CARTESIAN_POINT('Ctrl Pts',(-9.16301326767674,1.96038365300944,9.81462428506578));
#81613=CARTESIAN_POINT('Ctrl Pts',(-9.15279038805863,2.00757175076584,9.81379302783404));
#81614=CARTESIAN_POINT('Ctrl Pts',(-9.13376995447467,2.09220233701906,9.81230661095988));
#81615=CARTESIAN_POINT('Ctrl Pts',(-9.12510571381771,2.1296736648983,9.81165004482906));
#81616=CARTESIAN_POINT('Ctrl Pts',(-9.10699847921789,2.20584462395371,9.81031931725714));
#81617=CARTESIAN_POINT('Ctrl Pts',(-9.0975389093729,2.24453950786064,9.80964541056631));
#81618=CARTESIAN_POINT('Ctrl Pts',(-9.06899220921226,2.35816543529988,9.80767123382159));
#81619=CARTESIAN_POINT('Ctrl Pts',(-9.04922396630676,2.43292202167366,9.80637842426282));
#81620=CARTESIAN_POINT('Ctrl Pts',(-8.94337370986254,2.81405897278214,9.79980037592466));
#81621=CARTESIAN_POINT('Ctrl Pts',(-8.84264863934384,3.11615590514634,9.79462300969131));
#81622=CARTESIAN_POINT('Ctrl Pts',(-8.68837498155519,3.51067337539497,9.78766159179826));
#81623=CARTESIAN_POINT('Ctrl Pts',(-8.64834885809028,3.60815040641361,9.78592553120387));
#81624=CARTESIAN_POINT('Ctrl Pts',(-8.57980787977317,3.76737353073208,9.78305586700497));
#81625=CARTESIAN_POINT('Ctrl Pts',(-8.55224968151939,3.82952111136531,9.78192716972226));
#81626=CARTESIAN_POINT('Ctrl Pts',(-8.48179379436362,3.98385448775289,9.77910031506187));
#81627=CARTESIAN_POINT('Ctrl Pts',(-8.43806740645392,4.07565220900377,9.77739730208818));
#81628=CARTESIAN_POINT('Ctrl Pts',(-8.35935956885488,4.23419022927559,9.77441444012392));
#81629=CARTESIAN_POINT('Ctrl Pts',(-8.32505094184776,4.30125401316118,9.7731394182075));
#81630=CARTESIAN_POINT('Ctrl Pts',(-8.25079477081679,4.44218660673623,9.77043078646325));
#81631=CARTESIAN_POINT('Ctrl Pts',(-8.21065528678723,4.51594684649965,9.7689958818351));
#81632=CARTESIAN_POINT('Ctrl Pts',(-8.0985975445243,4.71542988388175,9.76506721782281));
#81633=CARTESIAN_POINT('Ctrl Pts',(-8.02474732280894,4.84004043338668,9.76256006691141));
#81634=CARTESIAN_POINT('Ctrl Pts',(-7.77585480204574,5.2386404171029,9.75437404140671));
#81635=CARTESIAN_POINT('Ctrl Pts',(-7.58943709331942,5.50524430743699,9.74862968388853));
#81636=CARTESIAN_POINT('Ctrl Pts',(-7.32903756728009,5.83921879721361,9.74121366945544));
#81637=CARTESIAN_POINT('Ctrl Pts',(-7.26731361530268,5.91586178832416,9.73949644827523));
#81638=CARTESIAN_POINT('Ctrl Pts',(-7.16929080085027,6.03372756372094,9.7368391180679));
#81639=CARTESIAN_POINT('Ctrl Pts',(-7.1338173722374,6.07562742567897,9.73589114609851));
#81640=CARTESIAN_POINT('Ctrl Pts',(-7.07171151984965,6.14769062591785,9.73425661573435));
#81641=CARTESIAN_POINT('Ctrl Pts',(-7.04524924007102,6.17799862454553,9.73356788713856));
#81642=CARTESIAN_POINT('Ctrl Pts',(-6.99038002590721,6.2400308838965,9.73215642384123));
#81643=CARTESIAN_POINT('Ctrl Pts',(-6.96195046996255,6.2717337309615,9.73143423670698));
#81644=CARTESIAN_POINT('Ctrl Pts',(-6.89647052485058,6.34375896771048,9.72979080349397));
#81645=CARTESIAN_POINT('Ctrl Pts',(-6.85928079487896,6.38395257931692,9.72887158413273));
#81646=CARTESIAN_POINT('Ctrl Pts',(-6.59946348466353,6.65986425235365,9.72253812629533));
#81647=CARTESIAN_POINT('Ctrl Pts',(-6.36508351529453,6.8842155563636,9.71726072590991));
#81648=CARTESIAN_POINT('Ctrl Pts',(-5.93965687468235,7.25110258736728,9.70803923335513));
#81649=CARTESIAN_POINT('Ctrl Pts',(-5.75393369285374,7.39934180084282,9.70412111269622));
#81650=CARTESIAN_POINT('Ctrl Pts',(-5.48685033527731,7.59637817479089,9.69856826591055));
#81651=CARTESIAN_POINT('Ctrl Pts',(-5.4100798096171,7.6512433221824,9.69698146893474));
#81652=CARTESIAN_POINT('Ctrl Pts',(-5.26756155546809,7.74987845294711,9.69404995902405));
#81653=CARTESIAN_POINT('Ctrl Pts',(-5.2020638203045,7.79399465946988,9.69270810277671));
#81654=CARTESIAN_POINT('Ctrl Pts',(-5.05245420713939,7.89203857983942,9.68965421081878));
#81655=CARTESIAN_POINT('Ctrl Pts',(-4.96802172762202,7.94545949007751,9.6879385360291));
#81656=CARTESIAN_POINT('Ctrl Pts',(-4.6123131296426,8.16263139348787,9.68074305000772));
#81657=CARTESIAN_POINT('Ctrl Pts',(-4.33367501773777,8.31391862634465,9.67517666434931));
#81658=CARTESIAN_POINT('Ctrl Pts',(-3.90484276208053,8.5193282001683,9.66681736999822));
#81659=CARTESIAN_POINT('Ctrl Pts',(-3.76005679862803,8.58421359019149,9.6640304442582));
#81660=CARTESIAN_POINT('Ctrl Pts',(-3.54766125799607,8.67299295073623,9.6600191147831));
#81661=CARTESIAN_POINT('Ctrl Pts',(-3.48131487885573,8.69983642768055,9.65877685003699));
#81662=CARTESIAN_POINT('Ctrl Pts',(-3.35998793109808,8.74731466579623,9.65652834389364));
#81663=CARTESIAN_POINT('Ctrl Pts',(-3.3051084299359,8.7681977080831,9.65551983087911));
#81664=CARTESIAN_POINT('Ctrl Pts',(-3.21438645160945,8.8017469577506,9.65386871577831));
#81665=CARTESIAN_POINT('Ctrl Pts',(-3.17865687575951,8.81471328201536,9.65322261236271));
#81666=CARTESIAN_POINT('Ctrl Pts',(-3.09124649999818,8.84583407691863,9.65165214028041));
#81667=CARTESIAN_POINT('Ctrl Pts',(-3.03948358654614,8.86375343664419,9.65073054789263));
#81668=CARTESIAN_POINT('Ctrl Pts',(-2.82958851631258,8.93436035992963,9.64702229241396));
#81669=CARTESIAN_POINT('Ctrl Pts',(-2.67022025543596,8.9832783726295,9.64427184140417));
#81670=CARTESIAN_POINT('Ctrl Pts',(-2.25388039479043,9.09901486867829,9.63717124727921));
#81671=CARTESIAN_POINT('Ctrl Pts',(-1.99522349845942,9.15921021058904,9.6328397228581));
#81672=CARTESIAN_POINT('Ctrl Pts',(-1.61819653155814,9.23022198285666,9.62650685270609));
#81673=CARTESIAN_POINT('Ctrl Pts',(-1.50162896872437,9.24990098466322,9.62454690799501));
#81674=CARTESIAN_POINT('Ctrl Pts',(-1.28315502308573,9.2825451309883,9.62086043098271));
#81675=CARTESIAN_POINT('Ctrl Pts',(-1.18134708126341,9.29605023260777,9.61913730267377));
#81676=CARTESIAN_POINT('Ctrl Pts',(-1.00083840925674,9.31698194567585,9.61606918747457));
#81677=CARTESIAN_POINT('Ctrl Pts',(-0.922226994541179,9.32509128289532,
9.61472872119132));
#81678=CARTESIAN_POINT('Ctrl Pts',(-0.750320111469826,9.34062966048367,
9.61178694211199));
#81679=CARTESIAN_POINT('Ctrl Pts',(-0.656996884485406,9.34765734088302,
9.61018321132451));
#81680=CARTESIAN_POINT('Ctrl Pts',(-0.159085799734555,9.37765907867496,
9.60159053004482));
#81681=CARTESIAN_POINT('Ctrl Pts',(0.246566480881064,9.37576660647323,9.59444130340288));
#81682=CARTESIAN_POINT('Ctrl Pts',(0.821122688949824,9.33576390710877,9.58433471452698));
#81683=CARTESIAN_POINT('Ctrl Pts',(0.991074477874135,9.31925436161385,9.58135095911158));
#81684=CARTESIAN_POINT('Ctrl Pts',(1.21544711270105,9.2912508188199,9.57745358147534));
#81685=CARTESIAN_POINT('Ctrl Pts',(1.27035196925926,9.28390323922144,9.57650327199206));
#81686=CARTESIAN_POINT('Ctrl Pts',(1.36706241237875,9.27008708871701,9.57483722031274));
#81687=CARTESIAN_POINT('Ctrl Pts',(1.40889514008422,9.26382149866546,9.57411931704548));
#81688=CARTESIAN_POINT('Ctrl Pts',(1.51285476689746,9.2475302438798,9.57234152044998));
#81689=CARTESIAN_POINT('Ctrl Pts',(1.57492569933575,9.23716158921034,9.5712854173374));
#81690=CARTESIAN_POINT('Ctrl Pts',(1.88481357589713,9.18218192864615,9.56603012210176));
#81691=CARTESIAN_POINT('Ctrl Pts',(2.130866718515,9.12821971109235,9.56191004885437));
#81692=CARTESIAN_POINT('Ctrl Pts',(2.64710362672033,8.99299004396167,9.55316307358536));
#81693=CARTESIAN_POINT('Ctrl Pts',(2.91639769053659,8.90930140530272,9.54853743418999));
#81694=CARTESIAN_POINT('Ctrl Pts',(3.27807339161354,8.77874477158698,9.54212035097174));
#81695=CARTESIAN_POINT('Ctrl Pts',(3.3740588222899,8.74230243818654,9.54039770043964));
#81696=CARTESIAN_POINT('Ctrl Pts',(3.54283326637152,8.67503096623534,9.53733009158272));
#81697=CARTESIAN_POINT('Ctrl Pts',(3.61586749603739,8.64484424589884,9.53598964806143));
#81698=CARTESIAN_POINT('Ctrl Pts',(3.77455683394854,8.57689146887311,9.53304753445643));
#81699=CARTESIAN_POINT('Ctrl Pts',(3.86004554597474,8.53875839272353,9.53144344226448));
#81700=CARTESIAN_POINT('Ctrl Pts',(4.06144905723485,8.44527755315026,9.52761849528154));
#81701=CARTESIAN_POINT('Ctrl Pts',(4.17679897906308,8.38882689144013,9.52539107763482));
#81702=CARTESIAN_POINT('Ctrl Pts',(4.29092667702531,8.33003801401246,9.52315240206829));
#81703=CARTESIAN_POINT('Ctrl Pts',(4.29092661458801,8.33003804617484,9.32538978630507));
#81704=CARTESIAN_POINT('Ctrl Pts',(4.03195386670708,8.46343876417583,9.33045345141923));
#81705=CARTESIAN_POINT('Ctrl Pts',(3.76687068924532,8.58470572170595,9.33558688684702));
#81706=CARTESIAN_POINT('Ctrl Pts',(3.31896268203108,8.76485628035645,9.34406654540643));
#81707=CARTESIAN_POINT('Ctrl Pts',(3.13924074862046,8.83082027695114,9.34741784325804));
#81708=CARTESIAN_POINT('Ctrl Pts',(2.9039949514902,8.90907362156652,9.3516929856681));
#81709=CARTESIAN_POINT('Ctrl Pts',(2.85020474931201,8.92642775021501,9.35266301114549));
#81710=CARTESIAN_POINT('Ctrl Pts',(2.75597499661287,8.95589015575653,9.3543472864938));
#81711=CARTESIAN_POINT('Ctrl Pts',(2.7156047370626,8.96821373414142,9.35506393320161));
#81712=CARTESIAN_POINT('Ctrl Pts',(2.61626987464547,8.99780483390906,9.35681564259426));
#81713=CARTESIAN_POINT('Ctrl Pts',(2.55721617472214,9.01476596183512,9.35784722157616));
#81714=CARTESIAN_POINT('Ctrl Pts',(2.19185847909412,9.11582329857587,9.36418022467171));
#81715=CARTESIAN_POINT('Ctrl Pts',(1.88160822869861,9.18488052119056,9.36935248666992));
#81716=CARTESIAN_POINT('Ctrl Pts',(1.40585615884353,9.26565445627061,9.37727224953256));
#81717=CARTESIAN_POINT('Ctrl Pts',(1.24256161270218,9.28896251107406,9.37998707829357));
#81718=CARTESIAN_POINT('Ctrl Pts',(0.952056619930774,9.32263036054288,9.38484104708303));
#81719=CARTESIAN_POINT('Ctrl Pts',(0.825089541315198,9.33472419379216,9.38697050552061));
#81720=CARTESIAN_POINT('Ctrl Pts',(0.616152079787817,9.35032963192814,9.39049588610954));
#81721=CARTESIAN_POINT('Ctrl Pts',(0.534312166825084,9.35536306523416,9.39188201760079));
#81722=CARTESIAN_POINT('Ctrl Pts',(0.378378712063795,9.36290067605776,9.3945344184598));
#81723=CARTESIAN_POINT('Ctrl Pts',(0.304300799970728,9.36560091583814,9.39579932908));
#81724=CARTESIAN_POINT('Ctrl Pts',(0.100489631490954,9.37060945262223,9.39929337241661));
#81725=CARTESIAN_POINT('Ctrl Pts',(-0.0292713981281078,9.37110253526522,
9.40153356066672));
#81726=CARTESIAN_POINT('Ctrl Pts',(-0.487088472794289,9.36333288012718,
9.40948794086229));
#81727=CARTESIAN_POINT('Ctrl Pts',(-0.814657004363527,9.34053480480239,
9.41527917770297));
#81728=CARTESIAN_POINT('Ctrl Pts',(-1.30388664945109,9.28055012118306,9.42392540199743));
#81729=CARTESIAN_POINT('Ctrl Pts',(-1.46686521689535,9.25618915325333,9.4268033891527));
#81730=CARTESIAN_POINT('Ctrl Pts',(-1.68327001953415,9.21798302666872,9.43059049158773));
#81731=CARTESIAN_POINT('Ctrl Pts',(-1.73733809467374,9.20794577536662,9.43153375404264));
#81732=CARTESIAN_POINT('Ctrl Pts',(-1.83287618305926,9.18933854177397,9.43319347771691));
#81733=CARTESIAN_POINT('Ctrl Pts',(-1.87438208356734,9.18096235396794,9.43391201496386));
#81734=CARTESIAN_POINT('Ctrl Pts',(-1.9779955273892,9.15932049385449,9.43570007594577));
#81735=CARTESIAN_POINT('Ctrl Pts',(-2.04002755989652,9.14570422643407,9.43676569056657));
#81736=CARTESIAN_POINT('Ctrl Pts',(-2.27798699308665,9.09092975027342,9.44084224748833));
#81737=CARTESIAN_POINT('Ctrl Pts',(-2.45284902290051,9.0453170476123,9.44381486217189));
#81738=CARTESIAN_POINT('Ctrl Pts',(-2.73830229590598,8.96196985483505,9.44869410655845));
#81739=CARTESIAN_POINT('Ctrl Pts',(-2.84970069272937,8.92717251490891,9.45060485667693));
#81740=CARTESIAN_POINT('Ctrl Pts',(-3.1249073818841,8.83553026856915,9.45536293490086));
#81741=CARTESIAN_POINT('Ctrl Pts',(-3.28784270638461,8.77620256449062,9.45821397125729));
#81742=CARTESIAN_POINT('Ctrl Pts',(-3.50676049499352,8.68953796035684,9.46211911492545));
#81743=CARTESIAN_POINT('Ctrl Pts',(-3.56425453046974,8.66611382123478,9.46315174656721));
#81744=CARTESIAN_POINT('Ctrl Pts',(-3.71605103224567,8.60250295156872,9.46589857868443));
#81745=CARTESIAN_POINT('Ctrl Pts',(-3.80993395611077,8.56133724881142,9.46761862800888));
#81746=CARTESIAN_POINT('Ctrl Pts',(-3.974955731117,8.48572656250711,9.47068348660121));
#81747=CARTESIAN_POINT('Ctrl Pts',(-4.0463697734286,8.451906292723,9.47202381269341));
#81748=CARTESIAN_POINT('Ctrl Pts',(-4.20153121473128,8.37600759084149,9.47496777637325));
#81749=CARTESIAN_POINT('Ctrl Pts',(-4.28509235027471,8.33356773563355,9.47657385867571));
#81750=CARTESIAN_POINT('Ctrl Pts',(-4.72435785518277,8.10211534927251,9.48512727306745));
#81751=CARTESIAN_POINT('Ctrl Pts',(-5.06823393754072,7.89156711337965,9.49223253473872));
#81752=CARTESIAN_POINT('Ctrl Pts',(-5.5384719377203,7.56020234115585,9.50232805073771));
#81753=CARTESIAN_POINT('Ctrl Pts',(-5.67668490589927,7.45698193683747,9.50534288132208));
#81754=CARTESIAN_POINT('Ctrl Pts',(-5.85550806685538,7.31557865764241,9.50927252240919));
#81755=CARTESIAN_POINT('Ctrl Pts',(-5.89873904376682,7.28076531209686,9.51022478267901));
#81756=CARTESIAN_POINT('Ctrl Pts',(-5.974357769707,7.21875492068353,9.5118926073746));
#81757=CARTESIAN_POINT('Ctrl Pts',(-6.00687529009995,7.19171903079481,9.51261035630734));
#81758=CARTESIAN_POINT('Ctrl Pts',(-6.08720596864857,7.12400513653154,9.51438541742146));
#81759=CARTESIAN_POINT('Ctrl Pts',(-6.13479539615825,7.08306509666565,9.51543897126861));
#81760=CARTESIAN_POINT('Ctrl Pts',(-6.37276443549706,6.87414851277008,9.5207268618826));
#81761=CARTESIAN_POINT('Ctrl Pts',(-6.55667311383526,6.69896133036394,9.52488055410098));
#81762=CARTESIAN_POINT('Ctrl Pts',(-6.92633141750336,6.31700938178691,9.53359293971307));
#81763=CARTESIAN_POINT('Ctrl Pts',(-7.11045903993934,6.10901351860957,9.53814999706784));
#81764=CARTESIAN_POINT('Ctrl Pts',(-7.35024905648573,5.81258648169658,9.5445112572555));
#81765=CARTESIAN_POINT('Ctrl Pts',(-7.41407880064955,5.73094741444385,9.54624960282394));
#81766=CARTESIAN_POINT('Ctrl Pts',(-7.52421327207485,5.58516376609647,9.54933392043113));
#81767=CARTESIAN_POINT('Ctrl Pts',(-7.57108442372572,5.52145997656743,9.55067518687867));
#81768=CARTESIAN_POINT('Ctrl Pts',(-7.6712769460494,5.38161079920131,9.55360674545033));
#81769=CARTESIAN_POINT('Ctrl Pts',(-7.72428305133752,5.30524985893696,9.55519932796924));
#81770=CARTESIAN_POINT('Ctrl Pts',(-7.88924684219942,5.05988748740033,9.56029135120862));
#81771=CARTESIAN_POINT('Ctrl Pts',(-7.99686035958828,4.88803652246012,9.56382154466096));
#81772=CARTESIAN_POINT('Ctrl Pts',(-8.22788491704698,4.49102992423959,9.57187006718879));
#81773=CARTESIAN_POINT('Ctrl Pts',(-8.34778847267389,4.26402010317994,9.57639931994303));
#81774=CARTESIAN_POINT('Ctrl Pts',(-8.48548882411757,3.9751828837433,9.58199567596121));
#81775=CARTESIAN_POINT('Ctrl Pts',(-8.51217425262138,3.91771477420357,9.5831009738114));
#81776=CARTESIAN_POINT('Ctrl Pts',(-8.57292277155079,3.78333907937482,9.58566345317276));
#81777=CARTESIAN_POINT('Ctrl Pts',(-8.60653733217042,3.70623456373532,9.5871172331749));
#81778=CARTESIAN_POINT('Ctrl Pts',(-8.65663929268137,3.5869527921276,9.58933559207532));
#81779=CARTESIAN_POINT('Ctrl Pts',(-8.67386665471468,3.54509117666246,9.59010836817494));
#81780=CARTESIAN_POINT('Ctrl Pts',(-8.70840352038536,3.45940932067852,9.59167719122824));
#81781=CARTESIAN_POINT('Ctrl Pts',(-8.72568722142075,3.41558007495524,9.59247294514734));
#81782=CARTESIAN_POINT('Ctrl Pts',(-8.77687615482799,3.28284682051177,9.59486499276071));
#81783=CARTESIAN_POINT('Ctrl Pts',(-8.80975856340142,3.19355482422796,9.596450197656));
#81784=CARTESIAN_POINT('Ctrl Pts',(-8.97175681844046,2.73209415675855,9.60455267378654));
#81785=CARTESIAN_POINT('Ctrl Pts',(-9.07867054082573,2.35255224189992,9.61093634227378));
#81786=CARTESIAN_POINT('Ctrl Pts',(-9.17571145966846,1.90067441587618,9.61858676474256));
#81787=CARTESIAN_POINT('Ctrl Pts',(-9.18931321881071,1.83378476824568,9.6197199360753));
#81788=CARTESIAN_POINT('Ctrl Pts',(-9.22275520653687,1.65960118615181,9.62267504954877));
#81789=CARTESIAN_POINT('Ctrl Pts',(-9.24145435870355,1.55209888607979,9.62450316030754));
#81790=CARTESIAN_POINT('Ctrl Pts',(-9.27053645623702,1.36567574796332,9.62768533650688));
#81791=CARTESIAN_POINT('Ctrl Pts',(-9.28179912522165,1.28690380360389,9.62903359317636));
#81792=CARTESIAN_POINT('Ctrl Pts',(-9.30364364642972,1.11887329046776,9.63191851110152));
#81793=CARTESIAN_POINT('Ctrl Pts',(-9.31394728413052,1.02958655737983,9.63345682088396));
#81794=CARTESIAN_POINT('Ctrl Pts',(-9.34159453834653,0.755428062834336,
9.63819708275899));
#81795=CARTESIAN_POINT('Ctrl Pts',(-9.35472909901267,0.570178209122063,
9.64142424983722));
#81796=CARTESIAN_POINT('Ctrl Pts',(-9.36496457604756,0.321054768496945,
9.6457860800192));
#81797=CARTESIAN_POINT('Ctrl Pts',(-9.36692964016035,0.257423353421096,
9.64690199720882));
#81798=CARTESIAN_POINT('Ctrl Pts',(-9.36958360770654,0.12911589718899,9.64915451793947));
#81799=CARTESIAN_POINT('Ctrl Pts',(-9.37025159845246,0.064442796714051,
9.65029110781168));
#81800=CARTESIAN_POINT('Ctrl Pts',(-9.37024358895048,-0.259047479483722,
9.65597809842893));
#81801=CARTESIAN_POINT('Ctrl Pts',(-9.35951408025761,-0.517751976556725,
9.66053531542523));
#81802=CARTESIAN_POINT('Ctrl Pts',(-9.33293198962286,-0.837762740394519,
9.66608396316692));
#81803=CARTESIAN_POINT('Ctrl Pts',(-9.32715600163992,-0.899792686609805,
9.66715516455485));
#81804=CARTESIAN_POINT('Ctrl Pts',(-9.31642463142568,-1.00379419831254,
9.66894143775335));
#81805=CARTESIAN_POINT('Ctrl Pts',(-9.31180311198124,-1.04579803244511,
9.66966008853402));
#81806=CARTESIAN_POINT('Ctrl Pts',(-9.30041346314148,-1.14324726840369,
9.67132068835133));
#81807=CARTESIAN_POINT('Ctrl Pts',(-9.29343340020085,-1.19866615767885,
9.67226031462418));
#81808=CARTESIAN_POINT('Ctrl Pts',(-9.2620913657378,-1.43075253853213,9.6761810893079));
#81809=CARTESIAN_POINT('Ctrl Pts',(-9.23318381867372,-1.60676888386266,
9.67912060677995));
#81810=CARTESIAN_POINT('Ctrl Pts',(-9.12516184268949,-2.16445983477208,
9.68844857363957));
#81811=CARTESIAN_POINT('Ctrl Pts',(-9.02725585264652,-2.54206937849595,
9.69480125181812));
#81812=CARTESIAN_POINT('Ctrl Pts',(-8.87634208554641,-3.00355062240493,
9.70292052773782));
#81813=CARTESIAN_POINT('Ctrl Pts',(-8.84516634645638,-3.09415536256451,
9.70453113878462));
#81814=CARTESIAN_POINT('Ctrl Pts',(-8.78847859361354,-3.25104140297041,
9.70735159396909));
#81815=CARTESIAN_POINT('Ctrl Pts',(-8.76359239414913,-3.31754043214808,
9.70855710340201));
#81816=CARTESIAN_POINT('Ctrl Pts',(-8.70346618504043,-3.47280602909746,
9.71139612319075));
#81817=CARTESIAN_POINT('Ctrl Pts',(-8.66762011776722,-3.56132935650102,
9.71303364994337));
#81818=CARTESIAN_POINT('Ctrl Pts',(-8.52908317945916,-3.88896384342072,
9.7191652373926));
#81819=CARTESIAN_POINT('Ctrl Pts',(-8.41779952544404,-4.12431204797088,
9.72371534481235));
#81820=CARTESIAN_POINT('Ctrl Pts',(-8.15585355459549,-4.62338652996406,
9.73361778681148));
#81821=CARTESIAN_POINT('Ctrl Pts',(-8.00187477903875,-4.88504356293677,
9.73897343965614));
#81822=CARTESIAN_POINT('Ctrl Pts',(-7.80665175202878,-5.18271507167016,
9.74511573233332));
#81823=CARTESIAN_POINT('Ctrl Pts',(-7.77746063282999,-5.2264187750404,9.7460186516215));
#81824=CARTESIAN_POINT('Ctrl Pts',(-7.72411063671725,-5.30485529244543,
9.74763957931448));
#81825=CARTESIAN_POINT('Ctrl Pts',(-7.70008131063667,-5.33967439344528,
9.74835918281124));
#81826=CARTESIAN_POINT('Ctrl Pts',(-7.64408135382787,-5.41965560677047,
9.75001199453729));
#81827=CARTESIAN_POINT('Ctrl Pts',(-7.61194491914114,-5.4646995532118,9.75094299131173));
#81828=CARTESIAN_POINT('Ctrl Pts',(-7.47959141150761,-5.6467795316409,9.75471237306425));
#81829=CARTESIAN_POINT('Ctrl Pts',(-7.37605755223019,-5.78136507104649,
9.75751311880526));
#81830=CARTESIAN_POINT('Ctrl Pts',(-7.01236547097728,-6.22845145238243,
9.76698166705506));
#81831=CARTESIAN_POINT('Ctrl Pts',(-6.73555294790581,-6.52680653794717,
9.77360304184834));
#81832=CARTESIAN_POINT('Ctrl Pts',(-6.37231870554139,-6.87050822425527,
9.78197190944461));
#81833=CARTESIAN_POINT('Ctrl Pts',(-6.3034389444158,-6.93375701660995,9.78354488189183));
#81834=CARTESIAN_POINT('Ctrl Pts',(-6.17461756645689,-7.04854091761982,
9.78646380293057));
#81835=CARTESIAN_POINT('Ctrl Pts',(-6.11494821616971,-7.10036896499729,
9.78780706802258));
#81836=CARTESIAN_POINT('Ctrl Pts',(-5.97617340185612,-7.21786008568665,
9.79091213425945));
#81837=CARTESIAN_POINT('Ctrl Pts',(-5.8966287278457,-7.28298855686858,9.79267814776122));
#81838=CARTESIAN_POINT('Ctrl Pts',(-5.76714118453818,-7.38549628720978,
9.79553091301787));
#81839=CARTESIAN_POINT('Ctrl Pts',(-5.71786863286161,-7.42370871828058,
9.79661143902064));
#81840=CARTESIAN_POINT('Ctrl Pts',(-5.52920715715587,-7.5670290944832,9.80072893218102));
#81841=CARTESIAN_POINT('Ctrl Pts',(-5.38727216035137,-7.66872607079314,
9.80378683133338));
#81842=CARTESIAN_POINT('Ctrl Pts',(-4.98682264548113,-7.93904293532666,
9.81227435301447));
#81843=CARTESIAN_POINT('Ctrl Pts',(-4.72269351334376,-8.09894864659562,
9.81772228609287));
#81844=CARTESIAN_POINT('Ctrl Pts',(-4.40558604622563,-8.27013171682081,
9.82393826689908));
#81845=CARTESIAN_POINT('Ctrl Pts',(-4.3598112718619,-8.29435426740229,9.82482774298874));
#81846=CARTESIAN_POINT('Ctrl Pts',(-4.2763438906194,-8.33764066683544,9.8264339927257));
#81847=CARTESIAN_POINT('Ctrl Pts',(-4.23871879245749,-8.35683145536787,
9.82715222903956));
#81848=CARTESIAN_POINT('Ctrl Pts',(-4.15080318801228,-8.4009265653471,9.82881678798085));
#81849=CARTESIAN_POINT('Ctrl Pts',(-4.10041625598607,-8.42563474221881,
9.8297607323785));
#81850=CARTESIAN_POINT('Ctrl Pts',(-3.88466274348786,-8.52903974838739,
9.83376579403471));
#81851=CARTESIAN_POINT('Ctrl Pts',(-3.71722965249949,-8.60333236482007,
9.83678295736674));
#81852=CARTESIAN_POINT('Ctrl Pts',(-3.18824879321056,-8.81972240889044,
9.8461656271432));
#81853=CARTESIAN_POINT('Ctrl Pts',(-2.81997669327092,-8.94428113492334,
9.852499443628));
#81854=CARTESIAN_POINT('Ctrl Pts',(-2.35386133549086,-9.07027247794415,
9.86057740704464));
#81855=CARTESIAN_POINT('Ctrl Pts',(-2.26231545268818,-9.09353807649935,
9.86216576435602));
#81856=CARTESIAN_POINT('Ctrl Pts',(-2.09362052017528,-9.13370532419569,
9.86509872029589));
#81857=CARTESIAN_POINT('Ctrl Pts',(-2.01657938627992,-9.15102329670546,
9.86644044284018));
#81858=CARTESIAN_POINT('Ctrl Pts',(-1.84002220860776,-9.18837343863706,
9.86952143020735));
#81859=CARTESIAN_POINT('Ctrl Pts',(-1.74038111291792,-9.20776637889404,
9.87126465783764));
#81860=CARTESIAN_POINT('Ctrl Pts',(-1.52606764319236,-9.24587466851182,
9.87502339841439));
#81861=CARTESIAN_POINT('Ctrl Pts',(-1.41132234542842,-9.26408387193702,
9.87704156786157));
#81862=CARTESIAN_POINT('Ctrl Pts',(-1.04453288943186,-9.31531767021668,
9.88350482828411));
#81863=CARTESIAN_POINT('Ctrl Pts',(-0.791471129584119,-9.3402229772792,
9.88798485372612));
#81864=CARTESIAN_POINT('Ctrl Pts',(-0.35766752165376,-9.3651578686177,9.89561376672246));
#81865=CARTESIAN_POINT('Ctrl Pts',(-0.177361926881824,-9.37030687927314,
9.89876879652595));
#81866=CARTESIAN_POINT('Ctrl Pts',(0.0588891785469922,-9.37023174565514,
9.90284269214161));
#81867=CARTESIAN_POINT('Ctrl Pts',(0.114797201998923,-9.36971357750192,
9.90380229020137));
#81868=CARTESIAN_POINT('Ctrl Pts',(0.212875920683018,-9.36792658652917,
9.90547596270072));
#81869=CARTESIAN_POINT('Ctrl Pts',(0.255048706833781,-9.36687326974289,
9.90619231046621));
#81870=CARTESIAN_POINT('Ctrl Pts',(0.358103001206895,-9.36360286478244,
9.90793506744506));
#81871=CARTESIAN_POINT('Ctrl Pts',(0.418972653271255,-9.36107677080669,
9.90895809982717));
#81872=CARTESIAN_POINT('Ctrl Pts',(0.555077681256161,-9.35409821581126,
9.9112353263616));
#81873=CARTESIAN_POINT('Ctrl Pts',(0.630292761214921,-9.34933129862128,
9.91248675054797));
#81874=CARTESIAN_POINT('Ctrl Pts',(0.88027935557292,-9.33045741555708,9.91663281677526));
#81875=CARTESIAN_POINT('Ctrl Pts',(1.05471181424678,-9.31235257618543,9.91950489440887));
#81876=CARTESIAN_POINT('Ctrl Pts',(1.50919004826045,-9.25224709061706,9.92701884197792));
#81877=CARTESIAN_POINT('Ctrl Pts',(1.78801986441566,-9.20242985800251,9.9316630122928));
#81878=CARTESIAN_POINT('Ctrl Pts',(2.16479118799068,-9.11734096523421,9.93810639296833));
#81879=CARTESIAN_POINT('Ctrl Pts',(2.26503523445243,-9.09295565157567,9.93983661510628));
#81880=CARTESIAN_POINT('Ctrl Pts',(2.4414824316134,-9.04693426771318,9.94291412478002));
#81881=CARTESIAN_POINT('Ctrl Pts',(2.51785231068971,-9.02597783156358,9.94425682685667));
#81882=CARTESIAN_POINT('Ctrl Pts',(2.68241691613286,-8.97856898476106,9.94717443915054));
#81883=CARTESIAN_POINT('Ctrl Pts',(2.77050598193635,-8.95177960393573,9.94875145966676));
#81884=CARTESIAN_POINT('Ctrl Pts',(3.05560844493263,-8.86046365535634,9.95390573533058));
#81885=CARTESIAN_POINT('Ctrl Pts',(3.25087767545638,-8.79069695728085,9.95751585593953));
#81886=CARTESIAN_POINT('Ctrl Pts',(3.66366784875799,-8.62757666542081,9.96529382930089));
#81887=CARTESIAN_POINT('Ctrl Pts',(3.88029324998445,-8.53234231505328,9.96946621869982));
#81888=CARTESIAN_POINT('Ctrl Pts',(4.21864521747847,-8.36804047238172,9.97605365122695));
#81889=CARTESIAN_POINT('Ctrl Pts',(4.34283050140176,-8.30426951834388,9.97848655990627));
#81890=CARTESIAN_POINT('Ctrl Pts',(4.51325602011697,-8.21188470577031,9.98182637580691));
#81891=CARTESIAN_POINT('Ctrl Pts',(4.56074158649539,-8.18560727883163,9.98275702292428));
#81892=CARTESIAN_POINT('Ctrl Pts',(4.64494607027385,-8.13805024875633,9.98440568117488));
#81893=CARTESIAN_POINT('Ctrl Pts',(4.68175361218616,-8.1169310064189,9.98512561672085));
#81894=CARTESIAN_POINT('Ctrl Pts',(4.77423451743203,-8.06302944789251,9.98693340132294));
#81895=CARTESIAN_POINT('Ctrl Pts',(4.82971465980063,-8.02992001443279,9.98801711641608));
#81896=CARTESIAN_POINT('Ctrl Pts',(5.10596503801475,-7.86116054582482,9.99341959155332));
#81897=CARTESIAN_POINT('Ctrl Pts',(5.32138474383488,-7.71696763199003,9.99765609796726));
#81898=CARTESIAN_POINT('Ctrl Pts',(5.61283675979855,-7.5038682782924,10.0035744018121));
#81899=CARTESIAN_POINT('Ctrl Pts',(5.69413472440661,-7.4423655750336,10.0052461634472));
#81900=CARTESIAN_POINT('Ctrl Pts',(5.93011288971839,-7.25771534454979,10.0101753126293));
#81901=CARTESIAN_POINT('Ctrl Pts',(6.0819175931054,-7.13098513228169,10.0134465010815));
#81902=CARTESIAN_POINT('Ctrl Pts',(6.29880186446494,-6.93795809258288,10.0183069684175));
#81903=CARTESIAN_POINT('Ctrl Pts',(6.36708711737817,-6.87534501025839,10.0198657758053));
#81904=CARTESIAN_POINT('Ctrl Pts',(6.49140104026012,-6.75791675334553,10.0227593995406));
#81905=CARTESIAN_POINT('Ctrl Pts',(6.5476921027984,-6.70339126148892,10.0240915927329));
#81906=CARTESIAN_POINT('Ctrl Pts',(6.67679546625164,-6.57515931750424,10.0271993824212));
#81907=CARTESIAN_POINT('Ctrl Pts',(6.74908248183686,-6.50093864979676,10.0289794612467));
#81908=CARTESIAN_POINT('Ctrl Pts',(6.99631005643468,-6.23852894797105,10.0352084125642));
#81909=CARTESIAN_POINT('Ctrl Pts',(7.16472974978712,-6.04435642627596,10.0397083122808));
#81910=CARTESIAN_POINT('Ctrl Pts',(7.4995418505116,-5.62466276451453,10.0491445588355));
#81911=CARTESIAN_POINT('Ctrl Pts',(7.66423248166289,-5.39810152453402,10.0540796025458));
#81912=CARTESIAN_POINT('Ctrl Pts',(7.84856231051454,-5.11904516081682,10.0598546207685));
#81913=CARTESIAN_POINT('Ctrl Pts',(7.87819533098797,-5.07332159876972,10.0607913574135));
#81914=CARTESIAN_POINT('Ctrl Pts',(7.93025297572879,-4.99144094248541,10.0624502660807));
#81915=CARTESIAN_POINT('Ctrl Pts',(7.95283328991462,-4.95538470997463,10.0631743605529));
#81916=CARTESIAN_POINT('Ctrl Pts',(8.00330636277727,-4.87355571612625,10.0648027808887));
#81917=CARTESIAN_POINT('Ctrl Pts',(8.03105343390526,-4.82769497937798,10.0657052683927));
#81918=CARTESIAN_POINT('Ctrl Pts',(8.13362829384361,-4.65482605398787,10.0690737660567));
#81919=CARTESIAN_POINT('Ctrl Pts',(8.20584928938428,-4.52629566972687,10.071511623549));
#81920=CARTESIAN_POINT('Ctrl Pts',(8.35771802366737,-4.24042620322682,10.0768386037089));
#81921=CARTESIAN_POINT('Ctrl Pts',(8.43601774708716,-4.08243427465195,10.079721745573));
#81922=CARTESIAN_POINT('Ctrl Pts',(8.61304511349541,-3.69835878634989,10.0866598002569));
#81923=CARTESIAN_POINT('Ctrl Pts',(8.70739405120004,-3.47040230679455,10.0907222646891));
#81924=CARTESIAN_POINT('Ctrl Pts',(8.82613240427037,-3.14807237852955,10.0964645423729));
#81925=CARTESIAN_POINT('Ctrl Pts',(8.85821219937101,-3.05664022915963,10.0980927746213));
#81926=CARTESIAN_POINT('Ctrl Pts',(8.9138218446291,-2.88991095673984,10.1010637458748));
#81927=CARTESIAN_POINT('Ctrl Pts',(8.93782988886079,-2.81478277312453,10.1024031171963));
#81928=CARTESIAN_POINT('Ctrl Pts',(8.98971475246432,-2.64505908544872,10.1054313643346));
#81929=CARTESIAN_POINT('Ctrl Pts',(9.01705245589767,-2.5503085773541,10.1071236446912));
#81930=CARTESIAN_POINT('Ctrl Pts',(9.15334005028203,-2.04832847139825,10.1160981001334));
#81931=CARTESIAN_POINT('Ctrl Pts',(9.23621199523202,-1.63452368460492,10.1235516805611));
#81932=CARTESIAN_POINT('Ctrl Pts',(9.30957423374593,-1.07424875450005,10.1334496880995));
#81933=CARTESIAN_POINT('Ctrl Pts',(9.32493571689913,-0.931534684471982,
10.1359516481559));
#81934=CARTESIAN_POINT('Ctrl Pts',(9.34154150826324,-0.734903384540886,
10.1393506899484));
#81935=CARTESIAN_POINT('Ctrl Pts',(9.34560786727666,-0.68124470198844,10.1402733026146));
#81936=CARTESIAN_POINT('Ctrl Pts',(9.35205860019965,-0.585142569214773,
10.1419151087129));
#81937=CARTESIAN_POINT('Ctrl Pts',(9.35461677888467,-0.542712454683558,
10.1426361282046));
#81938=CARTESIAN_POINT('Ctrl Pts',(9.36037542913204,-0.435003751700202,
10.1444574765857));
#81939=CARTESIAN_POINT('Ctrl Pts',(9.36318181358036,-0.369706360836267,
10.1455535170896));
#81940=CARTESIAN_POINT('Ctrl Pts',(9.36672434902895,-0.260709731672432,
10.1473730654771));
#81941=CARTESIAN_POINT('Ctrl Pts',(9.36783831417369,-0.217025162038524,
10.1480996381313));
#81942=CARTESIAN_POINT('Ctrl Pts',(9.371149455807,-0.0380594066177049,10.1510677295456));
#81943=CARTESIAN_POINT('Ctrl Pts',(9.37072208491539,0.0972541268768818,
10.1532921637666));
#81944=CARTESIAN_POINT('Ctrl Pts',(9.35817740144804,0.60265224564294,10.1615866244958));
#81945=CARTESIAN_POINT('Ctrl Pts',(9.32705958226323,0.971922420416597,10.1676325813907));
#81946=CARTESIAN_POINT('Ctrl Pts',(9.26057223576685,1.43263976702856,10.175418197495));
#81947=CARTESIAN_POINT('Ctrl Pts',(9.24553328644854,1.52668563535637,10.1770193723744));
#81948=CARTESIAN_POINT('Ctrl Pts',(9.21554614774134,1.69746973842361,10.179951533437));
#81949=CARTESIAN_POINT('Ctrl Pts',(9.20106621668669,1.77428147638907,10.1812793657297));
#81950=CARTESIAN_POINT('Ctrl Pts',(9.16586305781981,1.94898706400914,10.1843211279145));
#81951=CARTESIAN_POINT('Ctrl Pts',(9.14452940958802,2.0467481478695,10.1860388606589));
#81952=CARTESIAN_POINT('Ctrl Pts',(9.05795775111327,2.41504118320277,10.1925691210189));
#81953=CARTESIAN_POINT('Ctrl Pts',(8.98224569737743,2.68296173546328,10.1974453808365));
#81954=CARTESIAN_POINT('Ctrl Pts',(8.81287232303262,3.19414980005386,10.2069120801483));
#81955=CARTESIAN_POINT('Ctrl Pts',(8.72076503834788,3.43766913277399,10.2114956504665));
#81956=CARTESIAN_POINT('Ctrl Pts',(8.59356862578152,3.73580588414019,10.2170993937782));
#81957=CARTESIAN_POINT('Ctrl Pts',(8.56789565763895,3.79431566388508,10.218198551966));
#81958=CARTESIAN_POINT('Ctrl Pts',(8.52420453726292,3.89118459735888,10.2200147205667));
#81959=CARTESIAN_POINT('Ctrl Pts',(8.50652101932823,3.92969219266625,10.2207356334923));
#81960=CARTESIAN_POINT('Ctrl Pts',(8.46539933715897,4.01766034645509,10.2223797446501));
#81961=CARTESIAN_POINT('Ctrl Pts',(8.44178785323156,4.06703804463813,10.2233008597347));
#81962=CARTESIAN_POINT('Ctrl Pts',(8.34693818774827,4.26100799774475,10.2269173926668));
#81963=CARTESIAN_POINT('Ctrl Pts',(8.2724065346243,4.40395920592978,10.2295789707237));
#81964=CARTESIAN_POINT('Ctrl Pts',(8.03547639432324,4.83113066091047,10.237608762058));
#81965=CARTESIAN_POINT('Ctrl Pts',(7.8618418958453,5.10883024933997,10.2429413159281));
#81966=CARTESIAN_POINT('Ctrl Pts',(7.59802477075159,5.48535784760032,10.250565521944));
#81967=CARTESIAN_POINT('Ctrl Pts',(7.51972351230309,5.59221685002455,10.2527756127599));
#81968=CARTESIAN_POINT('Ctrl Pts',(7.39389292400272,5.75651638269419,10.2562559910987));
#81969=CARTESIAN_POINT('Ctrl Pts',(7.34789898012279,5.81511083178934,10.2575140718019));
#81970=CARTESIAN_POINT('Ctrl Pts',(7.25004745267303,5.93675502850652,10.2601627510037));
#81971=CARTESIAN_POINT('Ctrl Pts',(7.19805467209914,5.99968809478711,10.2615543830147));
#81972=CARTESIAN_POINT('Ctrl Pts',(7.06436046471031,6.15727445154968,10.2650944106049));
#81973=CARTESIAN_POINT('Ctrl Pts',(6.98157465898671,6.25098653039777,10.2672515303675));
#81974=CARTESIAN_POINT('Ctrl Pts',(6.83992665839876,6.40500441705825,10.2708836146243));
#81975=CARTESIAN_POINT('Ctrl Pts',(6.78208158589228,6.46622359704468,10.2723512136757));
#81976=CARTESIAN_POINT('Ctrl Pts',(6.51067300889796,6.74581455875415,10.2791614672836));
#81977=CARTESIAN_POINT('Ctrl Pts',(6.28733887298216,6.9544407703665,10.2845597209468));
#81978=CARTESIAN_POINT('Ctrl Pts',(5.96381700735658,7.2283123901585,10.2919687211966));
#81979=CARTESIAN_POINT('Ctrl Pts',(5.87197468072702,7.30311760674897,10.2940284546498));
#81980=CARTESIAN_POINT('Ctrl Pts',(5.73739892780726,7.40854888094058,10.2969715259456));
#81981=CARTESIAN_POINT('Ctrl Pts',(5.69578739033028,7.440587947122,10.2978714487297));
#81982=CARTESIAN_POINT('Ctrl Pts',(5.61980684758141,7.49807874036028,10.2994948408777));
#81983=CARTESIAN_POINT('Ctrl Pts',(5.58552886306757,7.52364812568489,10.3002198542422));
#81984=CARTESIAN_POINT('Ctrl Pts',(5.49652949781402,7.58909301991513,10.3020843812633));
#81985=CARTESIAN_POINT('Ctrl Pts',(5.44154875263911,7.62861170789344,10.3032191192111));
#81986=CARTESIAN_POINT('Ctrl Pts',(5.31451082038049,7.71785094881704,10.3058075571702));
#81987=CARTESIAN_POINT('Ctrl Pts',(5.24217542081502,7.76716456835253,10.3072572125868));
#81988=CARTESIAN_POINT('Ctrl Pts',(4.96814617483051,7.94840807426826,10.3126766369177));
#81989=CARTESIAN_POINT('Ctrl Pts',(4.76207819457341,8.07355429152338,10.3166095639365));
#81990=CARTESIAN_POINT('Ctrl Pts',(4.50298005476758,8.21753162763616,10.3214790341816));
#81991=CARTESIAN_POINT('Ctrl Pts',(4.45430718417808,8.24401618924771,10.3223904804223));
#81992=CARTESIAN_POINT('Ctrl Pts',(4.36738060196495,8.29032132115237,10.3240136632783));
#81993=CARTESIAN_POINT('Ctrl Pts',(4.32922113029058,8.31031197093883,10.3247246573602));
#81994=CARTESIAN_POINT('Ctrl Pts',(4.29092662690317,8.33003803983111,10.3254369059772));
#81995=CARTESIAN_POINT('Origin',(0.,0.,2.15141010809499));
#81996=CARTESIAN_POINT('',(4.29092665208775,8.33003802685816,11.5229686882669));
#81997=CARTESIAN_POINT('',(4.29126566285743,8.33069681713359,11.3257065478457));
#81998=CARTESIAN_POINT('',(4.29092662815669,8.33003803918541,2.15141010809499));
#81999=CARTESIAN_POINT('',(-9.3705222398215,0.000212818811248933,10.848589891905));
#82000=CARTESIAN_POINT('Ctrl Pts',(4.29092665208775,8.33003802685817,11.5229686882669));
#82001=CARTESIAN_POINT('Ctrl Pts',(4.41956745097948,8.26377323542136,11.520593532693));
#82002=CARTESIAN_POINT('Ctrl Pts',(4.54667758961367,8.19452631572227,11.5182115257494));
#82003=CARTESIAN_POINT('Ctrl Pts',(4.79074666401042,8.05413244729533,11.5135455764697));
#82004=CARTESIAN_POINT('Ctrl Pts',(4.90783147706481,7.98332594377128,11.5112643737165));
#82005=CARTESIAN_POINT('Ctrl Pts',(5.09369302732341,7.8652924519121,11.5075630917925));
#82006=CARTESIAN_POINT('Ctrl Pts',(5.16346283178717,7.8196665885812,11.5061550238087));
#82007=CARTESIAN_POINT('Ctrl Pts',(5.3011925865166,7.72695129776469,11.5033363700435));
#82008=CARTESIAN_POINT('Ctrl Pts',(5.36915669174465,7.67988122162119,11.5019260264738));
#82009=CARTESIAN_POINT('Ctrl Pts',(5.54411586436051,7.5552515284045,11.4982436699576));
#82010=CARTESIAN_POINT('Ctrl Pts',(5.65010874439515,7.47631710174249,11.4959613451287));
#82011=CARTESIAN_POINT('Ctrl Pts',(5.89233053951926,7.28783723043592,11.490627464591));
#82012=CARTESIAN_POINT('Ctrl Pts',(6.0272343899226,7.17666886986867,11.487566013402));
#82013=CARTESIAN_POINT('Ctrl Pts',(6.22268468063554,7.00620670604878,11.4830100673927));
#82014=CARTESIAN_POINT('Ctrl Pts',(6.2856640753546,6.94976000813127,11.4815226882742));
#82015=CARTESIAN_POINT('Ctrl Pts',(6.44779136540077,6.80044295749968,11.477648220966));
#82016=CARTESIAN_POINT('Ctrl Pts',(6.54569916649103,6.70625531905782,11.4752626692437));
#82017=CARTESIAN_POINT('Ctrl Pts',(6.71814143510164,6.53298990960608,11.4709973305568));
#82018=CARTESIAN_POINT('Ctrl Pts',(6.79341414591935,6.45468092517459,11.4691124029034));
#82019=CARTESIAN_POINT('Ctrl Pts',(6.90074705988993,6.3390607087022,11.4664009833136));
#82020=CARTESIAN_POINT('Ctrl Pts',(6.93390164910408,6.30277784693286,11.4655600580448));
#82021=CARTESIAN_POINT('Ctrl Pts',(6.99616820966099,6.23355019936897,11.4639756940377));
#82022=CARTESIAN_POINT('Ctrl Pts',(7.02533672241702,6.20065816188936,11.4632314877448));
#82023=CARTESIAN_POINT('Ctrl Pts',(7.10440876173399,6.11021793265991,11.4612068228262));
#82024=CARTESIAN_POINT('Ctrl Pts',(7.15384384563408,6.05226447818558,11.4599329441222));
#82025=CARTESIAN_POINT('Ctrl Pts',(7.23749526199406,5.95174168749394,11.4577575676415));
#82026=CARTESIAN_POINT('Ctrl Pts',(7.27205609996119,5.90946417809317,11.4568528002402));
#82027=CARTESIAN_POINT('Ctrl Pts',(7.42771419027369,5.7156175570998,11.45274501019));
#82028=CARTESIAN_POINT('Ctrl Pts',(7.54445596275977,5.56061207042768,11.4495712522038));
#82029=CARTESIAN_POINT('Ctrl Pts',(7.7448806877038,5.27655332609422,11.4438717521632));
#82030=CARTESIAN_POINT('Ctrl Pts',(7.83035820075265,5.14885251612277,11.4413496440123));
#82031=CARTESIAN_POINT('Ctrl Pts',(7.99712577256745,4.88594233667946,11.4362056494782));
#82032=CARTESIAN_POINT('Ctrl Pts',(8.07821927640738,4.7506658748682,11.4335836670146));
#82033=CARTESIAN_POINT('Ctrl Pts',(8.1983822181979,4.53823459202642,11.4294874255465));
#82034=CARTESIAN_POINT('Ctrl Pts',(8.23986295004745,4.46247719652791,11.4280307771367));
#82035=CARTESIAN_POINT('Ctrl Pts',(8.31807038809955,4.31483536528738,11.4251980787988));
#82036=CARTESIAN_POINT('Ctrl Pts',(8.3549272510876,4.24302837651527,11.4238231214834));
#82037=CARTESIAN_POINT('Ctrl Pts',(8.44358182885378,4.06467037068358,11.4204138706668));
#82038=CARTESIAN_POINT('Ctrl Pts',(8.49429522482729,3.95759622105893,11.4183722483068));
#82039=CARTESIAN_POINT('Ctrl Pts',(8.60448467211024,3.71306507309902,11.4137225784626));
#82040=CARTESIAN_POINT('Ctrl Pts',(8.66272303336974,3.57508576030736,11.411107819149));
#82041=CARTESIAN_POINT('Ctrl Pts',(8.80487176216494,3.21440975469719,11.4043110814434));
#82042=CARTESIAN_POINT('Ctrl Pts',(8.88365088034356,2.98980664153678,11.400113946015));
#82043=CARTESIAN_POINT('Ctrl Pts',(8.99224547400813,2.63782414370871,11.3936676029783));
#82044=CARTESIAN_POINT('Ctrl Pts',(9.02808914705693,2.51240947766224,11.3913964020703));
#82045=CARTESIAN_POINT('Ctrl Pts',(9.07499655340303,2.33429084753194,11.3882237482713));
#82046=CARTESIAN_POINT('Ctrl Pts',(9.08824200729681,2.28217734621896,11.3873018729595));
#82047=CARTESIAN_POINT('Ctrl Pts',(9.11115567449772,2.18866049084321,11.3856606905596));
#82048=CARTESIAN_POINT('Ctrl Pts',(9.12099199704146,2.14730003942896,11.3849395664472));
#82049=CARTESIAN_POINT('Ctrl Pts',(9.14525037058485,2.04212175727382,11.3831169446179));
#82050=CARTESIAN_POINT('Ctrl Pts',(9.15928613498678,1.97821716170038,11.3820197497822));
#82051=CARTESIAN_POINT('Ctrl Pts',(9.21488352024748,1.71179607794913,11.3774789058821));
#82052=CARTESIAN_POINT('Ctrl Pts',(9.25040667040158,1.50807859038459,11.3740855975635));
#82053=CARTESIAN_POINT('Ctrl Pts',(9.32482095701645,0.978289381433982,11.3653145179413));
#82054=CARTESIAN_POINT('Ctrl Pts',(9.35336664289584,0.651051407220187,11.3599427391217));
#82055=CARTESIAN_POINT('Ctrl Pts',(9.36813634946008,0.222826483443642,11.3527871234167));
#82056=CARTESIAN_POINT('Ctrl Pts',(9.36998381588262,0.122611295240142,11.3511043556485));
#82057=CARTESIAN_POINT('Ctrl Pts',(9.37041177136695,-0.0565206334172836,
11.3480784729755));
#82058=CARTESIAN_POINT('Ctrl Pts',(9.36960356803008,-0.135426331802459,
11.3467393890732));
#82059=CARTESIAN_POINT('Ctrl Pts',(9.36561540221525,-0.30975294512381,11.3437661793526));
#82060=CARTESIAN_POINT('Ctrl Pts',(9.3619735382191,-0.405154489659079,11.3421292614089));
#82061=CARTESIAN_POINT('Ctrl Pts',(9.34302093234984,-0.759486130723608,
11.3360129447384));
#82062=CARTESIAN_POINT('Ctrl Pts',(9.31841938269814,-1.01780086647856,11.331477924072));
#82063=CARTESIAN_POINT('Ctrl Pts',(9.24218551477918,-1.57295549186521,11.3216332951951));
#82064=CARTESIAN_POINT('Ctrl Pts',(9.18689308391084,-1.86900451967697,11.3163205799458));
#82065=CARTESIAN_POINT('Ctrl Pts',(9.10500382251618,-2.21436219384678,11.3101929599984));
#82066=CARTESIAN_POINT('Ctrl Pts',(9.09210607575656,-2.26673810961586,11.3092657843955));
#82067=CARTESIAN_POINT('Ctrl Pts',(9.06824678374012,-2.36014592674293,11.3076177528998));
#82068=CARTESIAN_POINT('Ctrl Pts',(9.05745717183549,-2.40122013266702,11.306895066372));
#82069=CARTESIAN_POINT('Ctrl Pts',(9.03229942467694,-2.49440861672463,11.3052604307046));
#82070=CARTESIAN_POINT('Ctrl Pts',(9.01775882031005,-2.5464746456243,11.304350419329));
#82071=CARTESIAN_POINT('Ctrl Pts',(8.96043308002719,-2.74509225004799,11.3008868630333));
#82072=CARTESIAN_POINT('Ctrl Pts',(8.91451913581543,-2.89071639504993,11.2983635816078));
#82073=CARTESIAN_POINT('Ctrl Pts',(8.7325342431694,-3.4222572814741,11.2891220299348));
#82074=CARTESIAN_POINT('Ctrl Pts',(8.5747884665114,-3.80026347487041,11.2824686121042));
#82075=CARTESIAN_POINT('Ctrl Pts',(8.34856989435705,-4.25592271021784,11.2739712717521));
#82076=CARTESIAN_POINT('Ctrl Pts',(8.30287903862549,-4.34438683858014,11.2722993850308));
#82077=CARTESIAN_POINT('Ctrl Pts',(8.21847405207963,-4.50160997968997,11.2692846791357));
#82078=CARTESIAN_POINT('Ctrl Pts',(8.18028472012145,-4.57064000093292,11.2679457589937));
#82079=CARTESIAN_POINT('Ctrl Pts',(8.09368341799795,-4.72261536244842,11.2649628543155));
#82080=CARTESIAN_POINT('Ctrl Pts',(8.0448587383063,-4.80531528140412,11.2633159665235));
#82081=CARTESIAN_POINT('Ctrl Pts',(7.85070507319806,-5.1229201154839,11.2568984069792));
#82082=CARTESIAN_POINT('Ctrl Pts',(7.69628890173883,-5.35210394959635,11.252063319376));
#82083=CARTESIAN_POINT('Ctrl Pts',(7.36461346989674,-5.80027634665401,11.2422639406318));
#82084=CARTESIAN_POINT('Ctrl Pts',(7.1871509706775,-6.01877052242378,11.2373040598758));
#82085=CARTESIAN_POINT('Ctrl Pts',(6.96395562108168,-6.26959871158336,11.2315064998035));
#82086=CARTESIAN_POINT('Ctrl Pts',(6.92743032477523,-6.3099330431662,11.2305710187155));
#82087=CARTESIAN_POINT('Ctrl Pts',(6.86173280590428,-6.38122378245983,11.2289135456529));
#82088=CARTESIAN_POINT('Ctrl Pts',(6.8326972498147,-6.41230398323212,11.2281896432418));
#82089=CARTESIAN_POINT('Ctrl Pts',(6.76655410739108,-6.48214546462628,11.2265604414798));
#82090=CARTESIAN_POINT('Ctrl Pts',(6.72932323347633,-6.52078777064284,11.2256569932477));
#82091=CARTESIAN_POINT('Ctrl Pts',(6.58811985198719,-6.66484691055137,11.2222766763406));
#82092=CARTESIAN_POINT('Ctrl Pts',(6.48198528521763,-6.76811454724948,11.2198282182329));
#82093=CARTESIAN_POINT('Ctrl Pts',(6.24282807631506,-6.99002386893736,11.2144596525456));
#82094=CARTESIAN_POINT('Ctrl Pts',(6.10877730509157,-7.10747325032063,11.2115457586906));
#82095=CARTESIAN_POINT('Ctrl Pts',(5.78325070996419,-7.37666879835267,11.2046152544383));
#82096=CARTESIAN_POINT('Ctrl Pts',(5.58902957218264,-7.5248906488868,11.2005913816635));
#82097=CARTESIAN_POINT('Ctrl Pts',(5.31006543084032,-7.72102050088655,11.1948906137783));
#82098=CARTESIAN_POINT('Ctrl Pts',(5.23003243792723,-7.77545581266769,11.1932641087567));
#82099=CARTESIAN_POINT('Ctrl Pts',(5.08327708936292,-7.87198192700135,11.1902948312084));
#82100=CARTESIAN_POINT('Ctrl Pts',(5.01683903818444,-7.91448870475178,11.188955405277));
#82101=CARTESIAN_POINT('Ctrl Pts',(4.86604866299914,-8.00830203948611,11.1859251403872));
#82102=CARTESIAN_POINT('Ctrl Pts',(4.78140616886971,-8.05912440221307,11.184230875049));
#82103=CARTESIAN_POINT('Ctrl Pts',(4.59952608815703,-8.16445758318166,11.1806044186245));
#82104=CARTESIAN_POINT('Ctrl Pts',(4.50208681872962,-8.21859002871254,11.1786699918157));
#82105=CARTESIAN_POINT('Ctrl Pts',(4.20036041618973,-8.37923792720377,11.1727101113469));
#82106=CARTESIAN_POINT('Ctrl Pts',(3.99309236801689,-8.47996868092159,11.1686558996977));
#82107=CARTESIAN_POINT('Ctrl Pts',(3.75691725811887,-8.58416733975753,11.1641189104818));
#82108=CARTESIAN_POINT('Ctrl Pts',(3.73146099534917,-8.59526352370031,11.1636309757074));
#82109=CARTESIAN_POINT('Ctrl Pts',(3.53274050550957,-8.68083501623256,11.1598311223301));
#82110=CARTESIAN_POINT('Ctrl Pts',(3.3573124198528,-8.75017746713286,11.1565297031563));
#82111=CARTESIAN_POINT('Ctrl Pts',(3.12733545232831,-8.83314677988633,11.1523138361618));
#82112=CARTESIAN_POINT('Ctrl Pts',(3.07459083549419,-8.85164393093529,11.1513545256751));
#82113=CARTESIAN_POINT('Ctrl Pts',(2.98175121337683,-8.88327217007262,11.1496811296333));
#82114=CARTESIAN_POINT('Ctrl Pts',(2.94172734329044,-8.89660637489602,11.148964774093));
#82115=CARTESIAN_POINT('Ctrl Pts',(2.84366959299135,-8.92854086865132,11.1472216771474));
#82116=CARTESIAN_POINT('Ctrl Pts',(2.78554178894041,-8.94684613501642,11.1461983166975));
#82117=CARTESIAN_POINT('Ctrl Pts',(2.50732838193869,-9.03148527318126,11.1413391922819));
#82118=CARTESIAN_POINT('Ctrl Pts',(2.28502919967817,-9.09027304966173,11.13757045591));
#82119=CARTESIAN_POINT('Ctrl Pts',(1.75800011902292,-9.20909139405502,11.1287147046982));
#82120=CARTESIAN_POINT('Ctrl Pts',(1.45200243512864,-9.26226846554898,11.1236300890653));
#82121=CARTESIAN_POINT('Ctrl Pts',(1.04403483791344,-9.31244902217868,11.1167685895778));
#82122=CARTESIAN_POINT('Ctrl Pts',(0.943946140021,-9.32312614703433,11.1150794346931));
#82123=CARTESIAN_POINT('Ctrl Pts',(0.765017581838083,-9.3393027303344,11.1120459368315));
#82124=CARTESIAN_POINT('Ctrl Pts',(0.68624340031113,-9.34542119709954,11.1107056897563));
#82125=CARTESIAN_POINT('Ctrl Pts',(0.513811422372697,-9.35662219639776,
11.107760560202));
#82126=CARTESIAN_POINT('Ctrl Pts',(0.4201356265172,-9.36129622988581,11.1061532186484));
#82127=CARTESIAN_POINT('Ctrl Pts',(0.0977176434978746,-9.37253423872393,
11.1005954177021));
#82128=CARTESIAN_POINT('Ctrl Pts',(-0.131184775563268,-9.37212551621604,
11.0966034596699));
#82129=CARTESIAN_POINT('Ctrl Pts',(-0.600847890812155,-9.35407594509233,
11.0883564337875));
#82130=CARTESIAN_POINT('Ctrl Pts',(-0.841406803379838,-9.33551228055605,
11.0841017271851));
#82131=CARTESIAN_POINT('Ctrl Pts',(-1.19395801001081,-9.29456751719272,
11.0779013244183));
#82132=CARTESIAN_POINT('Ctrl Pts',(-1.3066871768029,-9.27939059390266,11.0759245243684));
#82133=CARTESIAN_POINT('Ctrl Pts',(-1.47050124401979,-9.25429165176958,
11.0730722028225));
#82134=CARTESIAN_POINT('Ctrl Pts',(-1.52182389823631,-9.24599047823566,
11.0721815138153));
#82135=CARTESIAN_POINT('Ctrl Pts',(-1.61536118648213,-9.23006139141782,
11.070565168352));
#82136=CARTESIAN_POINT('Ctrl Pts',(-1.65759747059468,-9.22256990624319,
11.0698380847778));
#82137=CARTESIAN_POINT('Ctrl Pts',(-1.76741941471712,-9.20231190062029,
11.0679536289174));
#82138=CARTESIAN_POINT('Ctrl Pts',(-1.83491865618041,-9.18909077451248,
11.0668012560411));
#82139=CARTESIAN_POINT('Ctrl Pts',(-1.98994013058943,-9.15695039037478,
11.0641624796589));
#82140=CARTESIAN_POINT('Ctrl Pts',(-2.07734904930345,-9.13751734068116,
11.0626803475791));
#82141=CARTESIAN_POINT('Ctrl Pts',(-2.41173922755492,-9.05812835902748,
11.0570132250866));
#82142=CARTESIAN_POINT('Ctrl Pts',(-2.65652176010058,-8.98938640445197,
11.0528680142331));
#82143=CARTESIAN_POINT('Ctrl Pts',(-3.09066409352482,-8.8481827887134,11.0453617406064));
#82144=CARTESIAN_POINT('Ctrl Pts',(-3.28104253042078,-8.77936801606186,
11.0420155841091));
#82145=CARTESIAN_POINT('Ctrl Pts',(-3.55643267666661,-8.66961485324422,
11.0370552617146));
#82146=CARTESIAN_POINT('Ctrl Pts',(-3.64329313475421,-8.63347265979584,
11.0354730491027));
#82147=CARTESIAN_POINT('Ctrl Pts',(-3.80205441782347,-8.56459024628363,
11.0325457510767));
#82148=CARTESIAN_POINT('Ctrl Pts',(-3.8741138293466,-8.53223686299977,11.0312034651188));
#82149=CARTESIAN_POINT('Ctrl Pts',(-4.03827770859339,-8.45602174037447,
11.028113161768));
#82150=CARTESIAN_POINT('Ctrl Pts',(-4.1300921798462,-8.41155925146307,11.0263610846436));
#82151=CARTESIAN_POINT('Ctrl Pts',(-4.27617910585212,-8.33784593483541,
11.0235351781345));
#82152=CARTESIAN_POINT('Ctrl Pts',(-4.33092075136979,-8.3095431890033,11.0224675244031));
#82153=CARTESIAN_POINT('Ctrl Pts',(-4.5368013356058,-8.20051084294139,11.0184197966665));
#82154=CARTESIAN_POINT('Ctrl Pts',(-4.68599511580999,-8.11618099861006,
11.015419461597));
#82155=CARTESIAN_POINT('Ctrl Pts',(-5.09890024896231,-7.86760944597705,
11.0069544059769));
#82156=CARTESIAN_POINT('Ctrl Pts',(-5.35687832412414,-7.69427820438116,
11.0014689889127));
#82157=CARTESIAN_POINT('Ctrl Pts',(-5.64855046442738,-7.47651742973718,
10.995186281113));
#82158=CARTESIAN_POINT('Ctrl Pts',(-5.69105616193072,-7.44421352491204,
10.9942687869764));
#82159=CARTESIAN_POINT('Ctrl Pts',(-5.7668182963076,-7.38560690305223,10.9926316623988));
#82160=CARTESIAN_POINT('Ctrl Pts',(-5.80017661920584,-7.35943841559748,
10.9919102948555));
#82161=CARTESIAN_POINT('Ctrl Pts',(-5.8350227041693,-7.33171873697793,10.9911563566436));
#82162=CARTESIAN_POINT('Ctrl Pts',(-5.83668859953585,-7.33039260806499,
10.9911203115629));
#82163=CARTESIAN_POINT('Ctrl Pts',(-5.83932710802561,-7.32829076495229,
10.9910632196975));
#82164=CARTESIAN_POINT('Ctrl Pts',(-5.84030001886517,-7.32751542474334,
10.991042167425));
#82165=CARTESIAN_POINT('Ctrl Pts',(-5.84278858338152,-7.32553140669771,
10.9909883174671));
#82166=CARTESIAN_POINT('Ctrl Pts',(-5.84430401647933,-7.3243224521844,10.9909555238261));
#82167=CARTESIAN_POINT('Ctrl Pts',(-5.84722781351326,-7.32198847366916,
10.9908922509943));
#82168=CARTESIAN_POINT('Ctrl Pts',(-5.84863622818902,-7.32086351341033,
10.9908617708811));
#82169=CARTESIAN_POINT('Ctrl Pts',(-5.85136808453669,-7.31868017291583,
10.9908026473251));
#82170=CARTESIAN_POINT('Ctrl Pts',(-5.85269156388538,-7.31762183992801,
10.9907740032027));
#82171=CARTESIAN_POINT('Ctrl Pts',(-5.85527085484812,-7.31555813774285,
10.990718177404));
#82172=CARTESIAN_POINT('Ctrl Pts',(-5.8565266947959,-7.31455280406621,10.9906909952205));
#82173=CARTESIAN_POINT('Ctrl Pts',(-5.85898460764888,-7.31258413987955,
10.9906377926643));
#82174=CARTESIAN_POINT('Ctrl Pts',(-5.8601867020153,-7.31162083624473,10.9906117719101));
#82175=CARTESIAN_POINT('Ctrl Pts',(-5.86254855687697,-7.30972719677886,
10.9905606449096));
#82176=CARTESIAN_POINT('Ctrl Pts',(-5.86370833358325,-7.30879688127502,
10.9905355383772));
#82177=CARTESIAN_POINT('Ctrl Pts',(-5.86599517222388,-7.30696159776288,
10.9904860317233));
#82178=CARTESIAN_POINT('Ctrl Pts',(-5.86712224628781,-7.30605664492484,
10.990461631389));
#82179=CARTESIAN_POINT('Ctrl Pts',(-5.86935195390955,-7.30426551439291,
10.9904133580948));
#82180=CARTESIAN_POINT('Ctrl Pts',(-5.8704545962716,-7.30337934772153,10.9903894849814));
#82181=CARTESIAN_POINT('Ctrl Pts',(-5.87264271588078,-7.30161999386635,
10.9903421086721));
#82182=CARTESIAN_POINT('Ctrl Pts',(-5.87372819915641,-7.3007468142411,10.9903186053719));
#82183=CARTESIAN_POINT('Ctrl Pts',(-5.87588853919116,-7.29900820946103,
10.9902718271435));
#82184=CARTESIAN_POINT('Ctrl Pts',(-5.876963399581,-7.29814278887192,10.9902485521529));
#82185=CARTESIAN_POINT('Ctrl Pts',(-5.87910849967673,-7.29641488683421,
10.9902021004964));
#82186=CARTESIAN_POINT('Ctrl Pts',(-5.88017874085686,-7.29555240727954,
10.9901789238053));
#82187=CARTESIAN_POINT('Ctrl Pts',(-5.88232023900376,-7.2938258522208,10.9901325466618));
#82188=CARTESIAN_POINT('Ctrl Pts',(-5.8833914954546,-7.29296177611884,10.9901093462182));
#82189=CARTESIAN_POINT('Ctrl Pts',(-5.88554042640442,-7.29122766548963,
10.9900628045193));
#82190=CARTESIAN_POINT('Ctrl Pts',(-5.8866180984459,-7.29035762798312,10.9900394633056));
#82191=CARTESIAN_POINT('Ctrl Pts',(-5.88878514402303,-7.2886073122139,10.9899925255518));
#82192=CARTESIAN_POINT('Ctrl Pts',(-5.88987451318281,-7.28772702857922,
10.9899689290853));
#82193=CARTESIAN_POINT('Ctrl Pts',(-5.8920702199633,-7.28595193575882,10.9899213666281));
#82194=CARTESIAN_POINT('Ctrl Pts',(-5.8931765512165,-7.28505711874372,10.9898974007439));
#82195=CARTESIAN_POINT('Ctrl Pts',(-5.89541152672902,-7.28324859535273,
10.98984898353));
#82196=CARTESIAN_POINT('Ctrl Pts',(-5.89654016249166,-7.28233487854823,
10.9898245323415));
#82197=CARTESIAN_POINT('Ctrl Pts',(-5.89882525879532,-7.28048403914862,
10.9897750249269));
#82198=CARTESIAN_POINT('Ctrl Pts',(-5.89998170854144,-7.2795469032747,10.9897499688789));
#82199=CARTESIAN_POINT('Ctrl Pts',(-5.90232820048541,-7.27764448322589,
10.9896991265545));
#82200=CARTESIAN_POINT('Ctrl Pts',(-5.90351822930849,-7.27667918261458,
10.9896733404973));
#82201=CARTESIAN_POINT('Ctrl Pts',(-5.90593799330101,-7.27471538900458,
10.9896209053994));
#82202=CARTESIAN_POINT('Ctrl Pts',(-5.90716771216731,-7.27371687599022,
10.9895942566238));
#82203=CARTESIAN_POINT('Ctrl Pts',(-5.90967341098587,-7.27168123213273,
10.9895399537077));
#82204=CARTESIAN_POINT('Ctrl Pts',(-5.91094937126689,-7.2706440771492,10.9895122998847));
#82205=CARTESIAN_POINT('Ctrl Pts',(-5.91355464990306,-7.26852525634999,
10.9894558326538));
#82206=CARTESIAN_POINT('Ctrl Pts',(-5.91488394465064,-7.26744356159045,
10.9894270196241));
#82207=CARTESIAN_POINT('Ctrl Pts',(-5.91760364206364,-7.2652292058871,10.9893680655056));
#82208=CARTESIAN_POINT('Ctrl Pts',(-5.91899401646741,-7.26409651034892,
10.989337924866));
#82209=CARTESIAN_POINT('Ctrl Pts',(-5.92184439811943,-7.26177302981517,
10.9892761301267));
#82210=CARTESIAN_POINT('Ctrl Pts',(-5.92330437158937,-7.26058220348756,
10.9892444765593));
#82211=CARTESIAN_POINT('Ctrl Pts',(-5.92630338806166,-7.25813455120618,
10.9891794506432));
#82212=CARTESIAN_POINT('Ctrl Pts',(-5.92784239064463,-7.25687767586319,
10.9891460789259));
#82213=CARTESIAN_POINT('Ctrl Pts',(-5.93100996751195,-7.25428909359632,
10.9890773880983));
#82214=CARTESIAN_POINT('Ctrl Pts',(-5.93263849335326,-7.25295732755823,
10.9890420697376));
#82215=CARTESIAN_POINT('Ctrl Pts',(-5.9359968582298,-7.25020905632485,10.9889692299022));
#82216=CARTESIAN_POINT('Ctrl Pts',(-5.93772663907653,-7.24879248019496,
10.9889317093189));
#82217=CARTESIAN_POINT('Ctrl Pts',(-5.98494343423164,-7.21009680594858,
10.9879074417202));
#82218=CARTESIAN_POINT('Ctrl Pts',(-6.03007904898525,-7.1723908526717,10.9869260154301));
#82219=CARTESIAN_POINT('Ctrl Pts',(-6.15938598691588,-7.06228540998663,
10.9841033016293));
#82220=CARTESIAN_POINT('Ctrl Pts',(-6.24262948299761,-6.9888116417459,10.9822722821226));
#82221=CARTESIAN_POINT('Ctrl Pts',(-6.62404769718664,-6.63990493115117,
10.9737743527757));
#82222=CARTESIAN_POINT('Ctrl Pts',(-6.90542848173967,-6.34676320576499,
10.9671691391112));
#82223=CARTESIAN_POINT('Ctrl Pts',(-7.22965082951393,-5.96181335335713,
10.9587569783418));
#82224=CARTESIAN_POINT('Ctrl Pts',(-7.29122314183169,-5.88635155368662,
10.957120612771));
#82225=CARTESIAN_POINT('Ctrl Pts',(-7.39653820379273,-5.75309122269123,
10.9542498059002));
#82226=CARTESIAN_POINT('Ctrl Pts',(-7.44080749616265,-5.69571942741086,
10.9530197989552));
#82227=CARTESIAN_POINT('Ctrl Pts',(-7.53862946217726,-5.56585774482449,
10.9502480853874));
#82228=CARTESIAN_POINT('Ctrl Pts',(-7.59181075722689,-5.49309712100544,
10.9487035799898));
#82229=CARTESIAN_POINT('Ctrl Pts',(-7.76784447735452,-5.24481405172247,
10.9434612820827));
#82230=CARTESIAN_POINT('Ctrl Pts',(-7.88572431280793,-5.0658497587383,10.9397275930791));
#82231=CARTESIAN_POINT('Ctrl Pts',(-8.18079569777134,-4.58258287090693,
10.9297996673474));
#82232=CARTESIAN_POINT('Ctrl Pts',(-8.34715161977635,-4.27206551216097,
10.9235675773498));
#82233=CARTESIAN_POINT('Ctrl Pts',(-8.5185670040455,-3.90365907013084,10.9165515102537));
#82234=CARTESIAN_POINT('Ctrl Pts',(-8.54106201876819,-3.8541922042012,10.9156173113304));
#82235=CARTESIAN_POINT('Ctrl Pts',(-8.58013100758253,-3.76625691576903,
10.9139722220597));
#82236=CARTESIAN_POINT('Ctrl Pts',(-8.59687971231175,-3.72786782140688,
10.9132593310904));
#82237=CARTESIAN_POINT('Ctrl Pts',(-8.62288713202287,-3.66714967919227,
10.9121404383629));
#82238=CARTESIAN_POINT('Ctrl Pts',(-8.63231772131513,-3.64489506312267,
10.9117321071465));
#82239=CARTESIAN_POINT('Ctrl Pts',(-8.64642644225138,-3.61123894377407,
10.9111170769088));
#82240=CARTESIAN_POINT('Ctrl Pts',(-8.65116835627592,-3.59986430325827,
10.9109096466553));
#82241=CARTESIAN_POINT('Ctrl Pts',(-8.6609540451265,-3.57625993122506,10.9104800518261));
#82242=CARTESIAN_POINT('Ctrl Pts',(-8.66599438844497,-3.56402880560234,
10.9102579249601));
#82243=CARTESIAN_POINT('Ctrl Pts',(-8.67837828280957,-3.53379589583153,
10.9097100049437));
#82244=CARTESIAN_POINT('Ctrl Pts',(-8.68569174295965,-3.51578184760399,
10.9093845213264));
#82245=CARTESIAN_POINT('Ctrl Pts',(-8.72055402322892,-3.42913859213306,
10.9078235073762));
#82246=CARTESIAN_POINT('Ctrl Pts',(-8.74734584718554,-3.36020752593731,
10.9065950763379));
#82247=CARTESIAN_POINT('Ctrl Pts',(-8.83265925331908,-3.13277229428126,
10.9025764115461));
#82248=CARTESIAN_POINT('Ctrl Pts',(-8.88771016492782,-2.9730018386727,10.8998074235589));
#82249=CARTESIAN_POINT('Ctrl Pts',(-9.02968001927931,-2.52169973952233,
10.8920529674702));
#82250=CARTESIAN_POINT('Ctrl Pts',(-9.10676862325481,-2.22729780275952,
10.8870663932108));
#82251=CARTESIAN_POINT('Ctrl Pts',(-9.18996168082823,-1.83198121796618,
10.8803192193218));
#82252=CARTESIAN_POINT('Ctrl Pts',(-9.20895754288809,-1.73396995010261,
10.8786429454963));
#82253=CARTESIAN_POINT('Ctrl Pts',(-9.24015543529145,-1.55799129262525,
10.8756237450521));
#82254=CARTESIAN_POINT('Ctrl Pts',(-9.25294555037285,-1.48013781267209,
10.874284770683));
#82255=CARTESIAN_POINT('Ctrl Pts',(-9.27598441316437,-1.32790585972024,
10.8716593122357));
#82256=CARTESIAN_POINT('Ctrl Pts',(-9.28632542938372,-1.25354728533169,
10.8703735259577));
#82257=CARTESIAN_POINT('Ctrl Pts',(-9.30795068350567,-1.0830544509598,10.8674175790309));
#82258=CARTESIAN_POINT('Ctrl Pts',(-9.31864115091131,-0.986853542837705,
10.8657439699172));
#82259=CARTESIAN_POINT('Ctrl Pts',(-9.3561038556868,-0.594439909765311,
10.8588966555578));
#82260=CARTESIAN_POINT('Ctrl Pts',(-9.37025666368476,-0.29719841436659,
10.8536567989704));
#82261=CARTESIAN_POINT('Ctrl Pts',(-9.37024999764631,0.000210022444156327,
10.8484327663521));
#82262=CARTESIAN_POINT('Ctrl Pts',(4.29126860009441,8.33070247396408,10.522886232912));
#82263=CARTESIAN_POINT('Ctrl Pts',(2.96799777839083,9.01176106266219,10.5481706725962));
#82264=CARTESIAN_POINT('Ctrl Pts',(-0.0657392449123033,9.74679514529692,
10.599700716706));
#82265=CARTESIAN_POINT('Ctrl Pts',(-4.64250383747633,8.58644271179361,10.6774763652415));
#82266=CARTESIAN_POINT('Ctrl Pts',(-8.16258095402662,5.35276680725565,10.7562131785184));
#82267=CARTESIAN_POINT('Ctrl Pts',(-9.29464270735565,2.08042600373183,10.8132510207396));
#82268=CARTESIAN_POINT('Ctrl Pts',(-9.37078403118896,0.267868275173487,
10.8440432585352));
#82269=CARTESIAN_POINT('Ctrl Pts',(-9.3705222398215,0.000212818811248933,
10.848589891905));
#82270=CARTESIAN_POINT('',(-9.36953762859325,3.21162273520589E-5,10.6513777224354));
#82271=CARTESIAN_POINT('Ctrl Pts',(4.29092662690317,8.33003803983112,10.3254369059772));
#82272=CARTESIAN_POINT('Ctrl Pts',(4.17084852669809,8.39189205718544,10.3276702672494));
#82273=CARTESIAN_POINT('Ctrl Pts',(4.04944275948985,8.45114463703808,10.3299162156179));
#82274=CARTESIAN_POINT('Ctrl Pts',(3.84522640799292,8.54540166368771,10.3336854708738));
#82275=CARTESIAN_POINT('Ctrl Pts',(3.76312163318825,8.58187457660759,10.3351985495077));
#82276=CARTESIAN_POINT('Ctrl Pts',(3.60732266131618,8.64841840941565,10.3380675133813));
#82277=CARTESIAN_POINT('Ctrl Pts',(3.53374498682596,8.67874208054923,10.3394214930332));
#82278=CARTESIAN_POINT('Ctrl Pts',(3.3583172671846,8.7484405633889,10.342648426147));
#82279=CARTESIAN_POINT('Ctrl Pts',(3.25614771850194,8.78697952131914,10.3445268344419));
#82280=CARTESIAN_POINT('Ctrl Pts',(2.90463136731083,8.91260067885413,10.3509851546152));
#82281=CARTESIAN_POINT('Ctrl Pts',(2.65228898312657,8.99092300707285,10.3556173114874));
#82282=CARTESIAN_POINT('Ctrl Pts',(2.15139289303251,9.12346580228876,10.3647264880036));
#82283=CARTESIAN_POINT('Ctrl Pts',(1.90326719737982,9.17843635979939,10.3691984159237));
#82284=CARTESIAN_POINT('Ctrl Pts',(1.59143747703267,9.23433001889079,10.3746733536811));
#82285=CARTESIAN_POINT('Ctrl Pts',(1.52955015718988,9.24478233837405,10.3757527078762));
#82286=CARTESIAN_POINT('Ctrl Pts',(1.42579690258112,9.26123514859852,10.3775476421041));
#82287=CARTESIAN_POINT('Ctrl Pts',(1.38398706489976,9.26757536280537,10.3782668954658));
#82288=CARTESIAN_POINT('Ctrl Pts',(1.28719448313514,9.28158376399305,10.3799223917948));
#82289=CARTESIAN_POINT('Ctrl Pts',(1.23218377333498,9.28904677420117,10.3808563845891));
#82290=CARTESIAN_POINT('Ctrl Pts',(1.00586567563936,9.31770433558347,10.3846761142934));
#82291=CARTESIAN_POINT('Ctrl Pts',(0.83405440267793,9.33465229385922,10.3875229099805));
#82292=CARTESIAN_POINT('Ctrl Pts',(0.260280078110764,9.37528265384661,10.3969714201718));
#82293=CARTESIAN_POINT('Ctrl Pts',(-0.142726959625376,9.3778088918647,10.4035301470733));
#82294=CARTESIAN_POINT('Ctrl Pts',(-0.638212744594506,9.34896005978609,
10.4118357138485));
#82295=CARTESIAN_POINT('Ctrl Pts',(-0.731693548918824,9.34210865938655,
10.4134122411993));
#82296=CARTESIAN_POINT('Ctrl Pts',(-0.903762422886792,9.32689882553345,
10.4163343693944));
#82297=CARTESIAN_POINT('Ctrl Pts',(-0.982377914809031,9.3189463898799,10.4176772420524));
#82298=CARTESIAN_POINT('Ctrl Pts',(-1.16271416244987,9.29839690535284,10.4207765320311));
#82299=CARTESIAN_POINT('Ctrl Pts',(-1.26434759413489,9.2851232798917,10.4225371020645));
#82300=CARTESIAN_POINT('Ctrl Pts',(-1.4271471743319,9.26113861058198,10.4253793702454));
#82301=CARTESIAN_POINT('Ctrl Pts',(-1.48846027190029,9.25148222862207,10.4264548621507));
#82302=CARTESIAN_POINT('Ctrl Pts',(-1.72059244062901,9.21255565636578,10.430544977191));
#82303=CARTESIAN_POINT('Ctrl Pts',(-1.89068364028855,9.17915765302955,10.4335802678523));
#82304=CARTESIAN_POINT('Ctrl Pts',(-2.16696870775239,9.1169024986307,10.4385551699373));
#82305=CARTESIAN_POINT('Ctrl Pts',(-2.27375384451124,9.09085848527484,10.4404888377625));
#82306=CARTESIAN_POINT('Ctrl Pts',(-2.41009923006539,9.05505226965471,10.4429656944004));
#82307=CARTESIAN_POINT('Ctrl Pts',(-2.44010302073046,9.047013162023,10.4435112309203));
#82308=CARTESIAN_POINT('Ctrl Pts',(-2.63568170282498,8.99356680053742,10.4470696416051));
#82309=CARTESIAN_POINT('Ctrl Pts',(-2.80002239407253,8.9437652419079,10.4500713420335));
#82310=CARTESIAN_POINT('Ctrl Pts',(-3.01597626837983,8.87178685542622,10.4539966889123));
#82311=CARTESIAN_POINT('Ctrl Pts',(-3.06889102393441,8.85362201373918,10.4549569064722));
#82312=CARTESIAN_POINT('Ctrl Pts',(-3.16141412992714,8.82093108677411,10.4566311695366));
#82313=CARTESIAN_POINT('Ctrl Pts',(-3.2010927628784,8.80660943088274,10.4573474956131));
#82314=CARTESIAN_POINT('Ctrl Pts',(-3.29779346753757,8.77096626741891,10.4590894986237));
#82315=CARTESIAN_POINT('Ctrl Pts',(-3.35470696247938,8.749356104244,10.4601118077736));
#82316=CARTESIAN_POINT('Ctrl Pts',(-3.48152592292905,8.69978335403628,10.4623870595677));
#82317=CARTESIAN_POINT('Ctrl Pts',(-3.55131316488792,8.6715297379965,10.4636372396361));
#82318=CARTESIAN_POINT('Ctrl Pts',(-3.78214520791813,8.57482257479602,10.4677763243759));
#82319=CARTESIAN_POINT('Ctrl Pts',(-3.94161256469758,8.50269928546953,10.4706427375352));
#82320=CARTESIAN_POINT('Ctrl Pts',(-4.35406821020759,8.30205707136569,10.4781604999754));
#82321=CARTESIAN_POINT('Ctrl Pts',(-4.60340213844989,8.16644046362437,10.4828140784136));
#82322=CARTESIAN_POINT('Ctrl Pts',(-4.93446891518701,7.96638177345371,10.4892668222479));
#82323=CARTESIAN_POINT('Ctrl Pts',(-5.02185289938023,7.91158741487993,10.4909966376514));
#82324=CARTESIAN_POINT('Ctrl Pts',(-5.17469994002073,7.8121915178682,10.4940737066543));
#82325=CARTESIAN_POINT('Ctrl Pts',(-5.24053549278105,7.76818147935085,10.4954163796566));
#82326=CARTESIAN_POINT('Ctrl Pts',(-5.38170407843096,7.67120105499485,10.4983342362967));
#82327=CARTESIAN_POINT('Ctrl Pts',(-5.45683010777319,7.61794391789181,10.4999115334583));
#82328=CARTESIAN_POINT('Ctrl Pts',(-5.69863114852838,7.44111779788576,10.5050690923258));
#82329=CARTESIAN_POINT('Ctrl Pts',(-5.86198911404908,7.31311931897104,10.5086822848689));
#82330=CARTESIAN_POINT('Ctrl Pts',(-6.2022406729732,7.02778536731364,10.5164639555822));
#82331=CARTESIAN_POINT('Ctrl Pts',(-6.37769598684529,6.8689555463784,10.5206369271679));
#82332=CARTESIAN_POINT('Ctrl Pts',(-6.5639400543861,6.68706511831051,10.5251961126254));
#82333=CARTESIAN_POINT('Ctrl Pts',(-6.58086525938917,6.67040938567406,10.5256116405552));
#82334=CARTESIAN_POINT('Ctrl Pts',(-6.68306185774739,6.56907233736003,10.5281275915564));
#82335=CARTESIAN_POINT('Ctrl Pts',(-6.76676120586251,6.4828211511382,10.530217744517));
#82336=CARTESIAN_POINT('Ctrl Pts',(-6.88457529125023,6.35664685625078,10.5331894753512));
#82337=CARTESIAN_POINT('Ctrl Pts',(-6.92004961411017,6.31800993595218,10.5340882664836));
#82338=CARTESIAN_POINT('Ctrl Pts',(-6.98294720420412,6.24833963827138,10.5356874646636));
#82339=CARTESIAN_POINT('Ctrl Pts',(-7.01049257980542,6.21741857037591,10.5363896326605));
#82340=CARTESIAN_POINT('Ctrl Pts',(-7.0670898907368,6.15303091527123,10.5378368926243));
#82341=CARTESIAN_POINT('Ctrl Pts',(-7.09611120003982,6.11953877462381,10.5385815942532));
#82342=CARTESIAN_POINT('Ctrl Pts',(-7.16845388233287,6.0348448351629,10.5404462052842));
#82343=CARTESIAN_POINT('Ctrl Pts',(-7.2114651944997,5.98338140362511,10.5415624072961));
#82344=CARTESIAN_POINT('Ctrl Pts',(-7.34286258718182,5.82268806260461,10.545002969708));
#82345=CARTESIAN_POINT('Ctrl Pts',(-7.42934716756123,5.71192857428453,10.547311731627));
#82346=CARTESIAN_POINT('Ctrl Pts',(-7.72600151146538,5.31386648615137,10.5554545385955));
#82347=CARTESIAN_POINT('Ctrl Pts',(-7.92225948381115,5.01658057194837,10.5612707111013));
#82348=CARTESIAN_POINT('Ctrl Pts',(-8.14911128210152,4.62630381098445,10.5688161945727));
#82349=CARTESIAN_POINT('Ctrl Pts',(-8.19582882814969,4.54302667869393,10.5704204362597));
#82350=CARTESIAN_POINT('Ctrl Pts',(-8.27590875014456,4.39502209205269,10.5732642101574));
#82351=CARTESIAN_POINT('Ctrl Pts',(-8.30980468164635,4.33059244871261,10.5744997392411));
#82352=CARTESIAN_POINT('Ctrl Pts',(-8.37697956259821,4.19921268808174,10.5770149800967));
#82353=CARTESIAN_POINT('Ctrl Pts',(-8.41021496778702,4.13224611552453,10.5782948973097));
#82354=CARTESIAN_POINT('Ctrl Pts',(-8.51804068768397,3.90829552380059,10.582568379875));
#82355=CARTESIAN_POINT('Ctrl Pts',(-8.58906441221237,3.74963508513248,10.5855855671387));
#82356=CARTESIAN_POINT('Ctrl Pts',(-8.76948400339504,3.31452612854787,10.5938164149497));
#82357=CARTESIAN_POINT('Ctrl Pts',(-8.8702047099001,3.03469949200296,10.5990675614163));
#82358=CARTESIAN_POINT('Ctrl Pts',(-8.99525444303348,2.62746346553764,10.6065204232535));
#82359=CARTESIAN_POINT('Ctrl Pts',(-9.03051240725097,2.5035999221864,10.6087618874665));
#82360=CARTESIAN_POINT('Ctrl Pts',(-9.07660802574035,2.32799441099751,10.611887772485));
#82361=CARTESIAN_POINT('Ctrl Pts',(-9.08957798530984,2.27682746302171,10.6127923944102));
#82362=CARTESIAN_POINT('Ctrl Pts',(-9.11199007597492,2.18516603287298,10.6144002930796));
#82363=CARTESIAN_POINT('Ctrl Pts',(-9.12159627948588,2.14471327901367,10.6151053631754));
#82364=CARTESIAN_POINT('Ctrl Pts',(-9.14085835014687,2.06112766235579,10.6165535738545));
#82365=CARTESIAN_POINT('Ctrl Pts',(-9.15047890386238,2.01798772476627,10.6172963705571));
#82366=CARTESIAN_POINT('Ctrl Pts',(-9.1738576626009,1.90954806495943,10.6191535449164));
#82367=CARTESIAN_POINT('Ctrl Pts',(-9.18722420856145,1.84416636789655,10.6202642578069));
#82368=CARTESIAN_POINT('Ctrl Pts',(-9.24935707109379,1.52278981144875,10.6256902528088));
#82369=CARTESIAN_POINT('Ctrl Pts',(-9.28812803990355,1.26497952136606,10.6299420395103));
#82370=CARTESIAN_POINT('Ctrl Pts',(-9.33998953135348,0.784661013487193,
10.6378700542443));
#82371=CARTESIAN_POINT('Ctrl Pts',(-9.35598837409497,0.562653100174978,
10.6415365143556));
#82372=CARTESIAN_POINT('Ctrl Pts',(-9.36631987521606,0.278349433131978,
10.646284592698));
#82373=CARTESIAN_POINT('Ctrl Pts',(-9.36795609253744,0.216390954739834,
10.6473223976902));
#82374=CARTESIAN_POINT('Ctrl Pts',(-9.36982567910073,0.102959950969734,
10.6492288829697));
#82375=CARTESIAN_POINT('Ctrl Pts',(-9.37024986173454,0.0514929715521591,
10.6500963627277));
#82376=CARTESIAN_POINT('Ctrl Pts',(-9.37024999996621,2.5166514242315E-5,
10.6509665184497));
#82377=CARTESIAN_POINT('Ctrl Pts',(-9.36948152355139,3.26635738060604E-5,
10.651410108095));
#82378=CARTESIAN_POINT('Ctrl Pts',(-9.36938165429842,-0.809065474210415,
10.6651497815776));
#82379=CARTESIAN_POINT('Ctrl Pts',(-9.067402610047,-3.16378076784896,10.7051350594858));
#82380=CARTESIAN_POINT('Ctrl Pts',(-7.11741830632754,-6.67998478431112,
10.7713659418197));
#82381=CARTESIAN_POINT('Ctrl Pts',(-3.09251227489688,-9.25830480679301,
10.8501027550967));
#82382=CARTESIAN_POINT('Ctrl Pts',(1.67396187580663,-9.61653220782942,10.9288395683737));
#82383=CARTESIAN_POINT('Ctrl Pts',(6.03902880492754,-7.66876594760393,11.0075763816506));
#82384=CARTESIAN_POINT('Ctrl Pts',(8.95596850446328,-3.88207009376908,11.0863131949276));
#82385=CARTESIAN_POINT('Ctrl Pts',(9.72531423192883,0.835525676515664,11.1650500082046));
#82386=CARTESIAN_POINT('Ctrl Pts',(8.16258094297421,5.35276680000807,11.2437868214815));
#82387=CARTESIAN_POINT('Ctrl Pts',(5.76843016600557,7.55212420695635,11.2973390013619));
#82388=CARTESIAN_POINT('Ctrl Pts',(4.3467929946426,8.30212031658,11.3246455768166));
#82389=CARTESIAN_POINT('Ctrl Pts',(4.29126566285802,8.33069681713329,11.3257065478457));
#82390=CARTESIAN_POINT('Origin',(0.,0.,2.15141010809499));
#82391=CARTESIAN_POINT('',(4.290926628303,8.33003803911004,12.5233065119449));
#82392=CARTESIAN_POINT('',(4.29092662693973,8.33003803981228,12.3256242449617));
#82393=CARTESIAN_POINT('',(4.29092662815669,8.33003803918541,2.15141010809499));
#82394=CARTESIAN_POINT('Ctrl Pts',(4.290926628303,8.33003803911004,12.5233065119449));
#82395=CARTESIAN_POINT('Ctrl Pts',(4.31768745450385,8.31625313906499,12.522789592722));
#82396=CARTESIAN_POINT('Ctrl Pts',(4.34438201512415,8.30233919913577,12.522271794311));
#82397=CARTESIAN_POINT('Ctrl Pts',(4.72117556798361,8.10362911267626,12.5149325355195));
#82398=CARTESIAN_POINT('Ctrl Pts',(5.05928586639326,7.89695680217288,12.5079521348845));
#82399=CARTESIAN_POINT('Ctrl Pts',(5.52861123889295,7.56753317679459,12.4978867421488));
#82400=CARTESIAN_POINT('Ctrl Pts',(5.67098855288102,7.46143349127118,12.4947820990599));
#82401=CARTESIAN_POINT('Ctrl Pts',(5.85405036834622,7.31674750020578,12.4907595613347));
#82402=CARTESIAN_POINT('Ctrl Pts',(5.89752482581023,7.28175120731637,12.4898019715551));
#82403=CARTESIAN_POINT('Ctrl Pts',(5.97336591183359,7.2195755217487,12.4881292753579));
#82404=CARTESIAN_POINT('Ctrl Pts',(6.00586595612234,7.19256179340198,12.4874119204674));
#82405=CARTESIAN_POINT('Ctrl Pts',(6.0858671959053,7.12514520003728,12.4856441854311));
#82406=CARTESIAN_POINT('Ctrl Pts',(6.13314984898458,7.08448633307427,12.4845974780775));
#82407=CARTESIAN_POINT('Ctrl Pts',(6.37412201409765,6.87305118113548,12.4792434036888));
#82408=CARTESIAN_POINT('Ctrl Pts',(6.56109867829342,6.69479268331256,12.4750199897462));
#82409=CARTESIAN_POINT('Ctrl Pts',(6.93719980386168,6.30531893845217,12.4661453635287));
#82410=CARTESIAN_POINT('Ctrl Pts',(7.12458827741994,6.09278502444773,12.4614955802605));
#82411=CARTESIAN_POINT('Ctrl Pts',(7.36482366196115,5.7940475851451,12.4550934906634));
#82412=CARTESIAN_POINT('Ctrl Pts',(7.4263294058878,5.71500187943143,12.4534119729375));
#82413=CARTESIAN_POINT('Ctrl Pts',(7.53356231017847,5.57253387423459,12.4503998626127));
#82414=CARTESIAN_POINT('Ctrl Pts',(7.57978514818136,5.50949652287706,12.4490734015712));
#82415=CARTESIAN_POINT('Ctrl Pts',(7.68051825700837,5.36845222556593,12.4461183062698));
#82416=CARTESIAN_POINT('Ctrl Pts',(7.73463983131766,5.29017831611879,12.4444868184951));
#82417=CARTESIAN_POINT('Ctrl Pts',(7.99457690859153,4.90172330316235,12.4364310473885));
#82418=CARTESIAN_POINT('Ctrl Pts',(8.18297423164529,4.58029270845286,12.429876357283));
#82419=CARTESIAN_POINT('Ctrl Pts',(8.44050656628248,4.07403415704362,12.4198983845134));
#82420=CARTESIAN_POINT('Ctrl Pts',(8.52377396044781,3.89681706447842,12.4164695681118));
#82421=CARTESIAN_POINT('Ctrl Pts',(8.62392438883952,3.66506872529488,12.4121157715288));
#82422=CARTESIAN_POINT('Ctrl Pts',(8.64594635112469,3.61281224799119,12.4111424747668));
#82423=CARTESIAN_POINT('Ctrl Pts',(8.68352633023267,3.52132591469574,12.4094551121683));
#82424=CARTESIAN_POINT('Ctrl Pts',(8.69929610620092,3.48218508807503,12.4087386106085));
#82425=CARTESIAN_POINT('Ctrl Pts',(8.7372908901871,3.3860123137855,12.4069909060387));
#82426=CARTESIAN_POINT('Ctrl Pts',(8.7592224676561,3.32886666533055,12.4059631390923));
#82427=CARTESIAN_POINT('Ctrl Pts',(8.84033349413811,3.1111681580762,12.4020816273175));
#82428=CARTESIAN_POINT('Ctrl Pts',(8.8956713634313,2.94921937233149,12.3992629356841));
#82429=CARTESIAN_POINT('Ctrl Pts',(9.02186337899823,2.54396280847758,12.392294634973));
#82430=CARTESIAN_POINT('Ctrl Pts',(9.08734236000264,2.29912470790987,12.3881573625467));
#82431=CARTESIAN_POINT('Ctrl Pts',(9.16822482178275,1.93873619910536,12.3820580012193));
#82432=CARTESIAN_POINT('Ctrl Pts',(9.19152561894286,1.82507565604921,12.380133548302));
#82433=CARTESIAN_POINT('Ctrl Pts',(9.23122779132561,1.61130474348554,12.3765037452252));
#82434=CARTESIAN_POINT('Ctrl Pts',(9.24812579897358,1.51130362661827,12.3748015710626));
#82435=CARTESIAN_POINT('Ctrl Pts',(9.27528704512642,1.33299261894002,12.3717555245437));
#82436=CARTESIAN_POINT('Ctrl Pts',(9.28618979629196,1.25479007218304,12.3704159184955));
#82437=CARTESIAN_POINT('Ctrl Pts',(9.30797014856434,1.08268686936887,12.3674586564388));
#82438=CARTESIAN_POINT('Ctrl Pts',(9.3184178527194,0.988740516517039,12.3658383951677));
#82439=CARTESIAN_POINT('Ctrl Pts',(9.36438511037658,0.509496321658585,12.3575423377637));
#82440=CARTESIAN_POINT('Ctrl Pts',(9.37743592327813,0.122423116124578,12.3507233469904));
#82441=CARTESIAN_POINT('Ctrl Pts',(9.36132260650613,-0.44852429036887,12.3406939307722));
#82442=CARTESIAN_POINT('Ctrl Pts',(9.35069315540362,-0.63251309503906,12.337469699865));
#82443=CARTESIAN_POINT('Ctrl Pts',(9.32975361413182,-0.872031116921657,
12.3333242380941));
#82444=CARTESIAN_POINT('Ctrl Pts',(9.32435803271197,-0.927948310420261,
12.3323602261645));
#82445=CARTESIAN_POINT('Ctrl Pts',(9.31402587797725,-1.02581213604907,12.3306815858558));
#82446=CARTESIAN_POINT('Ctrl Pts',(9.3093079511679,-1.06777997220159,12.3299646322375));
#82447=CARTESIAN_POINT('Ctrl Pts',(9.29697857528566,-1.17115455288273,12.3282053529332));
#82448=CARTESIAN_POINT('Ctrl Pts',(9.28904231010952,-1.23252042674737,12.3271666006287));
#82449=CARTESIAN_POINT('Ctrl Pts',(9.24422172927056,-1.55402011319282,12.3217443681254));
#82450=CARTESIAN_POINT('Ctrl Pts',(9.19701619811235,-1.81259701714246,12.3174484145618));
#82451=CARTESIAN_POINT('Ctrl Pts',(9.07721437690192,-2.34181399057279,12.3085541546786));
#82452=CARTESIAN_POINT('Ctrl Pts',(9.00322327822113,-2.6118735916883,12.3039578885883));
#82453=CARTESIAN_POINT('Ctrl Pts',(8.88651362181195,-2.97346227375342,12.2976123397843));
#82454=CARTESIAN_POINT('Ctrl Pts',(8.85424671387549,-3.06821076687526,12.2959318633118));
#82455=CARTESIAN_POINT('Ctrl Pts',(8.79408861608191,-3.23600059891934,12.2929208330468));
#82456=CARTESIAN_POINT('Ctrl Pts',(8.7667894685895,-3.30924415002731,12.2915943982546));
#82457=CARTESIAN_POINT('Ctrl Pts',(8.70421178981572,-3.47092884835966,12.2886384179297));
#82458=CARTESIAN_POINT('Ctrl Pts',(8.66849515900038,-3.55919114023889,12.2870060085619));
#82459=CARTESIAN_POINT('Ctrl Pts',(8.48708053475402,-3.98856187417292,12.2789721476223));
#82460=CARTESIAN_POINT('Ctrl Pts',(8.32256218853322,-4.32135600933472,12.272441410467));
#82461=CARTESIAN_POINT('Ctrl Pts',(8.07187973856076,-4.76073033741008,12.2635547296593));
#82462=CARTESIAN_POINT('Ctrl Pts',(8.00248088373386,-4.87648394459782,12.2611888336418));
#82463=CARTESIAN_POINT('Ctrl Pts',(7.88251095357354,-5.06712545621422,12.2572701126206));
#82464=CARTESIAN_POINT('Ctrl Pts',(7.83331329552449,-5.14285350772862,12.2557075220137));
#82465=CARTESIAN_POINT('Ctrl Pts',(7.75723779701233,-5.25632875071231,12.253363359492));
#82466=CARTESIAN_POINT('Ctrl Pts',(7.7311620076357,-5.29460708634321,12.2525721461766));
#82467=CARTESIAN_POINT('Ctrl Pts',(7.6786440189412,-5.3704863776482,12.2510040493329));
#82468=CARTESIAN_POINT('Ctrl Pts',(7.65220678702168,-5.40808923754237,12.2502271370004));
#82469=CARTESIAN_POINT('Ctrl Pts',(7.57421709398963,-5.51730057842604,12.2479689852066));
#82470=CARTESIAN_POINT('Ctrl Pts',(7.52192851287517,-5.58837738256038,12.246497102835));
#82471=CARTESIAN_POINT('Ctrl Pts',(7.26113367411501,-5.93258753177329,12.2393330610985));
#82472=CARTESIAN_POINT('Ctrl Pts',(7.03871492603658,-6.19484872235001,12.2337518715515));
#82473=CARTESIAN_POINT('Ctrl Pts',(6.74167830782909,-6.50839094719336,12.2266361713548));
#82474=CARTESIAN_POINT('Ctrl Pts',(6.68005915448358,-6.5716199517705,12.225177412303));
#82475=CARTESIAN_POINT('Ctrl Pts',(6.52636420886475,-6.72493464546262,12.2215750783265));
#82476=CARTESIAN_POINT('Ctrl Pts',(6.43330688563364,-6.81401043168187,12.2194247562383));
#82477=CARTESIAN_POINT('Ctrl Pts',(6.27791974906918,-6.95672781128971,12.2158752408831));
#82478=CARTESIAN_POINT('Ctrl Pts',(6.21666784493071,-7.01151760209755,12.2144861342732));
#82479=CARTESIAN_POINT('Ctrl Pts',(6.09893920477838,-7.11407020396582,12.2118337656106));
#82480=CARTESIAN_POINT('Ctrl Pts',(6.04260210313655,-7.16198394902114,12.2105719194326));
#82481=CARTESIAN_POINT('Ctrl Pts',(5.88686302153342,-7.29129159602268,12.2071031705798));
#82482=CARTESIAN_POINT('Ctrl Pts',(5.78634521117979,-7.37131591609927,12.2048855036173));
#82483=CARTESIAN_POINT('Ctrl Pts',(5.42307591316495,-7.64851174347065,12.1969491060007));
#82484=CARTESIAN_POINT('Ctrl Pts',(5.15164083068724,-7.833905772279,12.1911523702776));
#82485=CARTESIAN_POINT('Ctrl Pts',(4.72877138774327,-8.0912322490523,12.1824680911832));
#82486=CARTESIAN_POINT('Ctrl Pts',(4.58422578394628,-8.17399488450496,12.1795586532532));
#82487=CARTESIAN_POINT('Ctrl Pts',(4.38900943065454,-8.27896242601902,12.1757386842921));
#82488=CARTESIAN_POINT('Ctrl Pts',(4.34023813127251,-8.30463458656947,12.1747932596799));
#82489=CARTESIAN_POINT('Ctrl Pts',(4.25361451141622,-8.34925986753677,12.1731316073053));
#82490=CARTESIAN_POINT('Ctrl Pts',(4.21585515532868,-8.36838945432873,12.1724132773586));
#82491=CARTESIAN_POINT('Ctrl Pts',(4.12128384976489,-8.4154984859769,12.1706284298743));
#82492=CARTESIAN_POINT('Ctrl Pts',(4.06431553200544,-8.44315904273697,12.1695657843411));
#82493=CARTESIAN_POINT('Ctrl Pts',(3.84812099432839,-8.54543558814328,12.1655727269206));
#82494=CARTESIAN_POINT('Ctrl Pts',(3.68708524587108,-8.61614225157389,12.162678453186));
#82495=CARTESIAN_POINT('Ctrl Pts',(3.41142548659548,-8.72803316537669,12.1577961270468));
#82496=CARTESIAN_POINT('Ctrl Pts',(3.29781525396879,-8.77159058246325,12.1558042439823));
#82497=CARTESIAN_POINT('Ctrl Pts',(3.02021248754538,-8.87186578024343,12.1509626313201));
#82498=CARTESIAN_POINT('Ctrl Pts',(2.85543050044,-8.92626475029556,12.1481095210349));
#82499=CARTESIAN_POINT('Ctrl Pts',(2.56321265425257,-9.01381344288971,12.1430499940944));
#82500=CARTESIAN_POINT('Ctrl Pts',(2.43641070713661,-9.04891123995747,12.1408547127254));
#82501=CARTESIAN_POINT('Ctrl Pts',(2.22887617803558,-9.10167654244627,12.1372531168472));
#82502=CARTESIAN_POINT('Ctrl Pts',(2.14857482402044,-9.12096656544736,12.1358575367338));
#82503=CARTESIAN_POINT('Ctrl Pts',(1.99622560421177,-9.1554403571349,12.1332046202023));
#82504=CARTESIAN_POINT('Ctrl Pts',(1.92423321744663,-9.17084136235773,12.1319488185789));
#82505=CARTESIAN_POINT('Ctrl Pts',(1.72862142527257,-9.21028291423305,12.1285302440255));
#82506=CARTESIAN_POINT('Ctrl Pts',(1.60468698926372,-9.23268232591389,12.1263572770347));
#82507=CARTESIAN_POINT('Ctrl Pts',(1.1269363856613,-9.30911864044745,12.1179578338046));
#82508=CARTESIAN_POINT('Ctrl Pts',(0.770584967044567,-9.3453663649633,12.1116328240685));
#82509=CARTESIAN_POINT('Ctrl Pts',(0.26714107833705,-9.36757962838908,12.102804531421));
#82510=CARTESIAN_POINT('Ctrl Pts',(0.12111309110198,-9.37060533107966,12.1002583678878));
#82511=CARTESIAN_POINT('Ctrl Pts',(-0.0784015928789827,-9.37007459436128,
12.0968222014112));
#82512=CARTESIAN_POINT('Ctrl Pts',(-0.131874998409679,-9.36947456989195,
12.0959054683887));
#82513=CARTESIAN_POINT('Ctrl Pts',(-0.227896953071996,-9.36757491615893,
12.0942685755694));
#82514=CARTESIAN_POINT('Ctrl Pts',(-0.270447174767061,-9.36644303653121,
12.0935466621319));
#82515=CARTESIAN_POINT('Ctrl Pts',(-0.367596158602747,-9.36319622116999,
12.0919054979266));
#82516=CARTESIAN_POINT('Ctrl Pts',(-0.422187097348309,-9.36089357295241,
12.0909882535312));
#82517=CARTESIAN_POINT('Ctrl Pts',(-0.76127936111548,-9.34361830948762,
12.085313904801));
#82518=CARTESIAN_POINT('Ctrl Pts',(-1.04499589300671,-9.31615447717814,
12.0806628034758));
#82519=CARTESIAN_POINT('Ctrl Pts',(-1.34703121687503,-9.27294454852215,
12.0756601624593));
#82520=CARTESIAN_POINT('Ctrl Pts',(-1.36703291916714,-9.27001697393318,
12.0753286546273));
#82521=CARTESIAN_POINT('Ctrl Pts',(-1.55780039781454,-9.24146420012366,
12.0721644163741));
#82522=CARTESIAN_POINT('Ctrl Pts',(-1.72783637447812,-9.21118797701864,
12.0693244979953));
#82523=CARTESIAN_POINT('Ctrl Pts',(-2.02540021078924,-9.14967468117147,
12.0642844711312));
#82524=CARTESIAN_POINT('Ctrl Pts',(-2.15329014571789,-9.12042401441933,
12.062095355139));
#82525=CARTESIAN_POINT('Ctrl Pts',(-2.36056867514636,-9.06841282913668,
12.0585009056206));
#82526=CARTESIAN_POINT('Ctrl Pts',(-2.44034488269627,-9.04727099878149,
12.0571062168502));
#82527=CARTESIAN_POINT('Ctrl Pts',(-2.60027428526652,-9.0026181875827,12.0542860011298));
#82528=CARTESIAN_POINT('Ctrl Pts',(-2.68041328563258,-8.97908375996134,
12.0528604305153));
#82529=CARTESIAN_POINT('Ctrl Pts',(-2.89199885550701,-8.91386231903143,
12.0490629272598));
#82530=CARTESIAN_POINT('Ctrl Pts',(-3.02285790261838,-8.87033983337841,
12.0466793375126));
#82531=CARTESIAN_POINT('Ctrl Pts',(-3.2595648777168,-8.78576677266696,12.0423068772961));
#82532=CARTESIAN_POINT('Ctrl Pts',(-3.36571883771927,-8.74565021119915,
12.0403232838729));
#82533=CARTESIAN_POINT('Ctrl Pts',(-3.70120976738887,-8.61185196119105,
12.0339907080032));
#82534=CARTESIAN_POINT('Ctrl Pts',(-3.92757215616201,-8.51100022322967,
12.0296197323768));
#82535=CARTESIAN_POINT('Ctrl Pts',(-4.22908925915903,-8.36207121424635,
12.0237393932926));
#82536=CARTESIAN_POINT('Ctrl Pts',(-4.30794670470571,-8.32172014609047,
12.0221962295652));
#82537=CARTESIAN_POINT('Ctrl Pts',(-4.44654438578843,-8.24830214068262,
12.0194811946656));
#82538=CARTESIAN_POINT('Ctrl Pts',(-4.50651761873477,-8.21568890375367,
12.0183054206292));
#82539=CARTESIAN_POINT('Ctrl Pts',(-4.60353057891062,-8.16155167566449,
12.0164050495242));
#82540=CARTESIAN_POINT('Ctrl Pts',(-4.64078846161003,-8.1404239460805,12.0156756594924));
#82541=CARTESIAN_POINT('Ctrl Pts',(-4.72316218725313,-8.09296316096412,
12.0140646914092));
#82542=CARTESIAN_POINT('Ctrl Pts',(-4.7682052379348,-8.06650683983694,12.0131846504033));
#82543=CARTESIAN_POINT('Ctrl Pts',(-4.91212813504827,-7.98034608720673,
12.010371898226));
#82544=CARTESIAN_POINT('Ctrl Pts',(-5.01012627566328,-7.91918943520432,
12.0084553236772));
#82545=CARTESIAN_POINT('Ctrl Pts',(-5.36535934533826,-7.68826917166705,
12.0014624309415));
#82546=CARTESIAN_POINT('Ctrl Pts',(-5.61530603107275,-7.50765626233686,
11.996446696073));
#82547=CARTESIAN_POINT('Ctrl Pts',(-5.92189770962247,-7.26222142632168,
11.9899717510559));
#82548=CARTESIAN_POINT('Ctrl Pts',(-5.98717935567564,-7.20849608891725,
11.9885737668783));
#82549=CARTESIAN_POINT('Ctrl Pts',(-6.14741223177839,-7.07294960324019,
11.9850889353469));
#82550=CARTESIAN_POINT('Ctrl Pts',(-6.24146564526041,-6.99009296935818,
11.9829953919736));
#82551=CARTESIAN_POINT('Ctrl Pts',(-6.39401662379642,-6.85016838043453,
11.9795115075811));
#82552=CARTESIAN_POINT('Ctrl Pts',(-6.45348030475094,-6.7941774590525,11.9781304544785));
#82553=CARTESIAN_POINT('Ctrl Pts',(-6.56572897680617,-6.68568093125183,
11.975477552825));
#82554=CARTESIAN_POINT('Ctrl Pts',(-6.61863514620357,-6.63330952727339,
11.9742069615877));
#82555=CARTESIAN_POINT('Ctrl Pts',(-6.76369071321681,-6.48625682465321,
11.9706660948966));
#82556=CARTESIAN_POINT('Ctrl Pts',(-6.85447002140418,-6.39024884019002,
11.9683842175856));
#82557=CARTESIAN_POINT('Ctrl Pts',(-7.16305048776074,-6.04975107257849,
11.9603981760712));
#82558=CARTESIAN_POINT('Ctrl Pts',(-7.37004563413656,-5.79579212824392,
11.9546187912052));
#82559=CARTESIAN_POINT('Ctrl Pts',(-7.65873605046277,-5.40106202987235,
11.9460419306215));
#82560=CARTESIAN_POINT('Ctrl Pts',(-7.75075888256456,-5.26815393992269,
11.9432194906204));
#82561=CARTESIAN_POINT('Ctrl Pts',(-7.86929729639372,-5.08711551261701,
11.939490601839));
#82562=CARTESIAN_POINT('Ctrl Pts',(-7.89889439409746,-5.04103675320063,
11.9385513057282));
#82563=CARTESIAN_POINT('Ctrl Pts',(-7.95067030425345,-4.9588528842676,11.9368951020214));
#82564=CARTESIAN_POINT('Ctrl Pts',(-7.97301122279005,-4.92285204510769,
11.9361761664174));
#82565=CARTESIAN_POINT('Ctrl Pts',(-8.02840211687665,-4.83222727265073,
11.9343821126553));
#82566=CARTESIAN_POINT('Ctrl Pts',(-8.06113938964473,-4.77741485878555,
11.9333109727464));
#82567=CARTESIAN_POINT('Ctrl Pts',(-8.20259025926706,-4.53498784909508,
11.9286256711248));
#82568=CARTESIAN_POINT('Ctrl Pts',(-8.30533315051947,-4.34396634320174,
11.9250685175744));
#82569=CARTESIAN_POINT('Ctrl Pts',(-8.49875368586371,-3.95235907577431,
11.9179085175732));
#82570=CARTESIAN_POINT('Ctrl Pts',(-8.58917751727127,-3.75179769084914,
11.9143077709331));
#82571=CARTESIAN_POINT('Ctrl Pts',(-8.69955341164976,-3.48202162076621,
11.9094874259298));
#82572=CARTESIAN_POINT('Ctrl Pts',(-8.72588707195513,-3.41549394942228,
11.9083007041134));
#82573=CARTESIAN_POINT('Ctrl Pts',(-8.7916714721266,-3.24357223855757,11.9052361840654));
#82574=CARTESIAN_POINT('Ctrl Pts',(-8.82999014524001,-3.13775749349727,
11.9033520720758));
#82575=CARTESIAN_POINT('Ctrl Pts',(-8.89225845062993,-2.9556246716787,11.9001073741583));
#82576=CARTESIAN_POINT('Ctrl Pts',(-8.91715389490071,-2.87964302172243,
11.8987533002724));
#82577=CARTESIAN_POINT('Ctrl Pts',(-8.96751835157484,-2.71900950293269,
11.8958884625798));
#82578=CARTESIAN_POINT('Ctrl Pts',(-8.99276805780504,-2.63429699815862,
11.894376378849));
#82579=CARTESIAN_POINT('Ctrl Pts',(-9.0639176832807,-2.38263649627961,11.8898800803435));
#82580=CARTESIAN_POINT('Ctrl Pts',(-9.10639327740534,-2.21475994489731,
11.886874639974));
#82581=CARTESIAN_POINT('Ctrl Pts',(-9.1739359796859,-1.91286219049046,11.8814692094131));
#82582=CARTESIAN_POINT('Ctrl Pts',(-9.20077589344695,-1.77928806024528,
11.879077549587));
#82583=CARTESIAN_POINT('Ctrl Pts',(-9.25801055837496,-1.45836671059114,
11.8733473993307));
#82584=CARTESIAN_POINT('Ctrl Pts',(-9.28564481324938,-1.270587842022,11.8700069862619));
#82585=CARTESIAN_POINT('Ctrl Pts',(-9.31661131678583,-1.00423294841858,
11.8653271500902));
#82586=CARTESIAN_POINT('Ctrl Pts',(-9.32468663864451,-0.92625556382907,
11.8639642606496));
#82587=CARTESIAN_POINT('Ctrl Pts',(-9.33745343762587,-0.785794629060744,
11.8615268929345));
#82588=CARTESIAN_POINT('Ctrl Pts',(-9.34249847499613,-0.723347889784348,
11.8604495279132));
#82589=CARTESIAN_POINT('Ctrl Pts',(-9.34962152018528,-0.622601895133839,
11.8587238749866));
#82590=CARTESIAN_POINT('Ctrl Pts',(-9.35209128426676,-0.584332367268015,
11.8580713271808));
#82591=CARTESIAN_POINT('Ctrl Pts',(-9.35740965877822,-0.49322360764179,
11.8565251923766));
#82592=CARTESIAN_POINT('Ctrl Pts',(-9.360045745514,-0.440373373567076,11.8556339907632));
#82593=CARTESIAN_POINT('Ctrl Pts',(-9.36757495534957,-0.258464796838727,
11.8525820450118));
#82594=CARTESIAN_POINT('Ctrl Pts',(-9.3702475293314,-0.129329034047358,
11.8504422176639));
#82595=CARTESIAN_POINT('Ctrl Pts',(-9.37025521179012,0.272536502316905,
11.8438187299654));
#82596=CARTESIAN_POINT('Ctrl Pts',(-9.3583545938649,0.545122483164087,11.8393735828791));
#82597=CARTESIAN_POINT('Ctrl Pts',(-9.31843072554074,1.00138145124772,11.8318325973368));
#82598=CARTESIAN_POINT('Ctrl Pts',(-9.29680819974264,1.18544211185105,11.8287637389125));
#82599=CARTESIAN_POINT('Ctrl Pts',(-9.25630800454349,1.45972824430486,11.8241211423927));
#82600=CARTESIAN_POINT('Ctrl Pts',(-9.24153407112169,1.55051358705666,11.8225732072624));
#82601=CARTESIAN_POINT('Ctrl Pts',(-9.21294407325015,1.71123522865247,11.8198104337153));
#82602=CARTESIAN_POINT('Ctrl Pts',(-9.19966197425767,1.78125911624256,11.818599157384));
#82603=CARTESIAN_POINT('Ctrl Pts',(-9.16580725045099,1.94925178333843,11.8156742323284));
#82604=CARTESIAN_POINT('Ctrl Pts',(-9.14446106787503,2.04705563640768,11.8139557171911));
#82605=CARTESIAN_POINT('Ctrl Pts',(-9.05660865640911,2.42073290306697,11.807329844894));
#82606=CARTESIAN_POINT('Ctrl Pts',(-8.97915094847459,2.69387364756707,11.8023557080151));
#82607=CARTESIAN_POINT('Ctrl Pts',(-8.80793681155371,3.20752703268637,11.792837111582));
#82608=CARTESIAN_POINT('Ctrl Pts',(-8.71640624928135,3.44851316553865,11.7883002807386));
#82609=CARTESIAN_POINT('Ctrl Pts',(-8.59051156057177,3.74280535145512,11.7827691006842));
#82610=CARTESIAN_POINT('Ctrl Pts',(-8.56539002994553,3.79994400378733,11.7816958151419));
#82611=CARTESIAN_POINT('Ctrl Pts',(-8.52230334638117,3.89534555620233,11.7799073347184));
#82612=CARTESIAN_POINT('Ctrl Pts',(-8.50464684481857,3.93374546589195,11.7791885367245));
#82613=CARTESIAN_POINT('Ctrl Pts',(-8.46309178607405,4.02253308057806,11.7775292748518));
#82614=CARTESIAN_POINT('Ctrl Pts',(-8.43900205156082,4.07282940435385,11.7765911148939));
#82615=CARTESIAN_POINT('Ctrl Pts',(-8.33667464099605,4.28166997018778,11.7726974978685));
#82616=CARTESIAN_POINT('Ctrl Pts',(-8.25440663762145,4.43819932377759,11.7697829387557));
#82617=CARTESIAN_POINT('Ctrl Pts',(-7.97325843676583,4.93824223131119,11.7603621423175));
#82618=CARTESIAN_POINT('Ctrl Pts',(-7.7569770859817,5.27146970706157,11.7538941366296));
#82619=CARTESIAN_POINT('Ctrl Pts',(-7.46412620310846,5.66544319775799,11.7456803092022));
#82620=CARTESIAN_POINT('Ctrl Pts',(-7.40689871715314,5.74005905394645,11.744098833228));
#82621=CARTESIAN_POINT('Ctrl Pts',(-7.29954870910749,5.87574787192606,11.7411722087659));
#82622=CARTESIAN_POINT('Ctrl Pts',(-7.24975812758066,5.9370726346314,11.7398298505216));
#82623=CARTESIAN_POINT('Ctrl Pts',(-7.13386549974865,6.07618022443728,11.7367384035546));
#82624=CARTESIAN_POINT('Ctrl Pts',(-7.06725595756548,6.15352713880212,11.734985243239));
#82625=CARTESIAN_POINT('Ctrl Pts',(-6.95838822267886,6.27584439643485,11.7321572507454));
#82626=CARTESIAN_POINT('Ctrl Pts',(-6.91692632224145,6.3215124602114,11.7310885981292));
#82627=CARTESIAN_POINT('Ctrl Pts',(-6.75842377658053,6.49266800867973,11.727035484177));
#82628=CARTESIAN_POINT('Ctrl Pts',(-6.63839483318035,6.6153415358973,11.7240307103267));
#82629=CARTESIAN_POINT('Ctrl Pts',(-6.29255806242352,6.94990225579621,11.7155791120917));
#82630=CARTESIAN_POINT('Ctrl Pts',(-6.05951949966166,7.15399553328796,11.7101119736628));
#82631=CARTESIAN_POINT('Ctrl Pts',(-5.77477243179699,7.37946225318874,11.7038423802237));
#82632=CARTESIAN_POINT('Ctrl Pts',(-5.73245273624548,7.41238459799262,11.7029208649586));
#82633=CARTESIAN_POINT('Ctrl Pts',(-5.65614444124179,7.47070378512315,11.7012792237194));
#82634=CARTESIAN_POINT('Ctrl Pts',(-5.62226155175163,7.49623639216644,11.7005573217241));
#82635=CARTESIAN_POINT('Ctrl Pts',(-5.54458789699379,7.55394485498502,11.6989187645929));
#82636=CARTESIAN_POINT('Ctrl Pts',(-5.50068839392389,7.58597159437817,11.6980041082215));
#82637=CARTESIAN_POINT('Ctrl Pts',(-5.3296024309688,7.70852081376689,11.6944785937235));
#82638=CARTESIAN_POINT('Ctrl Pts',(-5.20043979304515,7.79624149439363,11.6918994206645));
#82639=CARTESIAN_POINT('Ctrl Pts',(-4.79518944701295,8.05691307577214,11.683975655643));
#82640=CARTESIAN_POINT('Ctrl Pts',(-4.5122308978803,8.21872634248886,11.6786697306729));
#82641=CARTESIAN_POINT('Ctrl Pts',(-4.09942670878109,8.42703734176916,11.6710071682898));
#82642=CARTESIAN_POINT('Ctrl Pts',(-3.97609987545458,8.48592289238806,11.6687286762741));
#82643=CARTESIAN_POINT('Ctrl Pts',(-3.77555926556937,8.57634433478516,11.6650305411088));
#82644=CARTESIAN_POINT('Ctrl Pts',(-3.6991353764765,8.60958345939405,11.6636228680681));
#82645=CARTESIAN_POINT('Ctrl Pts',(-3.54601561508339,8.67376482080338,11.660804214718));
#82646=CARTESIAN_POINT('Ctrl Pts',(-3.46933314955876,8.70472000513018,11.6593934686362));
#82647=CARTESIAN_POINT('Ctrl Pts',(-3.26893155683732,8.78254934622352,11.6557080694746));
#82648=CARTESIAN_POINT('Ctrl Pts',(-3.14461184481551,8.82782548204847,11.6534230696947));
#82649=CARTESIAN_POINT('Ctrl Pts',(-2.85360994322664,8.92687836152949,11.6480806377425));
#82650=CARTESIAN_POINT('Ctrl Pts',(-2.68629561574012,8.9786448102217,11.6450132582269));
#82651=CARTESIAN_POINT('Ctrl Pts',(-2.22216486717069,9.10810959351065,11.6365483081471));
#82652=CARTESIAN_POINT('Ctrl Pts',(-1.92283108406904,9.17596850813177,11.6311331181685));
#82653=CARTESIAN_POINT('Ctrl Pts',(-1.56936955167219,9.23803990805093,11.6249420034389));
#82654=CARTESIAN_POINT('Ctrl Pts',(-1.51795523852665,9.24662717112057,11.6240466083681));
#82655=CARTESIAN_POINT('Ctrl Pts',(-1.42472817250501,9.26139951555455,11.6224339312574));
#82656=CARTESIAN_POINT('Ctrl Pts',(-1.3829402198343,9.26773153021587,11.6217151280375));
#82657=CARTESIAN_POINT('Ctrl Pts',(-1.28592130504233,9.28176174121341,11.6200559118559));
#82658=CARTESIAN_POINT('Ctrl Pts',(-1.23066173236495,9.28925004202506,11.6191178021681));
#82659=CARTESIAN_POINT('Ctrl Pts',(-0.999990891364524,9.31841411197458,
11.6152251054627));
#82660=CARTESIAN_POINT('Ctrl Pts',(-0.824050520857134,9.33561805437676,
11.6123113916896));
#82661=CARTESIAN_POINT('Ctrl Pts',(-0.251742936183824,9.37527429773653,
11.6028902622184));
#82662=CARTESIAN_POINT('Ctrl Pts',(0.145585102336383,9.37752353199337,11.5964211353018));
#82663=CARTESIAN_POINT('Ctrl Pts',(0.63572453665119,9.34913259230495,11.5882061735526));
#82664=CARTESIAN_POINT('Ctrl Pts',(0.729505680538814,9.3422827683105,11.5866247573239));
#82665=CARTESIAN_POINT('Ctrl Pts',(0.901852109414604,9.32708353275679,11.583698187452));
#82666=CARTESIAN_POINT('Ctrl Pts',(0.980445530950322,9.3191496919704,11.582355823305));
#82667=CARTESIAN_POINT('Ctrl Pts',(1.16034896044711,9.29868777838511,11.5792642833489));
#82668=CARTESIAN_POINT('Ctrl Pts',(1.26157334566924,9.28549604128712,11.5775110349829));
#82669=CARTESIAN_POINT('Ctrl Pts',(1.42359122582153,9.26168333156963,11.5746828729114));
#82670=CARTESIAN_POINT('Ctrl Pts',(1.4845305379115,9.25211106616551,11.5736141390854));
#82671=CARTESIAN_POINT('Ctrl Pts',(1.71463578571621,9.21363451018178,11.5695605870278));
#82672=CARTESIAN_POINT('Ctrl Pts',(1.88309090595818,9.18068653139277,11.5665554520948));
#82673=CARTESIAN_POINT('Ctrl Pts',(2.35254963772108,9.07540022118774,11.5581048889017));
#82674=CARTESIAN_POINT('Ctrl Pts',(2.65101256716353,8.99274772605419,11.5526391767798));
#82675=CARTESIAN_POINT('Ctrl Pts',(2.99575315419421,8.87862177831205,11.5463706182945));
#82676=CARTESIAN_POINT('Ctrl Pts',(3.04652381915877,8.86132914855666,11.5454487995259));
#82677=CARTESIAN_POINT('Ctrl Pts',(3.13718633835103,8.82957796548903,11.5438068165941));
#82678=CARTESIAN_POINT('Ctrl Pts',(3.17713368817045,8.81528256586302,11.5430848734763));
#82679=CARTESIAN_POINT('Ctrl Pts',(3.26800483273021,8.78206584837673,11.5414465312668));
#82680=CARTESIAN_POINT('Ctrl Pts',(3.31886382690908,8.7629720454028,11.5405321276272));
#82681=CARTESIAN_POINT('Ctrl Pts',(3.51504188231941,8.68736876222667,11.5370100553647));
#82682=CARTESIAN_POINT('Ctrl Pts',(3.65910814093394,8.6276777483283,11.5344339918744));
#82683=CARTESIAN_POINT('Ctrl Pts',(3.96697679396072,8.49101944946439,11.5288947975458));
#82684=CARTESIAN_POINT('Ctrl Pts',(4.13014723284788,8.41285790029682,11.525937234304));
#82685=CARTESIAN_POINT('Ctrl Pts',(4.29092665208774,8.33003802685817,11.5229686882669));
#82686=CARTESIAN_POINT('',(-9.37050454109232,0.000215087252814772,11.651410108095));
#82687=CARTESIAN_POINT('Ctrl Pts',(4.29126566285802,8.33069681713329,11.3257065478457));
#82688=CARTESIAN_POINT('Ctrl Pts',(2.97319433370317,9.00902701698846,11.3508911812423));
#82689=CARTESIAN_POINT('Ctrl Pts',(-0.0532844634904993,9.74542354540215,
11.4023214190646));
#82690=CARTESIAN_POINT('Ctrl Pts',(-4.62634724705184,8.5951585916474,11.4799972613125));
#82691=CARTESIAN_POINT('Ctrl Pts',(-8.15249965184079,5.36810855819908,11.5587340745894));
#82692=CARTESIAN_POINT('Ctrl Pts',(-9.29270465558192,2.09218219148154,11.6158716901836));
#82693=CARTESIAN_POINT('Ctrl Pts',(-9.37077357298385,0.273745585815924,
11.6467637013521));
#82694=CARTESIAN_POINT('Ctrl Pts',(-9.37050454109232,0.000215087252814772,
11.651410108095));
#82695=CARTESIAN_POINT('Ctrl Pts',(-9.37024999747657,0.000217463326891779,
11.6515570258181));
#82696=CARTESIAN_POINT('Ctrl Pts',(-9.37025827752224,-0.356560385193558,
11.6574103826834));
#82697=CARTESIAN_POINT('Ctrl Pts',(-9.34988983196303,-0.713046871971945,
11.6632368410448));
#82698=CARTESIAN_POINT('Ctrl Pts',(-9.30017325739077,-1.14660450984069,
11.6705259364666));
#82699=CARTESIAN_POINT('Ctrl Pts',(-9.29009465983067,-1.22558789929131,
11.6718615117638));
#82700=CARTESIAN_POINT('Ctrl Pts',(-9.26850688948526,-1.3791512725268,11.6744751217685));
#82701=CARTESIAN_POINT('Ctrl Pts',(-9.25710100482538,-1.45373971200085,
11.6757524102328));
#82702=CARTESIAN_POINT('Ctrl Pts',(-9.2307098134581,-1.61339421914325,11.6785042685968));
#82703=CARTESIAN_POINT('Ctrl Pts',(-9.21544665626782,-1.69840732695462,
11.6799805256023));
#82704=CARTESIAN_POINT('Ctrl Pts',(-9.16899758383324,-1.93802497468943,
11.6841730948638));
#82705=CARTESIAN_POINT('Ctrl Pts',(-9.13508075466979,-2.09206999482552,
11.6869061554968));
#82706=CARTESIAN_POINT('Ctrl Pts',(-9.06029448911578,-2.39509736007106,
11.6923503286997));
#82707=CARTESIAN_POINT('Ctrl Pts',(-9.01959673036752,-2.54407198973181,
11.69505984241));
#82708=CARTESIAN_POINT('Ctrl Pts',(-8.91965966099798,-2.87726960487477,
11.7011740319431));
#82709=CARTESIAN_POINT('Ctrl Pts',(-8.85835789972438,-3.06080124531979,
11.7045801598438));
#82710=CARTESIAN_POINT('Ctrl Pts',(-8.76403786258211,-3.31654749783302,
11.7093381471368));
#82711=CARTESIAN_POINT('Ctrl Pts',(-8.73571703466561,-3.39044169524443,
11.7107141432158));
#82712=CARTESIAN_POINT('Ctrl Pts',(-8.69839420879118,-3.48425023785669,
11.7124591174993));
#82713=CARTESIAN_POINT('Ctrl Pts',(-8.69025398025114,-3.50450385807561,
11.7128357511666));
#82714=CARTESIAN_POINT('Ctrl Pts',(-8.67671405437051,-3.53785513815779,
11.7134556598215));
#82715=CARTESIAN_POINT('Ctrl Pts',(-8.67135529482384,-3.55096931993642,
11.7136993428759));
#82716=CARTESIAN_POINT('Ctrl Pts',(-8.66142895547395,-3.5751050119766,11.7141476564716));
#82717=CARTESIAN_POINT('Ctrl Pts',(-8.65687002775453,-3.58613004785622,
11.7143523789189));
#82718=CARTESIAN_POINT('Ctrl Pts',(-8.64256086462344,-3.62054817205658,
11.7149912504345));
#82719=CARTESIAN_POINT('Ctrl Pts',(-8.63273676439685,-3.64391044394445,
11.715424564271));
#82720=CARTESIAN_POINT('Ctrl Pts',(-8.60651997705432,-3.7055543621546,11.7165667439014));
#82721=CARTESIAN_POINT('Ctrl Pts',(-8.58996674643086,-3.74376689228073,
11.7172734238478));
#82722=CARTESIAN_POINT('Ctrl Pts',(-8.54766339280212,-3.83966484214877,
11.7190441258113));
#82723=CARTESIAN_POINT('Ctrl Pts',(-8.52158367695186,-3.89720248897324,
11.7201041999243));
#82724=CARTESIAN_POINT('Ctrl Pts',(-8.35623533372941,-4.25240075359274,
11.726645896193));
#82725=CARTESIAN_POINT('Ctrl Pts',(-8.2019689250405,-4.54282827246313,11.7319921452607));
#82726=CARTESIAN_POINT('Ctrl Pts',(-7.91543234453419,-5.01990496137961,
11.7411308290787));
#82727=CARTESIAN_POINT('Ctrl Pts',(-7.79101374945527,-5.21091348249928,
11.7448920640079));
#82728=CARTESIAN_POINT('Ctrl Pts',(-7.60687702618811,-5.47224224650487,
11.7502406899701));
#82729=CARTESIAN_POINT('Ctrl Pts',(-7.55289781558291,-5.54650771505646,
11.7517844227582));
#82730=CARTESIAN_POINT('Ctrl Pts',(-7.45466177793009,-5.67756855555524,
11.7545539473547));
#82731=CARTESIAN_POINT('Ctrl Pts',(-7.41082517599283,-5.73466974739523,
11.7557763210703));
#82732=CARTESIAN_POINT('Ctrl Pts',(-7.30682033736164,-5.86696124805619,
11.7586461930245));
#82733=CARTESIAN_POINT('Ctrl Pts',(-7.24614235792571,-5.94174036772694,
11.7602977143204));
#82734=CARTESIAN_POINT('Ctrl Pts',(-6.91921007521248,-6.33219159654407,
11.7690779390418));
#82735=CARTESIAN_POINT('Ctrl Pts',(-6.63345731220092,-6.63093951384705,
11.7763718719545));
#82736=CARTESIAN_POINT('Ctrl Pts',(-6.24864500311747,-6.98339999644782,
11.7855212771274));
#82737=CARTESIAN_POINT('Ctrl Pts',(-6.16707842948267,-7.05553567062235,
11.7874243282979));
#82738=CARTESIAN_POINT('Ctrl Pts',(-6.04003874193091,-7.16400028434122,
11.7903234887166));
#82739=CARTESIAN_POINT('Ctrl Pts',(-5.99545352098128,-7.20135439857369,
11.79132906257));
#82740=CARTESIAN_POINT('Ctrl Pts',(-5.94885312234674,-7.23966409899496,
11.7923666577955));
#82741=CARTESIAN_POINT('Ctrl Pts',(-5.94718241385495,-7.24103660216315,
11.792403839693));
#82742=CARTESIAN_POINT('Ctrl Pts',(-5.94393575601392,-7.24370188134245,
11.7924760599835));
#82743=CARTESIAN_POINT('Ctrl Pts',(-5.94235985959501,-7.24499472163091,
11.7925110991815));
#82744=CARTESIAN_POINT('Ctrl Pts',(-5.93929179923145,-7.24751003497578,
11.7925792849198));
#82745=CARTESIAN_POINT('Ctrl Pts',(-5.93779967941335,-7.24873256167256,
11.7926124321375));
#82746=CARTESIAN_POINT('Ctrl Pts',(-5.93488928784949,-7.25111560808192,
11.7926770582424));
#82747=CARTESIAN_POINT('Ctrl Pts',(-5.93347105295981,-7.252276172657,11.7927085377008));
#82748=CARTESIAN_POINT('Ctrl Pts',(-5.93069952696751,-7.25454280007351,
11.7927700299057));
#82749=CARTESIAN_POINT('Ctrl Pts',(-5.92934626668653,-7.25564890047763,
11.792800043134));
#82750=CARTESIAN_POINT('Ctrl Pts',(-5.92669662205911,-7.25781337686115,
11.7928587851456));
#82751=CARTESIAN_POINT('Ctrl Pts',(-5.92540026348583,-7.25887178428949,
11.7928875143352));
#82752=CARTESIAN_POINT('Ctrl Pts',(-5.92285706276996,-7.26094703637782,
11.7929438541598));
#82753=CARTESIAN_POINT('Ctrl Pts',(-5.92161024215835,-7.26196390730866,
11.7929714651365));
#82754=CARTESIAN_POINT('Ctrl Pts',(-5.91915935108872,-7.26396173248286,
11.7930257207095));
#82755=CARTESIAN_POINT('Ctrl Pts',(-5.91795529852006,-7.26494270860241,
11.7930523655923));
#82756=CARTESIAN_POINT('Ctrl Pts',(-5.91558366571431,-7.26687396496663,
11.7931048298424));
#82757=CARTESIAN_POINT('Ctrl Pts',(-5.91441610025334,-7.26782426327441,
11.7931306494476));
#82758=CARTESIAN_POINT('Ctrl Pts',(-5.91211155551752,-7.26969904225769,
11.793181594908));
#82759=CARTESIAN_POINT('Ctrl Pts',(-5.9109745882872,-7.2706235376692,11.7932067209585));
#82760=CARTESIAN_POINT('Ctrl Pts',(-5.90872565431023,-7.27245132379723,
11.7932564040477));
#82761=CARTESIAN_POINT('Ctrl Pts',(-5.90761369720132,-7.27335462627414,
11.7932809612428));
#82762=CARTESIAN_POINT('Ctrl Pts',(-5.90540941011123,-7.27514444808972,
11.793329626319));
#82763=CARTESIAN_POINT('Ctrl Pts',(-5.90431708754685,-7.27603097652172,
11.793353734322));
#82764=CARTESIAN_POINT('Ctrl Pts',(-5.9021468208591,-7.27779155331112,11.7934016176372));
#82765=CARTESIAN_POINT('Ctrl Pts',(-5.90106888212153,-7.27866560826097,
11.7934253930383));
#82766=CARTESIAN_POINT('Ctrl Pts',(-5.89892216894355,-7.28040549689321,
11.7934727267066));
#82767=CARTESIAN_POINT('Ctrl Pts',(-5.89785339795813,-7.28127133477668,
11.7934962850305));
#82768=CARTESIAN_POINT('Ctrl Pts',(-5.89571974466799,-7.28299908222527,
11.7935433011611));
#82769=CARTESIAN_POINT('Ctrl Pts',(-5.89465486390261,-7.28386099365109,
11.7935667589929));
#82770=CARTESIAN_POINT('Ctrl Pts',(-5.89252354773943,-7.28558530132259,
11.7936136941554));
#82771=CARTESIAN_POINT('Ctrl Pts',(-5.89145711194916,-7.28644769703149,
11.7936371714784));
#82772=CARTESIAN_POINT('Ctrl Pts',(-5.88931695290851,-7.28817760459654,
11.793684271709));
#82773=CARTESIAN_POINT('Ctrl Pts',(-5.88824322722204,-7.28904511338984,
11.7937078945741));
#82774=CARTESIAN_POINT('Ctrl Pts',(-5.88608232136698,-7.29079021236492,
11.7937554212038));
#82775=CARTESIAN_POINT('Ctrl Pts',(-5.88499513654329,-7.29166779670379,
11.7937793248869));
#82776=CARTESIAN_POINT('Ctrl Pts',(-5.85056202449961,-7.31944976461304,
11.794536153742));
#82777=CARTESIAN_POINT('Ctrl Pts',(-5.81703210747886,-7.3461253965394,11.7952658228471));
#82778=CARTESIAN_POINT('Ctrl Pts',(-5.74226706309223,-7.40477389789333,
11.7968760680792));
#82779=CARTESIAN_POINT('Ctrl Pts',(-5.70094554022213,-7.43663414903239,
11.7977551206528));
#82780=CARTESIAN_POINT('Ctrl Pts',(-5.56128925478417,-7.54246563961377,
11.800693446891));
#82781=CARTESIAN_POINT('Ctrl Pts',(-5.46176384850315,-7.61484483813702,
11.802733836577));
#82782=CARTESIAN_POINT('Ctrl Pts',(-5.2752615515039,-7.74493952598008,11.8064843216716));
#82783=CARTESIAN_POINT('Ctrl Pts',(-5.18869012234299,-7.80320239063289,
11.8081971854807));
#82784=CARTESIAN_POINT('Ctrl Pts',(-4.9081546311232,-7.98527060121895,11.8136812670319));
#82785=CARTESIAN_POINT('Ctrl Pts',(-4.71059719536616,-8.1033821584547,11.8174453030595));
#82786=CARTESIAN_POINT('Ctrl Pts',(-4.4112387782878,-8.2677062937956,11.8230899708851));
#82787=CARTESIAN_POINT('Ctrl Pts',(-4.31263626913686,-8.31956508827047,
11.824939685282));
#82788=CARTESIAN_POINT('Ctrl Pts',(-4.12498324431703,-8.41402624101412,
11.828449725641));
#82789=CARTESIAN_POINT('Ctrl Pts',(-4.03613839187225,-8.45700367568024,
11.8301073371404));
#82790=CARTESIAN_POINT('Ctrl Pts',(-3.8750992870705,-8.53178825929391,11.8331075391023));
#82791=CARTESIAN_POINT('Ctrl Pts',(-3.80315071724062,-8.56410240331542,
11.8344464038826));
#82792=CARTESIAN_POINT('Ctrl Pts',(-3.64199001933242,-8.6340527835849,11.8374429479094));
#82793=CARTESIAN_POINT('Ctrl Pts',(-3.55258519599724,-8.6712223552983,11.8391036840123));
#82794=CARTESIAN_POINT('Ctrl Pts',(-3.12233623126596,-8.84232479916431,
11.847088160262));
#82795=CARTESIAN_POINT('Ctrl Pts',(-2.77441251175253,-8.95758472270911,
11.8535362898012));
#82796=CARTESIAN_POINT('Ctrl Pts',(-2.29028575988383,-9.08704483258368,
11.8623400492072));
#82797=CARTESIAN_POINT('Ctrl Pts',(-2.15919256488033,-9.11908329911449,
11.8647057340253));
#82798=CARTESIAN_POINT('Ctrl Pts',(-1.98486550951542,-9.15771787966835,
11.8678121401052));
#82799=CARTESIAN_POINT('Ctrl Pts',(-1.94221241042051,-9.16685872117275,
11.8685690679227));
#82800=CARTESIAN_POINT('Ctrl Pts',(-1.83557692591325,-9.18893374027633,
11.8704524922185));
#82801=CARTESIAN_POINT('Ctrl Pts',(-1.77152020411468,-9.20149781989316,
11.8715758751053));
#82802=CARTESIAN_POINT('Ctrl Pts',(-1.66555002747531,-9.22113519650408,
11.8734183512872));
#82803=CARTESIAN_POINT('Ctrl Pts',(-1.62371049846678,-9.22859444566639,
11.8741416277109));
#82804=CARTESIAN_POINT('Ctrl Pts',(-1.5287348974826,-9.24486103343541,11.8757735556247));
#82805=CARTESIAN_POINT('Ctrl Pts',(-1.4755708388355,-9.25349537372788,11.8766803122785));
#82806=CARTESIAN_POINT('Ctrl Pts',(-1.2934246070044,-9.28146797229241,11.8797681129884));
#82807=CARTESIAN_POINT('Ctrl Pts',(-1.16411436464797,-9.29857154877264,
11.8819281225086));
#82808=CARTESIAN_POINT('Ctrl Pts',(-0.742275708960373,-9.34542958307081,
11.8889214358734));
#82809=CARTESIAN_POINT('Ctrl Pts',(-0.448696487790422,-9.36411763976509,
11.8937104597581));
#82810=CARTESIAN_POINT('Ctrl Pts',(-0.0719032005515667,-9.37034024772009,
11.8999256695569));
#82811=CARTESIAN_POINT('Ctrl Pts',(0.0109332770555784,-9.37060973820518,
11.9012958804959));
#82812=CARTESIAN_POINT('Ctrl Pts',(0.217470262225723,-9.36854294601706,
11.9047265089184));
#82813=CARTESIAN_POINT('Ctrl Pts',(0.341141269917283,-9.36485519204564,
11.9067935901955));
#82814=CARTESIAN_POINT('Ctrl Pts',(0.546042859255265,-9.35468090271269,
11.9102469638122));
#82815=CARTESIAN_POINT('Ctrl Pts',(0.627326774636237,-9.34958173808023,
11.9116243333842));
#82816=CARTESIAN_POINT('Ctrl Pts',(0.783015607445258,-9.33777548820628,
11.9142780418331));
#82817=CARTESIAN_POINT('Ctrl Pts',(0.857427151325094,-9.33123695773185,
11.9155532009062));
#82818=CARTESIAN_POINT('Ctrl Pts',(1.06510286449693,-9.31048338520604,11.9191316300244));
#82819=CARTESIAN_POINT('Ctrl Pts',(1.19815171700217,-9.29429810635462,11.9214469468847));
#82820=CARTESIAN_POINT('Ctrl Pts',(1.67231561757276,-9.22626546439931,11.9297744272908));
#82821=CARTESIAN_POINT('Ctrl Pts',(2.01085680972513,-9.15844240941028,11.9358713800179));
#82822=CARTESIAN_POINT('Ctrl Pts',(2.48447884280982,-9.03602450417845,11.9444400285374));
#82823=CARTESIAN_POINT('Ctrl Pts',(2.62322371920065,-8.99672559744819,11.9469533426583));
#82824=CARTESIAN_POINT('Ctrl Pts',(2.81194389204922,-8.93853443819587,11.9503543376118));
#82825=CARTESIAN_POINT('Ctrl Pts',(2.86274628214175,-8.92239374249897,11.9512680596098));
#82826=CARTESIAN_POINT('Ctrl Pts',(2.95389400960604,-8.89257610321638,11.9529024767391));
#82827=CARTESIAN_POINT('Ctrl Pts',(2.99428889907819,-8.87905589350197,11.9536248882178));
#82828=CARTESIAN_POINT('Ctrl Pts',(3.08648844251275,-8.8474958697544,11.9552701430638));
#82829=CARTESIAN_POINT('Ctrl Pts',(3.13822969621515,-8.82927564766102,11.9561909434569));
#82830=CARTESIAN_POINT('Ctrl Pts',(3.49314319483674,-8.70078205373212,11.9624985801331));
#82831=CARTESIAN_POINT('Ctrl Pts',(3.79060579018193,-8.57536980418779,11.9677500916013));
#82832=CARTESIAN_POINT('Ctrl Pts',(4.25137374587279,-8.35243828596401,11.9761518310564));
#82833=CARTESIAN_POINT('Ctrl Pts',(4.41920331139903,-8.26486817217375,11.9792696752741));
#82834=CARTESIAN_POINT('Ctrl Pts',(4.68363508910786,-8.11653429246689,11.9843156648112));
#82835=CARTESIAN_POINT('Ctrl Pts',(4.78197973690698,-8.05898481659339,11.9862227861367));
#82836=CARTESIAN_POINT('Ctrl Pts',(4.94765415409519,-7.95793460858439,11.98949341468));
#82837=CARTESIAN_POINT('Ctrl Pts',(5.01552001053204,-7.91533725447361,11.9908501167608));
#82838=CARTESIAN_POINT('Ctrl Pts',(5.15663836149598,-7.82421782497642,11.993708238018));
#82839=CARTESIAN_POINT('Ctrl Pts',(5.22977160146937,-7.77552523719921,11.9952108541188));
#82840=CARTESIAN_POINT('Ctrl Pts',(5.44146337477904,-7.63024159168775,11.9996240581793));
#82841=CARTESIAN_POINT('Ctrl Pts',(5.57810783188802,-7.53092445428313,12.002554594613));
#82842=CARTESIAN_POINT('Ctrl Pts',(5.94788856088106,-7.24656880777628,12.01070155656));
#82843=CARTESIAN_POINT('Ctrl Pts',(6.17500838431288,-7.05403492187524,12.0159580231464));
#82844=CARTESIAN_POINT('Ctrl Pts',(6.49226981816965,-6.75800325425452,12.0235534315158));
#82845=CARTESIAN_POINT('Ctrl Pts',(6.589917005805,-6.66281992903234,12.0259280685498));
#82846=CARTESIAN_POINT('Ctrl Pts',(6.72225980316967,-6.52806002571574,12.0291796694575));
#82847=CARTESIAN_POINT('Ctrl Pts',(6.75875136620614,-6.49027153107556,12.0300798561044));
#82848=CARTESIAN_POINT('Ctrl Pts',(6.82436717948298,-6.42117015036403,12.0317034536345));
#82849=CARTESIAN_POINT('Ctrl Pts',(6.85359841793103,-6.38996105031942,12.0324284118396));
#82850=CARTESIAN_POINT('Ctrl Pts',(6.92854065598597,-6.3088421883687,12.0342923907706));
#82851=CARTESIAN_POINT('Ctrl Pts',(6.97392643238248,-6.25863527671691,12.0354266419463));
#82852=CARTESIAN_POINT('Ctrl Pts',(7.14205487513995,-6.06854746489289,12.039657781273));
#82853=CARTESIAN_POINT('Ctrl Pts',(7.26116580383477,-5.92551159874945,12.0427160681941));
#82854=CARTESIAN_POINT('Ctrl Pts',(7.52068723082718,-5.59427674264096,12.0496174400519));
#82855=CARTESIAN_POINT('Ctrl Pts',(7.65844368588057,-5.40415663244292,12.0534554557688));
#82856=CARTESIAN_POINT('Ctrl Pts',(7.83013353655825,-5.1474353838737,12.0585593638696));
#82857=CARTESIAN_POINT('Ctrl Pts',(7.87061773326577,-5.08531795545669,12.0597882999757));
#82858=CARTESIAN_POINT('Ctrl Pts',(7.97209948606517,-4.9254929656291,12.062938268785));
#82859=CARTESIAN_POINT('Ctrl Pts',(8.03204040018019,-4.82712938370015,12.0648657164095));
#82860=CARTESIAN_POINT('Ctrl Pts',(8.13065694977619,-4.65837390049898,12.0681593441981));
#82861=CARTESIAN_POINT('Ctrl Pts',(8.17026877206463,-4.58854421237305,12.0695184580675));
#82862=CARTESIAN_POINT('Ctrl Pts',(8.25112824350716,-4.44163359396412,12.0723712670849));
#82863=CARTESIAN_POINT('Ctrl Pts',(8.29220441069198,-4.36446700522779,12.0738660554183));
#82864=CARTESIAN_POINT('Ctrl Pts',(8.40790182903271,-4.13958420977134,12.0782122273806));
#82865=CARTESIAN_POINT('Ctrl Pts',(8.47969712123332,-3.99045198665932,12.081082558403));
#82866=CARTESIAN_POINT('Ctrl Pts',(8.6072584635711,-3.70647438194532,12.086517603255));
#82867=CARTESIAN_POINT('Ctrl Pts',(8.6638981718463,-3.57207488314956,12.0890772590472));
#82868=CARTESIAN_POINT('Ctrl Pts',(8.78743743275953,-3.25868419831798,12.0949984299578));
#82869=CARTESIAN_POINT('Ctrl Pts',(8.85204542551602,-3.07885875328019,12.0983615603606));
#82870=CARTESIAN_POINT('Ctrl Pts',(8.93542891699001,-2.82238919875888,12.1030684412296));
#82871=CARTESIAN_POINT('Ctrl Pts',(8.95880374598082,-2.74729070118157,12.1044358897558));
#82872=CARTESIAN_POINT('Ctrl Pts',(8.99913608122187,-2.61171935539102,12.1068803476539));
#82873=CARTESIAN_POINT('Ctrl Pts',(9.01643633490976,-2.55135337505736,12.1079602680587));
#82874=CARTESIAN_POINT('Ctrl Pts',(9.04332681009985,-2.45383315457247,12.1096887491837));
#82875=CARTESIAN_POINT('Ctrl Pts',(9.05329786412195,-2.41678603573668,12.1103415980538));
#82876=CARTESIAN_POINT('Ctrl Pts',(9.07645680296243,-2.3285848730109,12.1118865447318));
#82877=CARTESIAN_POINT('Ctrl Pts',(9.08944016255843,-2.27737857085425,12.1127762760613));
#82878=CARTESIAN_POINT('Ctrl Pts',(9.13261111436083,-2.10086012345344,12.115822590472));
#82879=CARTESIAN_POINT('Ctrl Pts',(9.16064577368532,-1.97503625220237,12.1179583196231));
#82880=CARTESIAN_POINT('Ctrl Pts',(9.23312794103505,-1.61487177038786,12.1240137606862));
#82881=CARTESIAN_POINT('Ctrl Pts',(9.2712368780749,-1.37935833436649,12.1279059235321));
#82882=CARTESIAN_POINT('Ctrl Pts',(9.32678024421574,-0.927275916618748,
12.1353907912067));
#82883=CARTESIAN_POINT('Ctrl Pts',(9.3457518377083,-0.711050291764133,12.1389763471467));
#82884=CARTESIAN_POINT('Ctrl Pts',(9.36210116757148,-0.401592965387163,
12.1441635712763));
#82885=CARTESIAN_POINT('Ctrl Pts',(9.36562249229279,-0.308756313786629,
12.1457265801955));
#82886=CARTESIAN_POINT('Ctrl Pts',(9.36958498997166,-0.136812392930031,
12.1486366355776));
#82887=CARTESIAN_POINT('Ctrl Pts',(9.37040600137804,-0.0577221845912397,
12.1499811244683));
#82888=CARTESIAN_POINT('Ctrl Pts',(9.36999326106826,0.123264445837158,12.153072276048));
#82889=CARTESIAN_POINT('Ctrl Pts',(9.36809882276587,0.22514931227928,12.1548229535946));
#82890=CARTESIAN_POINT('Ctrl Pts',(9.3521635163753,0.681524574679411,12.1627114301312));
#82891=CARTESIAN_POINT('Ctrl Pts',(9.31965950871019,1.03507615203196,12.1689609089425));
#82892=CARTESIAN_POINT('Ctrl Pts',(9.23878266715062,1.57586931631202,12.1785654032703));
#82893=CARTESIAN_POINT('Ctrl Pts',(9.20454378320442,1.76489188325154,12.1819283182393));
#82894=CARTESIAN_POINT('Ctrl Pts',(9.15273601766901,2.00803539605582,12.1862152699104));
#82895=CARTESIAN_POINT('Ctrl Pts',(9.14045113240248,2.06323432434942,12.1871858046079));
#82896=CARTESIAN_POINT('Ctrl Pts',(9.11812559441515,2.15943329564272,12.1888705597519));
#82897=CARTESIAN_POINT('Ctrl Pts',(9.10830621776878,2.20048275670053,12.1895871830892));
#82898=CARTESIAN_POINT('Ctrl Pts',(9.08352143422814,2.30108534985934,12.1913382648875));
#82899=CARTESIAN_POINT('Ctrl Pts',(9.06824737958857,2.3605602980635,12.1923692471056));
#82900=CARTESIAN_POINT('Ctrl Pts',(8.96970950176652,2.72917483732367,12.1987437884873));
#82901=CARTESIAN_POINT('Ctrl Pts',(8.87123168093822,3.03402934284792,12.2039560889006));
#82902=CARTESIAN_POINT('Ctrl Pts',(8.69912827900111,3.48619190754937,12.2118970419112));
#82903=CARTESIAN_POINT('Ctrl Pts',(8.63691643007624,3.63758728599481,12.2145913868715));
#82904=CARTESIAN_POINT('Ctrl Pts',(8.51947382736378,3.90336509756044,12.2194146876727));
#82905=CARTESIAN_POINT('Ctrl Pts',(8.46582257005918,4.01840036236476,12.2215341691647));
#82906=CARTESIAN_POINT('Ctrl Pts',(8.37373213570585,4.20581777581546,12.2250480153088));
#82907=CARTESIAN_POINT('Ctrl Pts',(8.33665082353039,4.27884868316025,12.2264327298131));
#82908=CARTESIAN_POINT('Ctrl Pts',(8.25946693929844,4.42604771072856,12.2292567500072));
#82909=CARTESIAN_POINT('Ctrl Pts',(8.21931116987626,4.50017958651058,12.2306963387084));
#82910=CARTESIAN_POINT('Ctrl Pts',(8.10824983003253,4.69876403269093,12.234600582531));
#82911=CARTESIAN_POINT('Ctrl Pts',(8.03548238136048,4.82214904975152,12.2370781948386));
#82912=CARTESIAN_POINT('Ctrl Pts',(7.78509626690922,5.22528942198437,12.2453399415565));
#82913=CARTESIAN_POINT('Ctrl Pts',(7.59547031766549,5.49729050660566,12.251195002146));
#82914=CARTESIAN_POINT('Ctrl Pts',(7.30450904084259,5.87076863777904,12.2594863465227));
#82915=CARTESIAN_POINT('Ctrl Pts',(7.21464150038117,5.98086322676164,12.2619627342723));
#82916=CARTESIAN_POINT('Ctrl Pts',(7.08779656307944,6.12923691234635,12.2653240936072));
#82917=CARTESIAN_POINT('Ctrl Pts',(7.05294561096457,6.16930818432155,12.2662343416934));
#82918=CARTESIAN_POINT('Ctrl Pts',(6.98950372935933,6.24101277806357,12.2678659305045));
#82919=CARTESIAN_POINT('Ctrl Pts',(6.96103405399495,6.27275121275399,12.2685889444367));
#82920=CARTESIAN_POINT('Ctrl Pts',(6.89527172062327,6.34506500475445,12.2702390267609));
#82921=CARTESIAN_POINT('Ctrl Pts',(6.85783573197619,6.38550789732074,12.2711640091832));
#82922=CARTESIAN_POINT('Ctrl Pts',(6.63309201289867,6.62404716998508,12.2766402117316));
#82923=CARTESIAN_POINT('Ctrl Pts',(6.43756735176066,6.81422323365515,12.2810950206056));
#82924=CARTESIAN_POINT('Ctrl Pts',(6.05015218479438,7.15946255742574,12.2896018127144));
#82925=CARTESIAN_POINT('Ctrl Pts',(5.85988667665508,7.31600801767173,12.2936474633893));
#82926=CARTESIAN_POINT('Ctrl Pts',(5.57564918258047,7.53166186261353,12.2995900297831));
#82927=CARTESIAN_POINT('Ctrl Pts',(5.48644825185093,7.59688618555996,12.3014408343938));
#82928=CARTESIAN_POINT('Ctrl Pts',(5.33094146338329,7.70642610698145,12.3046482390422));
#82929=CARTESIAN_POINT('Ctrl Pts',(5.26518495138276,7.75150099152724,12.3059987469718));
#82930=CARTESIAN_POINT('Ctrl Pts',(5.12461637582803,7.84524415887816,12.3088748448073));
#82931=CARTESIAN_POINT('Ctrl Pts',(5.04966796620778,7.89369383081742,12.3104019446758));
#82932=CARTESIAN_POINT('Ctrl Pts',(4.82136350883556,8.03669671835688,12.3150351412617));
#82933=CARTESIAN_POINT('Ctrl Pts',(4.66596225545873,8.12790478021591,12.318164657097));
#82934=CARTESIAN_POINT('Ctrl Pts',(4.45941974016268,8.24125203543735,12.32228413474));
#82935=CARTESIAN_POINT('Ctrl Pts',(4.41057468704577,8.26749602083678,12.3232554227997));
#82936=CARTESIAN_POINT('Ctrl Pts',(4.33802651072136,8.30564954902547,12.3246931548461));
#82937=CARTESIAN_POINT('Ctrl Pts',(4.31450196866873,8.31789403025546,12.3251585999007));
#82938=CARTESIAN_POINT('Ctrl Pts',(4.29092662693973,8.33003803981228,12.3256242449617));
#82939=CARTESIAN_POINT('Origin',(0.,0.,2.15141010809499));
#82940=CARTESIAN_POINT('',(4.29092664483271,8.33003803059534,13.5226410022223));
#82941=CARTESIAN_POINT('',(4.29092662791762,8.33003803930856,13.3252837277684));
#82942=CARTESIAN_POINT('',(4.29092662815669,8.33003803918541,2.15141010809499));
#82943=CARTESIAN_POINT('',(-9.37024987213592,-9.34868092301034E-5,12.8489977063995));
#82944=CARTESIAN_POINT('Ctrl Pts',(4.2909266448327,8.33003803059535,13.5226410022224));
#82945=CARTESIAN_POINT('Ctrl Pts',(4.40796820389162,8.26974818048013,13.5203344890077));
#82946=CARTESIAN_POINT('Ctrl Pts',(4.52374228459837,8.20698994738235,13.5180376176366));
#82947=CARTESIAN_POINT('Ctrl Pts',(4.68510179281196,8.11506768681626,13.5148314800693));
#82948=CARTESIAN_POINT('Ctrl Pts',(4.73180090659712,8.08792696355659,13.51390303251));
#82949=CARTESIAN_POINT('Ctrl Pts',(4.8148018533311,8.03872331042009,13.5122535599883));
#82950=CARTESIAN_POINT('Ctrl Pts',(4.85119319956073,8.01681444888224,13.5115306921446));
#82951=CARTESIAN_POINT('Ctrl Pts',(4.93350281422246,7.9664954971173,13.509896912888));
#82952=CARTESIAN_POINT('Ctrl Pts',(4.97932691627481,7.93793449218484,13.508987925753));
#82953=CARTESIAN_POINT('Ctrl Pts',(5.15313839658482,7.82750486555867,13.5055376762997));
#82954=CARTESIAN_POINT('Ctrl Pts',(5.27937501874081,7.74292369971175,13.5030263768984));
#82955=CARTESIAN_POINT('Ctrl Pts',(5.733786246584,7.42217762197547,13.4938767684595));
#82956=CARTESIAN_POINT('Ctrl Pts',(6.04863860605967,7.16791440375308,13.4873027375562));
#82957=CARTESIAN_POINT('Ctrl Pts',(6.42014281635164,6.82594193639402,13.4788738896804));
#82958=CARTESIAN_POINT('Ctrl Pts',(6.49309802369832,6.75658161286644,13.4771846073928));
#82959=CARTESIAN_POINT('Ctrl Pts',(6.62129752846268,6.63070482702753,13.4741509746564));
#82960=CARTESIAN_POINT('Ctrl Pts',(6.67697115520701,6.57463942908205,13.4728107216251));
#82961=CARTESIAN_POINT('Ctrl Pts',(6.79716265176064,6.45050074814443,13.4698656871598));
#82962=CARTESIAN_POINT('Ctrl Pts',(6.86138102899827,6.38214935078093,13.4682584478128));
#82963=CARTESIAN_POINT('Ctrl Pts',(7.0786694477314,6.14380561256954,13.4627021973097));
#82964=CARTESIAN_POINT('Ctrl Pts',(7.22653440708546,5.9691798735086,13.4587117230776));
#82965=CARTESIAN_POINT('Ctrl Pts',(7.51686139568803,5.59969106398734,13.4504665526502));
#82966=CARTESIAN_POINT('Ctrl Pts',(7.65848604660077,5.40438125065069,13.4462122005262));
#82967=CARTESIAN_POINT('Ctrl Pts',(7.85563123530068,5.10916813071561,13.4400105444198));
#82968=CARTESIAN_POINT('Ctrl Pts',(7.91711453012031,5.01336600708722,13.4380321912112));
#82969=CARTESIAN_POINT('Ctrl Pts',(8.00412189833516,4.87219887262912,13.4351781170507));
#82970=CARTESIAN_POINT('Ctrl Pts',(8.03103757062529,4.82770388210212,13.4342872034832));
#82971=CARTESIAN_POINT('Ctrl Pts',(8.07947530161691,4.74610404549726,13.4326706901483));
#82972=CARTESIAN_POINT('Ctrl Pts',(8.10111556349292,4.70907118071052,13.4319436604033));
#82973=CARTESIAN_POINT('Ctrl Pts',(8.15678005902085,4.61229347094315,13.4300597077864));
#82974=CARTESIAN_POINT('Ctrl Pts',(8.19040239141105,4.55232036364884,13.4289077786814));
#82975=CARTESIAN_POINT('Ctrl Pts',(8.26626105152168,4.41344778591673,13.4262702732956));
#82976=CARTESIAN_POINT('Ctrl Pts',(8.30803324173971,4.33430234683507,13.424788962643));
#82977=CARTESIAN_POINT('Ctrl Pts',(8.46390505203484,4.02843797199665,13.4191282788039));
#82978=CARTESIAN_POINT('Ctrl Pts',(8.5699096572916,3.79771642036605,13.4149886084481));
#82979=CARTESIAN_POINT('Ctrl Pts',(8.74311171727017,3.3764278537845,13.4074993697508));
#82980=CARTESIAN_POINT('Ctrl Pts',(8.81376294545501,3.1874519517316,13.4041647016374));
#82981=CARTESIAN_POINT('Ctrl Pts',(8.90845995259179,2.90686178372168,13.3992102782388));
#82982=CARTESIAN_POINT('Ctrl Pts',(8.93730494022251,2.81692820416644,13.3976220813808));
#82983=CARTESIAN_POINT('Ctrl Pts',(8.98776167940976,2.65102996634805,13.3946892785676));
#82984=CARTESIAN_POINT('Ctrl Pts',(9.00978204245337,2.57519851702767,13.3933475467423));
#82985=CARTESIAN_POINT('Ctrl Pts',(9.05791628867108,2.40125865897946,13.3902663388288));
#82986=CARTESIAN_POINT('Ctrl Pts',(9.08339946490536,2.30298604670164,13.3885228975579));
#82987=CARTESIAN_POINT('Ctrl Pts',(9.13461457037467,2.09138765711117,13.3847635747976));
#82988=CARTESIAN_POINT('Ctrl Pts',(9.15984541991545,1.97795790561759,13.3827450348816));
#82989=CARTESIAN_POINT('Ctrl Pts',(9.23354833862487,1.61487913396577,13.3762794186493));
#82990=CARTESIAN_POINT('Ctrl Pts',(9.27397074063018,1.3637139732343,13.3717973772946));
#82991=CARTESIAN_POINT('Ctrl Pts',(9.32551032435178,0.932177414901172,13.3641670438992));
#82992=CARTESIAN_POINT('Ctrl Pts',(9.34172122356433,0.752557259324356,13.3610125667854));
#82993=CARTESIAN_POINT('Ctrl Pts',(9.35615234546906,0.516834318716708,13.3569402614641));
#82994=CARTESIAN_POINT('Ctrl Pts',(9.3590667275941,0.461057949065512,13.3559816784151));
#82995=CARTESIAN_POINT('Ctrl Pts',(9.36330690478786,0.363109810734202,13.3543089746373));
#82996=CARTESIAN_POINT('Ctrl Pts',(9.36484685291686,0.320949147487481,13.3535925924372));
#82997=CARTESIAN_POINT('Ctrl Pts',(9.36791664019424,0.21781401273862,13.3518486041548));
#82998=CARTESIAN_POINT('Ctrl Pts',(9.36913596651226,0.156832353626897,13.3508243897097));
#82999=CARTESIAN_POINT('Ctrl Pts',(9.37053194993767,0.0203589357649303,
13.348543933461));
#83000=CARTESIAN_POINT('Ctrl Pts',(9.37039188189736,-0.0551318765680639,
13.3472904737359));
#83001=CARTESIAN_POINT('Ctrl Pts',(9.36688762051223,-0.306505458640138,
13.3431329580897));
#83002=CARTESIAN_POINT('Ctrl Pts',(9.35948297504986,-0.482294432059399,
13.3402515862976));
#83003=CARTESIAN_POINT('Ctrl Pts',(9.32732807791046,-0.939225902899539,
13.3327437566695));
#83004=CARTESIAN_POINT('Ctrl Pts',(9.29481931695558,-1.21964246199828,13.328114885758));
#83005=CARTESIAN_POINT('Ctrl Pts',(9.23320783818254,-1.60003373388339,13.3216867735744));
#83006=CARTESIAN_POINT('Ctrl Pts',(9.21502623143167,-1.70162464059846,13.3199559355863));
#83007=CARTESIAN_POINT('Ctrl Pts',(9.17993312386435,-1.88060745799853,13.3168777623345));
#83008=CARTESIAN_POINT('Ctrl Pts',(9.16371137205373,-1.9581242109515,13.3155350199275));
#83009=CARTESIAN_POINT('Ctrl Pts',(9.12651509793152,-2.12527156590577,13.3126177900176));
#83010=CARTESIAN_POINT('Ctrl Pts',(9.10519851538116,-2.21481760072378,13.311041197156));
#83011=CARTESIAN_POINT('Ctrl Pts',(9.03165830748466,-2.50471503646468,13.3058919526134));
#83012=CARTESIAN_POINT('Ctrl Pts',(8.9741135292501,-2.70365217101305,13.3022865354116));
#83013=CARTESIAN_POINT('Ctrl Pts',(8.83681892454648,-3.12540380615162,13.2945142281144));
#83014=CARTESIAN_POINT('Ctrl Pts',(8.75512353169543,-3.34743625235401,13.2903427351711));
#83015=CARTESIAN_POINT('Ctrl Pts',(8.6119601426669,-3.6952990829628,13.2837544929934));
#83016=CARTESIAN_POINT('Ctrl Pts',(8.55592301990391,-3.82325440791566,13.2813199846486));
#83017=CARTESIAN_POINT('Ctrl Pts',(8.47411685331421,-3.99923586314651,13.2779763550341));
#83018=CARTESIAN_POINT('Ctrl Pts',(8.45075800260977,-4.0483617837587,13.2770435148628));
#83019=CARTESIAN_POINT('Ctrl Pts',(8.40842491531257,-4.13542921196689,13.2753929619564));
#83020=CARTESIAN_POINT('Ctrl Pts',(8.38961837023935,-4.17345036231935,13.2746732980573));
#83021=CARTESIAN_POINT('Ctrl Pts',(8.34160660844577,-4.26887956262941,13.272869088469));
#83022=CARTESIAN_POINT('Ctrl Pts',(8.31206643884393,-4.32611662748276,13.2717886359332));
#83023=CARTESIAN_POINT('Ctrl Pts',(8.26192182652364,-4.42086688117238,13.2699994655871));
#83024=CARTESIAN_POINT('Ctrl Pts',(8.24164632175286,-4.45855157669259,13.2692877106335));
#83025=CARTESIAN_POINT('Ctrl Pts',(8.09578006991762,-4.72526807249007,13.2642450766829));
#83026=CARTESIAN_POINT('Ctrl Pts',(7.96091869776515,-4.94909966143834,13.25998285017));
#83027=CARTESIAN_POINT('Ctrl Pts',(7.68297386424863,-5.36958741986179,13.2517125645945));
#83028=CARTESIAN_POINT('Ctrl Pts',(7.54124098901064,-5.56688784775669,13.2477110441061));
#83029=CARTESIAN_POINT('Ctrl Pts',(7.33258708968269,-5.83473218891323,13.242034929786));
#83030=CARTESIAN_POINT('Ctrl Pts',(7.27199246496761,-5.91008110564837,13.2404100563124));
#83031=CARTESIAN_POINT('Ctrl Pts',(7.15987037501171,-6.04516847618693,13.2374423712309));
#83032=CARTESIAN_POINT('Ctrl Pts',(7.10873384052372,-6.10521980304239,13.2361028862485));
#83033=CARTESIAN_POINT('Ctrl Pts',(6.99182560121766,-6.23904858616611,13.2330706805898));
#83034=CARTESIAN_POINT('Ctrl Pts',(6.92563248994424,-6.31244540951852,13.2313745126429));
#83035=CARTESIAN_POINT('Ctrl Pts',(6.81827461710172,-6.42776518121584,13.2286559160603));
#83036=CARTESIAN_POINT('Ctrl Pts',(6.77785520908137,-6.47037191601856,13.2276394580657));
#83037=CARTESIAN_POINT('Ctrl Pts',(6.67880844333969,-6.57283210868215,13.2251660589487));
#83038=CARTESIAN_POINT('Ctrl Pts',(6.61977372892985,-6.63228466667112,13.2237062771434));
#83039=CARTESIAN_POINT('Ctrl Pts',(6.3444963603943,-6.90217296165201,13.2169691272194));
#83040=CARTESIAN_POINT('Ctrl Pts',(6.11896635179262,-7.10287800087862,13.2116373767196));
#83041=CARTESIAN_POINT('Ctrl Pts',(5.78715224157288,-7.37061649434051,13.2041818518444));
#83042=CARTESIAN_POINT('Ctrl Pts',(5.68860472919086,-7.44693862932104,13.2020136427525));
#83043=CARTESIAN_POINT('Ctrl Pts',(5.54678927775254,-7.55231238636502,13.1989727352766));
#83044=CARTESIAN_POINT('Ctrl Pts',(5.50475662497567,-7.58300390274411,13.1980810716903));
#83045=CARTESIAN_POINT('Ctrl Pts',(5.42763000836478,-7.63834119975101,13.1964639964031));
#83046=CARTESIAN_POINT('Ctrl Pts',(5.39261849500465,-7.66309921355812,13.1957371451792));
#83047=CARTESIAN_POINT('Ctrl Pts',(5.30110525512929,-7.72687405946329,13.1938548665736));
#83048=CARTESIAN_POINT('Ctrl Pts',(5.24434236902495,-7.76551175430718,13.1927044141857));
#83049=CARTESIAN_POINT('Ctrl Pts',(5.11277454421888,-7.85296756324806,13.1900711366269));
#83050=CARTESIAN_POINT('Ctrl Pts',(5.03768591250549,-7.90134696016396,13.1885925578243));
#83051=CARTESIAN_POINT('Ctrl Pts',(4.74758360898969,-8.0824424134982,13.182953220033));
#83052=CARTESIAN_POINT('Ctrl Pts',(4.52792604785014,-8.20751555069617,13.1788319096193));
#83053=CARTESIAN_POINT('Ctrl Pts',(4.12193316203394,-8.4174237759249,13.1713178799442));
#83054=CARTESIAN_POINT('Ctrl Pts',(3.93736170677208,-8.50532412339891,13.1679390964062));
#83055=CARTESIAN_POINT('Ctrl Pts',(3.66387530964422,-8.62475785530703,13.1629457176721));
#83056=CARTESIAN_POINT('Ctrl Pts',(3.57712459516057,-8.66109750112375,13.1613639165582));
#83057=CARTESIAN_POINT('Ctrl Pts',(3.41653627533654,-8.72554319548189,13.1584369949076));
#83058=CARTESIAN_POINT('Ctrl Pts',(3.34286192067799,-8.75403326029941,13.1570946686814));
#83059=CARTESIAN_POINT('Ctrl Pts',(3.17320524220403,-8.81718583374221,13.1540037271484));
#83060=CARTESIAN_POINT('Ctrl Pts',(3.07699929109938,-8.85121871992185,13.1522510454903));
#83061=CARTESIAN_POINT('Ctrl Pts',(2.9218029982917,-8.90328331038958,13.1494239748187));
#83062=CARTESIAN_POINT('Ctrl Pts',(2.86315704662275,-8.92231574079415,13.1483557636404));
#83063=CARTESIAN_POINT('Ctrl Pts',(2.64070284205451,-8.99208988836369,13.1443050305917));
#83064=CARTESIAN_POINT('Ctrl Pts',(2.47570039370991,-9.03891029960496,13.141302218957));
#83065=CARTESIAN_POINT('Ctrl Pts',(2.0090424774951,-9.15758980948017,13.1328448263403));
#83066=CARTESIAN_POINT('Ctrl Pts',(1.70497090449188,-9.21904427436467,13.127369764697));
#83067=CARTESIAN_POINT('Ctrl Pts',(1.34549468835034,-9.2733000237612,13.1210944567717));
#83068=CARTESIAN_POINT('Ctrl Pts',(1.29250805154037,-9.28083359619497,13.1201746583157));
#83069=CARTESIAN_POINT('Ctrl Pts',(1.19741911663357,-9.29352308917012,13.1185349478401));
#83070=CARTESIAN_POINT('Ctrl Pts',(1.15534091009123,-9.2988478506439,13.117813276403));
#83071=CARTESIAN_POINT('Ctrl Pts',(1.05918668209728,-9.31035288735936,13.1161734934029));
#83072=CARTESIAN_POINT('Ctrl Pts',(1.00509017404632,-9.31634805462525,13.1152573994326));
#83073=CARTESIAN_POINT('Ctrl Pts',(0.794547377858548,-9.33782598410069,
13.111712140444));
#83074=CARTESIAN_POINT('Ctrl Pts',(0.6377730940271,-9.34984199877075,13.1091151211794));
#83075=CARTESIAN_POINT('Ctrl Pts',(0.15508990447036,-9.37464026168652,13.1011678181589));
#83076=CARTESIAN_POINT('Ctrl Pts',(-0.171241853759035,-9.37435914366116,
13.09585555272));
#83077=CARTESIAN_POINT('Ctrl Pts',(-0.632409571113196,-9.34986949561738,
13.0882012423772));
#83078=CARTESIAN_POINT('Ctrl Pts',(-0.767752975622561,-9.33973001090355,
13.085938121223));
#83079=CARTESIAN_POINT('Ctrl Pts',(-0.985637489753486,-9.31863860542893,
13.0822578279393));
#83080=CARTESIAN_POINT('Ctrl Pts',(-1.06833635235231,-9.30952007996978,
13.0808523939818));
#83081=CARTESIAN_POINT('Ctrl Pts',(-1.23309690467648,-9.28912893962376,
13.0780336943179));
#83082=CARTESIAN_POINT('Ctrl Pts',(-1.31515251543884,-9.27786711780006,
13.0766206171028));
#83083=CARTESIAN_POINT('Ctrl Pts',(-1.52873209547759,-9.24566375107585,
13.0729176005749));
#83084=CARTESIAN_POINT('Ctrl Pts',(-1.65997771398991,-9.22300351609862,
13.0706171122036));
#83085=CARTESIAN_POINT('Ctrl Pts',(-1.96447316743057,-9.16372051266204,
13.0652249817773));
#83086=CARTESIAN_POINT('Ctrl Pts',(-2.13725681400388,-9.12496912538269,
13.0621230880308));
#83087=CARTESIAN_POINT('Ctrl Pts',(-2.60195739059717,-9.00682381242067,
13.0536988860746));
#83088=CARTESIAN_POINT('Ctrl Pts',(-2.89129678421748,-8.91815343809958,
13.0483609096829));
#83089=CARTESIAN_POINT('Ctrl Pts',(-3.22516296886264,-8.79787800074208,
13.0422380548354));
#83090=CARTESIAN_POINT('Ctrl Pts',(-3.27433557615743,-8.77969589689867,
13.0413374050691));
#83091=CARTESIAN_POINT('Ctrl Pts',(-3.36289610044361,-8.74610219057587,
13.0397189759948));
#83092=CARTESIAN_POINT('Ctrl Pts',(-3.4023371009814,-8.73083478126839,13.038999623827));
#83093=CARTESIAN_POINT('Ctrl Pts',(-3.49325666819293,-8.69493063056182,
13.0373449283989));
#83094=CARTESIAN_POINT('Ctrl Pts',(-3.54465796816425,-8.67410287741465,
13.0364118238669));
#83095=CARTESIAN_POINT('Ctrl Pts',(-3.75447803791881,-8.58690749041558,
13.0326072193572));
#83096=CARTESIAN_POINT('Ctrl Pts',(-3.91124293509302,-8.51664632560923,
13.029774266869));
#83097=CARTESIAN_POINT('Ctrl Pts',(-4.41159463152439,-8.27566123374181,
13.0206513555163));
#83098=CARTESIAN_POINT('Ctrl Pts',(-4.74665250849149,-8.08814107561432,
13.0144016021705));
#83099=CARTESIAN_POINT('Ctrl Pts',(-5.15395694547843,-7.82613901459014,
13.0063149420751));
#83100=CARTESIAN_POINT('Ctrl Pts',(-5.2377582367167,-7.77030325407255,13.0046245402432));
#83101=CARTESIAN_POINT('Ctrl Pts',(-5.38560970812548,-7.66831286297231,
13.001590759307));
#83102=CARTESIAN_POINT('Ctrl Pts',(-5.45000732781649,-7.62267893760626,
13.000251503766));
#83103=CARTESIAN_POINT('Ctrl Pts',(-5.59070029913252,-7.52028565004488,
12.9972847648431));
#83104=CARTESIAN_POINT('Ctrl Pts',(-5.6667237002757,-7.46316746026565,12.9956545645022));
#83105=CARTESIAN_POINT('Ctrl Pts',(-5.94010496518926,-7.25118381433151,
12.9896923591598));
#83106=CARTESIAN_POINT('Ctrl Pts',(-6.13209185138352,-7.08956715082722,
12.9853089005774));
#83107=CARTESIAN_POINT('Ctrl Pts',(-6.5491797400863,-6.70882635959014,12.9753902718138));
#83108=CARTESIAN_POINT('Ctrl Pts',(-6.7702188440969,-6.48569529935909,12.9698463124284));
#83109=CARTESIAN_POINT('Ctrl Pts',(-7.01474859725542,-6.21270115495295,
12.9635223486083));
#83110=CARTESIAN_POINT('Ctrl Pts',(-7.04952377421502,-6.17321375751872,
12.9626183578704));
#83111=CARTESIAN_POINT('Ctrl Pts',(-7.11166009930628,-6.10144785663763,
12.9609962510237));
#83112=CARTESIAN_POINT('Ctrl Pts',(-7.13913864378171,-6.06927300067393,
12.9602765293121));
#83113=CARTESIAN_POINT('Ctrl Pts',(-7.19269167513335,-6.00570038276606,
12.9588693898657));
#83114=CARTESIAN_POINT('Ctrl Pts',(-7.21878072655044,-5.97431631660935,
12.9581815993275));
#83115=CARTESIAN_POINT('Ctrl Pts',(-7.28064058040269,-5.89890461516016,
12.9565439995588));
#83116=CARTESIAN_POINT('Ctrl Pts',(-7.3162182622989,-5.85472059752223,12.9555966355733));
#83117=CARTESIAN_POINT('Ctrl Pts',(-7.41600621310316,-5.72846360879097,
12.9529197627028));
#83118=CARTESIAN_POINT('Ctrl Pts',(-7.47925174568263,-5.64563874710119,
12.9511993836763));
#83119=CARTESIAN_POINT('Ctrl Pts',(-7.77145333516526,-5.24944836914489,
12.9430999503543));
#83120=CARTESIAN_POINT('Ctrl Pts',(-7.98217777109818,-4.92311219068823,
12.9367885478748));
#83121=CARTESIAN_POINT('Ctrl Pts',(-8.22462584507596,-4.49095284698223,
12.9285329196642));
#83122=CARTESIAN_POINT('Ctrl Pts',(-8.27557684785323,-4.39635707418454,
12.9267330607153));
#83123=CARTESIAN_POINT('Ctrl Pts',(-8.36077921373284,-4.23143827232256,
12.9236031074117));
#83124=CARTESIAN_POINT('Ctrl Pts',(-8.39579763103608,-4.16152388187751,
12.9222786570999));
#83125=CARTESIAN_POINT('Ctrl Pts',(-8.46505390344619,-4.01882029167887,
12.9195791303703));
#83126=CARTESIAN_POINT('Ctrl Pts',(-8.4992377913579,-3.94601204453747,12.918203800745));
#83127=CARTESIAN_POINT('Ctrl Pts',(-8.57016498219457,-3.78974549753141,
12.9152558493934));
#83128=CARTESIAN_POINT('Ctrl Pts',(-8.60663598511223,-3.70617265250556,
12.9136815698809));
#83129=CARTESIAN_POINT('Ctrl Pts',(-8.67261252243909,-3.54875999022363,
12.9107214972547));
#83130=CARTESIAN_POINT('Ctrl Pts',(-8.70240922746164,-3.4750509412293,12.9093375195691));
#83131=CARTESIAN_POINT('Ctrl Pts',(-8.82893292208684,-3.15022853642411,
12.9032509199261));
#83132=CARTESIAN_POINT('Ctrl Pts',(-8.9157549222299,-2.89539463019322,12.8985039438546));
#83133=CARTESIAN_POINT('Ctrl Pts',(-9.03709174969183,-2.48169550405554,
12.8909421878323));
#83134=CARTESIAN_POINT('Ctrl Pts',(-9.07865412938785,-2.32505469080471,
12.8881123461397));
#83135=CARTESIAN_POINT('Ctrl Pts',(-9.12874984060905,-2.11435242857279,
12.8843797880283));
#83136=CARTESIAN_POINT('Ctrl Pts',(-9.140902234698,-2.0611807777376,12.8834441404231));
#83137=CARTESIAN_POINT('Ctrl Pts',(-9.16073828440998,-1.97076258804941,
12.8818654108044));
#83138=CARTESIAN_POINT('Ctrl Pts',(-9.16866064140778,-1.93357005070896,
12.88121965639));
#83139=CARTESIAN_POINT('Ctrl Pts',(-9.18485258293491,-1.85521711875724,
12.8798666610249));
#83140=CARTESIAN_POINT('Ctrl Pts',(-9.19307236590699,-1.81404741159164,
12.8791599214581));
#83141=CARTESIAN_POINT('Ctrl Pts',(-9.21241883691012,-1.71363857649148,
12.8774450081386));
#83142=CARTESIAN_POINT('Ctrl Pts',(-9.22325115943001,-1.65434460348244,
12.8764397023883));
#83143=CARTESIAN_POINT('Ctrl Pts',(-9.2532452330598,-1.48070244117914,12.8735125096194));
#83144=CARTESIAN_POINT('Ctrl Pts',(-9.27085773806322,-1.36609807419211,
12.8716017353241));
#83145=CARTESIAN_POINT('Ctrl Pts',(-9.33095789351405,-0.920036641902406,
12.8642063249432));
#83146=CARTESIAN_POINT('Ctrl Pts',(-9.3578305814888,-0.586727814351847,
12.8587604154233));
#83147=CARTESIAN_POINT('Ctrl Pts',(-9.3691130617853,-0.168514986455563,
12.8518128918622));
#83148=CARTESIAN_POINT('Ctrl Pts',(-9.3702491589803,-0.0843061205128449,
12.8504087881159));
#83149=CARTESIAN_POINT('Ctrl Pts',(-9.37024999953324,-9.35274742388515E-5,
12.8489979277639));
#83150=CARTESIAN_POINT('Ctrl Pts',(-9.37024999953368,-9.34831142609071E-5,
12.8489979270207));
#83151=CARTESIAN_POINT('Ctrl Pts',(-9.37025068795026,0.0689097317925185,
12.8478418778276));
#83152=CARTESIAN_POINT('Ctrl Pts',(-9.36948915928981,0.13791078196804,12.8466813796634));
#83153=CARTESIAN_POINT('Ctrl Pts',(-9.36645008943694,0.275514971673631,
12.8443569913286));
#83154=CARTESIAN_POINT('Ctrl Pts',(-9.36418075739126,0.344114077532216,
12.8431932232752));
#83155=CARTESIAN_POINT('Ctrl Pts',(-9.35719707657167,0.502529865745441,
12.8404934081459));
#83156=CARTESIAN_POINT('Ctrl Pts',(-9.35194285634548,0.592315927649199,
12.8389540316959));
#83157=CARTESIAN_POINT('Ctrl Pts',(-9.33251077801821,0.858587506071259,
12.8343610783562));
#83158=CARTESIAN_POINT('Ctrl Pts',(-9.31462281536421,1.03476152411561,12.8312853539796));
#83159=CARTESIAN_POINT('Ctrl Pts',(-9.24801550851545,1.54611188847006,12.8222692063276));
#83160=CARTESIAN_POINT('Ctrl Pts',(-9.18610627931292,1.87928272811455,12.8162752902034));
#83161=CARTESIAN_POINT('Ctrl Pts',(-9.08511188705283,2.2957371633505,12.8088138303866));
#83162=CARTESIAN_POINT('Ctrl Pts',(-9.06266800784841,2.38279578757585,12.8072564536651));
#83163=CARTESIAN_POINT('Ctrl Pts',(-9.02834732016025,2.50841699045259,12.805018757162));
#83164=CARTESIAN_POINT('Ctrl Pts',(-9.01746883241015,2.54724694437324,12.8043284122212));
#83165=CARTESIAN_POINT('Ctrl Pts',(-8.99460288295917,2.62688270505295,12.802916184013));
#83166=CARTESIAN_POINT('Ctrl Pts',(-8.98258761326947,2.66767942945808,12.8021948252546));
#83167=CARTESIAN_POINT('Ctrl Pts',(-8.95457446358068,2.76045998732238,12.8005583708945));
#83168=CARTESIAN_POINT('Ctrl Pts',(-8.93840088449609,2.81238916414691,12.7996452392358));
#83169=CARTESIAN_POINT('Ctrl Pts',(-8.83539783251091,3.13323907016311,12.7940130163272));
#83170=CARTESIAN_POINT('Ctrl Pts',(-8.73689171841284,3.39825930246818,12.7893985545897));
#83171=CARTESIAN_POINT('Ctrl Pts',(-8.51914741384282,3.91170031804821,12.7802548303991));
#83172=CARTESIAN_POINT('Ctrl Pts',(-8.40063319704573,4.16012419588458,12.7757308071256));
#83173=CARTESIAN_POINT('Ctrl Pts',(-8.23478779205425,4.47167902837219,12.7698290285569));
#83174=CARTESIAN_POINT('Ctrl Pts',(-8.19735952861368,4.53992731674847,12.7685219947654));
#83175=CARTESIAN_POINT('Ctrl Pts',(-8.13014546214521,4.65894660077353,12.7662159730845));
#83176=CARTESIAN_POINT('Ctrl Pts',(-8.10072343900325,4.70991809009699,12.7652196566524));
#83177=CARTESIAN_POINT('Ctrl Pts',(-8.02810698053066,4.83302725600549,12.7627913962187));
#83178=CARTESIAN_POINT('Ctrl Pts',(-7.98441805263359,4.90486722229292,12.7613558627459));
#83179=CARTESIAN_POINT('Ctrl Pts',(-7.8676074262543,5.09124763279602,12.7575820106739));
#83180=CARTESIAN_POINT('Ctrl Pts',(-7.79295076391193,5.20480233121666,12.7552326984802));
#83181=CARTESIAN_POINT('Ctrl Pts',(-7.52382022283719,5.59537805712278,12.7469812473793));
#83182=CARTESIAN_POINT('Ctrl Pts',(-7.31683180453062,5.86345438910015,12.7410005236719));
#83183=CARTESIAN_POINT('Ctrl Pts',(-7.03063885861127,6.19529303366789,12.7333255214571));
#83184=CARTESIAN_POINT('Ctrl Pts',(-6.96427807975564,6.26979819611523,12.7315840841177));
#83185=CARTESIAN_POINT('Ctrl Pts',(-6.88863653807405,6.35204022389922,12.7296468582307));
#83186=CARTESIAN_POINT('Ctrl Pts',(-6.88051605684362,6.36083541300986,12.7294394919915));
#83187=CARTESIAN_POINT('Ctrl Pts',(-6.86773833749641,6.37462169782446,12.7291141596582));
#83188=CARTESIAN_POINT('Ctrl Pts',(-6.86309246289031,6.37962330459454,12.7289960703085));
#83189=CARTESIAN_POINT('Ctrl Pts',(-6.85336239926296,6.39007546467776,12.7287491697594));
#83190=CARTESIAN_POINT('Ctrl Pts',(-6.84827716374798,6.39552503774588,12.7286203704845));
#83191=CARTESIAN_POINT('Ctrl Pts',(-6.83908434605188,6.40535294984171,12.7283879687194));
#83192=CARTESIAN_POINT('Ctrl Pts',(-6.83497904844297,6.409733419716,12.7282843395184));
#83193=CARTESIAN_POINT('Ctrl Pts',(-6.82755388256784,6.41764103899447,12.728097191415));
#83194=CARTESIAN_POINT('Ctrl Pts',(-6.82423548397376,6.42116956512113,12.7280136547766));
#83195=CARTESIAN_POINT('Ctrl Pts',(-6.81822653213817,6.42754909636868,12.727862572655));
#83196=CARTESIAN_POINT('Ctrl Pts',(-6.81553692308385,6.43040098904178,12.7277950154882));
#83197=CARTESIAN_POINT('Ctrl Pts',(-6.8106589097118,6.43556682985437,12.7276726127832));
#83198=CARTESIAN_POINT('Ctrl Pts',(-6.80847111389313,6.43788135159733,12.7276177595633));
#83199=CARTESIAN_POINT('Ctrl Pts',(-6.80449613629775,6.44208228340539,12.727518178698));
#83200=CARTESIAN_POINT('Ctrl Pts',(-6.80270934908332,6.44396906626288,12.7274734459909));
#83201=CARTESIAN_POINT('Ctrl Pts',(-6.79945695108753,6.44740062095882,12.7273920756374));
#83202=CARTESIAN_POINT('Ctrl Pts',(-6.7979915981891,6.44894563690718,12.7273554346395));
#83203=CARTESIAN_POINT('Ctrl Pts',(-6.79531943581326,6.45176114702816,12.7272886541176));
#83204=CARTESIAN_POINT('Ctrl Pts',(-6.79411279639709,6.45303180240709,12.7272585123605));
#83205=CARTESIAN_POINT('Ctrl Pts',(-6.79190861199632,6.4553516220754,12.7272034768958));
#83206=CARTESIAN_POINT('Ctrl Pts',(-6.79091118017791,6.45640089378566,12.7271785816891));
#83207=CARTESIAN_POINT('Ctrl Pts',(-6.78908624261721,6.45831978875433,12.7271330495524));
#83208=CARTESIAN_POINT('Ctrl Pts',(-6.78825881287262,6.45918948421297,12.7271124116087));
#83209=CARTESIAN_POINT('Ctrl Pts',(-6.78674271439468,6.46078241302412,12.7270746084777));
#83210=CARTESIAN_POINT('Ctrl Pts',(-6.7860540971278,6.46150569532258,12.7270574425997));
#83211=CARTESIAN_POINT('Ctrl Pts',(-6.78479069749854,6.46283226983135,12.727025956674));
#83212=CARTESIAN_POINT('Ctrl Pts',(-6.78421595026531,6.46343559548651,12.7270116361522));
#83213=CARTESIAN_POINT('Ctrl Pts',(-6.783160244788,6.46454349834128,12.7269853376597));
#83214=CARTESIAN_POINT('Ctrl Pts',(-6.78267931071224,6.46504809854151,12.7269733593619));
#83215=CARTESIAN_POINT('Ctrl Pts',(-6.78048266630905,6.46735232198527,12.7269186589345));
#83216=CARTESIAN_POINT('Ctrl Pts',(-6.77876629592429,6.46915131605748,12.7268759457779));
#83217=CARTESIAN_POINT('Ctrl Pts',(-6.77544051880157,6.47263441460103,12.7267932349078));
#83218=CARTESIAN_POINT('Ctrl Pts',(-6.77383119971992,6.47431860249386,12.7267532359936));
#83219=CARTESIAN_POINT('Ctrl Pts',(-6.77070781143242,6.4775848578038,12.7266756527707));
#83220=CARTESIAN_POINT('Ctrl Pts',(-6.76919381534365,6.47916699492733,12.7266380674492));
#83221=CARTESIAN_POINT('Ctrl Pts',(-6.76625039196162,6.48224073634446,12.7265650381346));
#83222=CARTESIAN_POINT('Ctrl Pts',(-6.76482102572094,6.48373239890491,12.7265295932876));
#83223=CARTESIAN_POINT('Ctrl Pts',(-6.74383561979175,6.50561792176144,12.7260094878117));
#83224=CARTESIAN_POINT('Ctrl Pts',(-6.72418791086855,6.5259237164346,12.7255261302429));
#83225=CARTESIAN_POINT('Ctrl Pts',(-6.67491057299716,6.57639275062133,12.7243231318315));
#83226=CARTESIAN_POINT('Ctrl Pts',(-6.64516820719732,6.60644475262474,12.7236054847017));
#83227=CARTESIAN_POINT('Ctrl Pts',(-6.57817743453521,6.67322281916118,12.7220073445606));
#83228=CARTESIAN_POINT('Ctrl Pts',(-6.54082293949006,6.70984026964447,12.7211284594741));
#83229=CARTESIAN_POINT('Ctrl Pts',(-6.27623946923494,6.96489410060998,12.7149808490458));
#83230=CARTESIAN_POINT('Ctrl Pts',(-6.03842135734806,7.17205695632022,12.7098457561277));
#83231=CARTESIAN_POINT('Ctrl Pts',(-5.65671499568797,7.47209260172947,12.7018802957643));
#83232=CARTESIAN_POINT('Ctrl Pts',(-5.51996942592922,7.57367346626392,12.6990784672235));
#83233=CARTESIAN_POINT('Ctrl Pts',(-5.33027186584697,7.70672145381521,12.6952344702456));
#83234=CARTESIAN_POINT('Ctrl Pts',(-5.27966683229501,7.74147736919135,12.6942131041715));
#83235=CARTESIAN_POINT('Ctrl Pts',(-5.14428730960835,7.83251214534628,12.6914898236771));
#83236=CARTESIAN_POINT('Ctrl Pts',(-5.05893157485354,7.88791161746215,12.6897820997537));
#83237=CARTESIAN_POINT('Ctrl Pts',(-4.90575605715464,7.98381984146777,12.6867302367064));
#83238=CARTESIAN_POINT('Ctrl Pts',(-4.83829437248597,8.02488188603704,12.685390431205));
#83239=CARTESIAN_POINT('Ctrl Pts',(-4.68918771397459,8.11307520800644,12.6824374364602));
#83240=CARTESIAN_POINT('Ctrl Pts',(-4.60733425417488,8.15983711612044,12.6808216929367));
#83241=CARTESIAN_POINT('Ctrl Pts',(-4.18131940413554,8.39476019069,12.6724393018009));
#83242=CARTESIAN_POINT('Ctrl Pts',(-3.82629694868124,8.56241082020753,12.6655246390163));
#83243=CARTESIAN_POINT('Ctrl Pts',(-3.29433056417342,8.77390778054548,12.6554743066057));
#83244=CARTESIAN_POINT('Ctrl Pts',(-3.12495517088969,8.83565091517452,12.652321438248));
#83245=CARTESIAN_POINT('Ctrl Pts',(-2.90079579789922,8.91011226362078,12.6482492252726));
#83246=CARTESIAN_POINT('Ctrl Pts',(-2.84753014880143,8.92727779799855,12.6472889543156));
#83247=CARTESIAN_POINT('Ctrl Pts',(-2.75378773997722,8.95656312711505,12.6456137856883));
#83248=CARTESIAN_POINT('Ctrl Pts',(-2.71337704906949,8.96888816747332,12.6448966074594));
#83249=CARTESIAN_POINT('Ctrl Pts',(-2.61331199889471,8.99866927085689,12.6431324490398));
#83250=CARTESIAN_POINT('Ctrl Pts',(-2.55356478393201,9.01580585248389,12.6420890996788));
#83251=CARTESIAN_POINT('Ctrl Pts',(-2.2428860759334,9.1015780689023,12.6367059270095));
#83252=CARTESIAN_POINT('Ctrl Pts',(-1.98934548662513,9.16033660958113,12.6324515687093));
#83253=CARTESIAN_POINT('Ctrl Pts',(-1.44765654606138,9.26232097921423,12.6234165312014));
#83254=CARTESIAN_POINT('Ctrl Pts',(-1.15927120322874,9.30281618959144,12.6186366857865));
#83255=CARTESIAN_POINT('Ctrl Pts',(-0.773104579368081,9.33880406983154,
12.6121530474745));
#83256=CARTESIAN_POINT('Ctrl Pts',(-0.67660526437447,9.34629110413154,12.6105265685955));
#83257=CARTESIAN_POINT('Ctrl Pts',(-0.501289393057884,9.35716379971669,
12.6075573165885));
#83258=CARTESIAN_POINT('Ctrl Pts',(-0.422512941165264,9.36105166160757,
12.6062178897357));
#83259=CARTESIAN_POINT('Ctrl Pts',(-0.245039371129517,9.36756570265129,
12.6031875938936));
#83260=CARTESIAN_POINT('Ctrl Pts',(-0.146330940901112,9.36962745675422,
12.6014932981909));
#83261=CARTESIAN_POINT('Ctrl Pts',(0.356140373736641,9.37218045634467,12.5928234976521));
#83262=CARTESIAN_POINT('Ctrl Pts',(0.759598769324292,9.34813397349099,12.5856932237886));
#83263=CARTESIAN_POINT('Ctrl Pts',(1.31811063074986,9.27844168522384,12.5758234835243));
#83264=CARTESIAN_POINT('Ctrl Pts',(1.4754527460543,9.25472501895612,12.5730460091534));
#83265=CARTESIAN_POINT('Ctrl Pts',(1.68585375626433,9.21750836184417,12.5693643964998));
#83266=CARTESIAN_POINT('Ctrl Pts',(1.73950867985349,9.20753348401263,12.5684284459436));
#83267=CARTESIAN_POINT('Ctrl Pts',(1.83468370863912,9.18897807017679,12.5667751820613));
#83268=CARTESIAN_POINT('Ctrl Pts',(1.87623821958174,9.18058344714477,12.5660558813679));
#83269=CARTESIAN_POINT('Ctrl Pts',(1.96996115498921,9.160987117938,12.564438651363));
#83270=CARTESIAN_POINT('Ctrl Pts',(2.02209362602352,9.14962126599199,12.5635425113279));
#83271=CARTESIAN_POINT('Ctrl Pts',(2.37715871531596,9.06902758353891,12.5574545000721));
#83272=CARTESIAN_POINT('Ctrl Pts',(2.67658333092039,8.98521275253325,12.5523907831215));
#83273=CARTESIAN_POINT('Ctrl Pts',(3.13376318343708,8.83235313510846,12.5444824385657));
#83274=CARTESIAN_POINT('Ctrl Pts',(3.2947156829486,8.773584330605,12.5416645053969));
#83275=CARTESIAN_POINT('Ctrl Pts',(3.51124418559039,8.68772386550307,12.5378004817293));
#83276=CARTESIAN_POINT('Ctrl Pts',(3.56829672573757,8.66444690434702,12.536775412961));
#83277=CARTESIAN_POINT('Ctrl Pts',(3.71917235501035,8.60114794219391,12.5340443878932));
#83278=CARTESIAN_POINT('Ctrl Pts',(3.81257846468535,8.56015387204622,12.5323326090934));
#83279=CARTESIAN_POINT('Ctrl Pts',(3.97709530717437,8.48472372760624,12.529276483005));
#83280=CARTESIAN_POINT('Ctrl Pts',(4.04847489125391,8.45089787166887,12.5279365185356));
#83281=CARTESIAN_POINT('Ctrl Pts',(4.17688098086435,8.38804765013894,12.5254996843973));
#83282=CARTESIAN_POINT('Ctrl Pts',(4.23405345369067,8.35933425819504,12.5244050892833));
#83283=CARTESIAN_POINT('Ctrl Pts',(4.290926628303,8.33003803911004,12.5233065119449));
#83284=CARTESIAN_POINT('Ctrl Pts',(4.29092662693973,8.33003803981228,12.3256242449617));
#83285=CARTESIAN_POINT('Ctrl Pts',(4.10018693584926,8.42829089476957,12.3293916132614));
#83286=CARTESIAN_POINT('Ctrl Pts',(3.90612200113809,8.51996701307972,12.3331737430698));
#83287=CARTESIAN_POINT('Ctrl Pts',(3.65267042137266,8.62921527930986,12.3379988945992));
#83288=CARTESIAN_POINT('Ctrl Pts',(3.59602888310997,8.65297254301987,12.3390699215654));
#83289=CARTESIAN_POINT('Ctrl Pts',(3.50246379508337,8.69113933399208,12.3408251808568));
#83290=CARTESIAN_POINT('Ctrl Pts',(3.465675147465,8.70587453023978,12.341511809104));
#83291=CARTESIAN_POINT('Ctrl Pts',(3.37198635540229,8.74271234330628,12.3432506201701));
#83292=CARTESIAN_POINT('Ctrl Pts',(3.31496160327234,8.76449317941675,12.3442998345609));
#83293=CARTESIAN_POINT('Ctrl Pts',(3.21816935841031,8.80038357627886,12.3460630149162));
#83294=CARTESIAN_POINT('Ctrl Pts',(3.1785121382877,8.81478449590424,12.3467803051359));
#83295=CARTESIAN_POINT('Ctrl Pts',(3.08617057416272,8.84761274560848,12.3484385798004));
#83296=CARTESIAN_POINT('Ctrl Pts',(3.03341627330563,8.86583813529258,12.3493772464112));
#83297=CARTESIAN_POINT('Ctrl Pts',(2.81872121646125,8.93786971398334,12.3531676549845));
#83298=CARTESIAN_POINT('Ctrl Pts',(2.65548716333115,8.98771898657934,12.3559818463684));
#83299=CARTESIAN_POINT('Ctrl Pts',(2.41796575284859,9.05321841104248,12.3600290138679));
#83300=CARTESIAN_POINT('Ctrl Pts',(2.34470724966143,9.07246768528441,12.3612707179495));
#83301=CARTESIAN_POINT('Ctrl Pts',(2.06588739233299,9.14212715791704,12.3659813008466));
#83302=CARTESIAN_POINT('Ctrl Pts',(1.85887235999473,9.18645595886654,12.3694487713326));
#83303=CARTESIAN_POINT('Ctrl Pts',(1.58162114140453,9.23606846910573,12.3741086040337));
#83304=CARTESIAN_POINT('Ctrl Pts',(1.51257168796278,9.24762742935078,12.3752702779839));
#83305=CARTESIAN_POINT('Ctrl Pts',(1.33378496775185,9.27550052830089,12.3782837637686));
#83306=CARTESIAN_POINT('Ctrl Pts',(1.22387605106547,9.2906415127309,12.3801418237822));
#83307=CARTESIAN_POINT('Ctrl Pts',(1.0345210397253,9.31330845353266,12.3833573270572));
#83308=CARTESIAN_POINT('Ctrl Pts',(0.955199923120752,9.32177779206421,12.3847085871674));
#83309=CARTESIAN_POINT('Ctrl Pts',(0.787122701057217,9.33755601762871,12.3875820708725));
#83310=CARTESIAN_POINT('Ctrl Pts',(0.698350956302175,9.34461451440436,12.389105761754));
#83311=CARTESIAN_POINT('Ctrl Pts',(0.431346196273203,9.36201881970316,12.3937072643365));
#83312=CARTESIAN_POINT('Ctrl Pts',(0.252905212216841,9.36853748148371,12.3968079771902));
#83313=CARTESIAN_POINT('Ctrl Pts',(0.00740264328893203,9.37048651556237,
12.4011000631563));
#83314=CARTESIAN_POINT('Ctrl Pts',(-0.0595861065972801,9.37029998575161,
12.4022737802285));
#83315=CARTESIAN_POINT('Ctrl Pts',(-0.360700199179532,9.36623236775615,
12.4075579214997));
#83316=CARTESIAN_POINT('Ctrl Pts',(-0.594632414339054,9.35429450392961,
12.4116878511372));
#83317=CARTESIAN_POINT('Ctrl Pts',(-0.888142150973626,9.3282608105357,12.4168383796325));
#83318=CARTESIAN_POINT('Ctrl Pts',(-0.948359976785155,9.32233123195316,
12.4178932766622));
#83319=CARTESIAN_POINT('Ctrl Pts',(-1.04750943995519,9.31159746387329,12.4196252838786));
#83320=CARTESIAN_POINT('Ctrl Pts',(-1.08647583805339,9.30713133110853,12.4203047226472));
#83321=CARTESIAN_POINT('Ctrl Pts',(-1.18557402264217,9.29514236646072,12.4220285930561));
#83322=CARTESIAN_POINT('Ctrl Pts',(-1.24566305324711,9.28728060078173,12.4230700726671));
#83323=CARTESIAN_POINT('Ctrl Pts',(-1.34743361270927,9.27295995436028,12.4248252300336));
#83324=CARTESIAN_POINT('Ctrl Pts',(-1.38915533010638,9.26680155918781,12.4255421422928));
#83325=CARTESIAN_POINT('Ctrl Pts',(-1.48634614085464,9.25178444133653,12.4272060081606));
#83326=CARTESIAN_POINT('Ctrl Pts',(-1.54177985667985,9.24270821201918,12.4281505698583));
#83327=CARTESIAN_POINT('Ctrl Pts',(-1.77991433949845,9.20151619537182,12.4321950481225));
#83328=CARTESIAN_POINT('Ctrl Pts',(-1.96172140641083,9.16447733875931,12.4352500879022));
#83329=CARTESIAN_POINT('Ctrl Pts',(-2.38595017380165,9.06484758045496,12.4424028587785));
#83330=CARTESIAN_POINT('Ctrl Pts',(-2.62720089302723,8.99789060438845,12.4464908829958));
#83331=CARTESIAN_POINT('Ctrl Pts',(-2.97538731318275,8.88605542407084,12.4525307071389));
#83332=CARTESIAN_POINT('Ctrl Pts',(-3.0846318429092,8.8487262913478,12.4544458015077));
#83333=CARTESIAN_POINT('Ctrl Pts',(-3.28818196763926,8.77494502546297,12.4580606397742));
#83334=CARTESIAN_POINT('Ctrl Pts',(-3.38264167823421,8.73896653290437,12.4597572668517));
#83335=CARTESIAN_POINT('Ctrl Pts',(-3.54980692525323,8.67217893350925,12.4627975253513));
#83336=CARTESIAN_POINT('Ctrl Pts',(-3.62274003534073,8.64196570602424,12.4641369577684));
#83337=CARTESIAN_POINT('Ctrl Pts',(-3.78238397439797,8.57345556815873,12.4670986264043));
#83338=CARTESIAN_POINT('Ctrl Pts',(-3.86891307157105,8.53475720195737,12.4687235199776));
#83339=CARTESIAN_POINT('Ctrl Pts',(-4.34430541480735,8.31343226183535,12.4777603550593));
#83340=CARTESIAN_POINT('Ctrl Pts',(-4.720839110414,8.10554250504209,12.4853549651812));
#83341=CARTESIAN_POINT('Ctrl Pts',(-5.20538432107292,7.79276621272657,12.4954593706856));
#83342=CARTESIAN_POINT('Ctrl Pts',(-5.32709854324198,7.71007473970601,12.4980247854707));
#83343=CARTESIAN_POINT('Ctrl Pts',(-5.49040896891864,7.59340929124898,12.5014815291635));
#83344=CARTESIAN_POINT('Ctrl Pts',(-5.53373476161795,7.56189360649492,12.5023999956596));
#83345=CARTESIAN_POINT('Ctrl Pts',(-5.61097929889184,7.50468564582699,12.5040383296582));
#83346=CARTESIAN_POINT('Ctrl Pts',(-5.64499770620132,7.47913071367678,12.5047599721763));
#83347=CARTESIAN_POINT('Ctrl Pts',(-5.72220490318684,7.42030512635671,12.5063988411738));
#83348=CARTESIAN_POINT('Ctrl Pts',(-5.76527975067285,7.38688747281286,12.5073140819593));
#83349=CARTESIAN_POINT('Ctrl Pts',(-6.0410691708539,7.1690470277892,12.5131878210227));
#83350=CARTESIAN_POINT('Ctrl Pts',(-6.26519866683398,6.97402603365502,12.5180309843374));
#83351=CARTESIAN_POINT('Ctrl Pts',(-6.60774895259073,6.64610159922737,12.5258082207553));
#83352=CARTESIAN_POINT('Ctrl Pts',(-6.7323027751634,6.51990121634516,12.5287223046292));
#83353=CARTESIAN_POINT('Ctrl Pts',(-6.94409460980743,6.29276558707732,12.5338716642795));
#83354=CARTESIAN_POINT('Ctrl Pts',(-7.03289761939615,6.19335931646279,12.536095133488));
#83355=CARTESIAN_POINT('Ctrl Pts',(-7.17340675698332,6.02915272654743,12.5397294195011));
#83356=CARTESIAN_POINT('Ctrl Pts',(-7.22642664434636,5.96550123768505,12.5411290887672));
#83357=CARTESIAN_POINT('Ctrl Pts',(-7.33098032339454,5.83654276931601,12.5439483263265));
#83358=CARTESIAN_POINT('Ctrl Pts',(-7.38250239972979,5.77123576703363,12.5453678279671));
#83359=CARTESIAN_POINT('Ctrl Pts',(-7.51570779995777,5.59768768567244,12.5491193757425));
#83360=CARTESIAN_POINT('Ctrl Pts',(-7.59592281972188,5.48834469772859,12.5514625351314));
#83361=CARTESIAN_POINT('Ctrl Pts',(-7.86090650556243,5.11019673058696,12.5594918122024));
#83362=CARTESIAN_POINT('Ctrl Pts',(-8.03400283670296,4.83350379233838,12.565250382179));
#83363=CARTESIAN_POINT('Ctrl Pts',(-8.26869221245894,4.41079021604326,12.5737276883858));
#83364=CARTESIAN_POINT('Ctrl Pts',(-8.34158933103926,4.27132636338498,12.5764740932088));
#83365=CARTESIAN_POINT('Ctrl Pts',(-8.43493433332424,4.08122913472762,12.5801229601713));
#83366=CARTESIAN_POINT('Ctrl Pts',(-8.45850214303701,4.03215698752978,12.5810565283575));
#83367=CARTESIAN_POINT('Ctrl Pts',(-8.49966855575182,3.94449214631311,12.5827077165169));
#83368=CARTESIAN_POINT('Ctrl Pts',(-8.51743519037644,3.90598023921442,12.5834272964882));
#83369=CARTESIAN_POINT('Ctrl Pts',(-8.55702361428688,3.81861165148472,12.5850473179145));
#83370=CARTESIAN_POINT('Ctrl Pts',(-8.57868960430758,3.76968603065122,12.5859459458041));
#83371=CARTESIAN_POINT('Ctrl Pts',(-8.72305585277571,3.43599040955934,12.5920250303003));
#83372=CARTESIAN_POINT('Ctrl Pts',(-8.83197472711547,3.14546619399227,12.5970781241561));
#83373=CARTESIAN_POINT('Ctrl Pts',(-8.97844502858045,2.68672899232054,12.6049781222875));
#83374=CARTESIAN_POINT('Ctrl Pts',(-9.02610672054987,2.52198039704787,12.6077986057257));
#83375=CARTESIAN_POINT('Ctrl Pts',(-9.08472261532293,2.29634516751517,12.6116658000495));
#83376=CARTESIAN_POINT('Ctrl Pts',(-9.09963501140484,2.23652157870451,12.6126914543787));
#83377=CARTESIAN_POINT('Ctrl Pts',(-9.13765780546985,2.07730757723042,12.615423705342));
#83378=CARTESIAN_POINT('Ctrl Pts',(-9.15973691788171,1.97767956659277,12.6171361265439));
#83379=CARTESIAN_POINT('Ctrl Pts',(-9.19601293007418,1.8003250758322,12.620192933027));
#83380=CARTESIAN_POINT('Ctrl Pts',(-9.21086225564588,1.7227421927309,12.6215329277304));
#83381=CARTESIAN_POINT('Ctrl Pts',(-9.24124005282667,1.55238949577581,12.6244824208304));
#83382=CARTESIAN_POINT('Ctrl Pts',(-9.25635621775802,1.45955485492888,12.6260944312275));
#83383=CARTESIAN_POINT('Ctrl Pts',(-9.30000516016737,1.16345070975723,12.6312511241511));
#83384=CARTESIAN_POINT('Ctrl Pts',(-9.32325802937735,0.959464835855618,
12.6348272221993));
#83385=CARTESIAN_POINT('Ctrl Pts',(-9.36009399285118,0.503710460934793,
12.6428416194209));
#83386=CARTESIAN_POINT('Ctrl Pts',(-9.37025445438468,0.251823575469268,
12.6472885537035));
#83387=CARTESIAN_POINT('Ctrl Pts',(-9.37024777945855,-0.125660008993952,
12.6538898603629));
#83388=CARTESIAN_POINT('Ctrl Pts',(-9.36772447063175,-0.251141934044318,
12.6560732124325));
#83389=CARTESIAN_POINT('Ctrl Pts',(-9.36058956714581,-0.428553724362328,
12.6591292337324));
#83390=CARTESIAN_POINT('Ctrl Pts',(-9.35806408724459,-0.48055373735057,
12.6600211776118));
#83391=CARTESIAN_POINT('Ctrl Pts',(-9.35266863418075,-0.575337177688494,
12.6616384666671));
#83392=CARTESIAN_POINT('Ctrl Pts',(-9.34993810082631,-0.618126975254532,
12.6623652549006));
#83393=CARTESIAN_POINT('Ctrl Pts',(-9.34207338985221,-0.729355841125541,
12.6642469254591));
#83394=CARTESIAN_POINT('Ctrl Pts',(-9.3364808253961,-0.797759985463153,
12.6653968396457));
#83395=CARTESIAN_POINT('Ctrl Pts',(-9.32188707556834,-0.954973034984231,
12.668028575662));
#83396=CARTESIAN_POINT('Ctrl Pts',(-9.31236735529,-1.0437271845457,12.6695061581443));
#83397=CARTESIAN_POINT('Ctrl Pts',(-9.27109792347475,-1.38273642558648,
12.6751377293242));
#83398=CARTESIAN_POINT('Ctrl Pts',(-9.23051565711507,-1.63180812299914,
12.6792523619423));
#83399=CARTESIAN_POINT('Ctrl Pts',(-9.13885095435991,-2.07965453734036,
12.6867675659307));
#83400=CARTESIAN_POINT('Ctrl Pts',(-9.09119689265554,-2.27896872641043,
12.6901544577921));
#83401=CARTESIAN_POINT('Ctrl Pts',(-9.01218731680539,-2.56727726220549,
12.6951563606688));
#83402=CARTESIAN_POINT('Ctrl Pts',(-8.98596209643664,-2.65761508153139,
12.6967383725954));
#83403=CARTESIAN_POINT('Ctrl Pts',(-8.93522059776889,-2.823058082827,12.6996654918217));
#83404=CARTESIAN_POINT('Ctrl Pts',(-8.91110604765518,-2.89827759945263,
12.7010078022192));
#83405=CARTESIAN_POINT('Ctrl Pts',(-8.85367091620872,-3.06993573480985,
12.704098435573));
#83406=CARTESIAN_POINT('Ctrl Pts',(-8.81972047407431,-3.16615299646679,
12.7058508216072));
#83407=CARTESIAN_POINT('Ctrl Pts',(-8.76274867611298,-3.31958132814912,
12.7086773215939));
#83408=CARTESIAN_POINT('Ctrl Pts',(-8.74072205927097,-3.37715300566313,
12.7097452587643));
#83409=CARTESIAN_POINT('Ctrl Pts',(-8.65529935627304,-3.5939896555623,12.7137945115269));
#83410=CARTESIAN_POINT('Ctrl Pts',(-8.58810526253273,-3.75172178793961,
12.7167961027377));
#83411=CARTESIAN_POINT('Ctrl Pts',(-8.38721848115428,-4.18956375899621,
12.7252572305336));
#83412=CARTESIAN_POINT('Ctrl Pts',(-8.24388370220131,-4.46500393824816,
12.7307373534822));
#83413=CARTESIAN_POINT('Ctrl Pts',(-8.06014858242053,-4.77895880835748,
12.7370162877287));
#83414=CARTESIAN_POINT('Ctrl Pts',(-8.03275481892451,-4.82486191493164,
12.7379349684493));
#83415=CARTESIAN_POINT('Ctrl Pts',(-7.982927898071,-4.90675508555095,12.7395734257385));
#83416=CARTESIAN_POINT('Ctrl Pts',(-7.96064039456578,-4.94283196374476,
12.740294950886));
#83417=CARTESIAN_POINT('Ctrl Pts',(-7.9091591695063,-5.02491341500588,12.7419355499385));
#83418=CARTESIAN_POINT('Ctrl Pts',(-7.87980761818948,-5.07081704614308,
12.7428525938493));
#83419=CARTESIAN_POINT('Ctrl Pts',(-7.76381515635722,-5.2487813217405,12.7464110358226));
#83420=CARTESIAN_POINT('Ctrl Pts',(-7.67424096165355,-5.37889924499028,
12.7490199785164));
#83421=CARTESIAN_POINT('Ctrl Pts',(-7.38963317210013,-5.77073734565759,
12.7569828281751));
#83422=CARTESIAN_POINT('Ctrl Pts',(-7.18418257138099,-6.02458371304721,
12.762299151219));
#83423=CARTESIAN_POINT('Ctrl Pts',(-6.87555506321372,-6.36761939360104,
12.7699479345883));
#83424=CARTESIAN_POINT('Ctrl Pts',(-6.78304107448008,-6.46607978686093,
12.7722009630794));
#83425=CARTESIAN_POINT('Ctrl Pts',(-6.63022776282626,-6.6218253791488,12.7758695459237));
#83426=CARTESIAN_POINT('Ctrl Pts',(-6.57123807541899,-6.68036837730453,
12.7772735135125));
#83427=CARTESIAN_POINT('Ctrl Pts',(-6.45185741836016,-6.79573358313071,
12.7800922993934));
#83428=CARTESIAN_POINT('Ctrl Pts',(-6.39147534676179,-6.85255440930589,
12.7815069596919));
#83429=CARTESIAN_POINT('Ctrl Pts',(-6.2317213458274,-6.9989376462568,12.7852219176209));
#83430=CARTESIAN_POINT('Ctrl Pts',(-6.13117178901886,-7.08718642700513,
12.7875329021493));
#83431=CARTESIAN_POINT('Ctrl Pts',(-5.89222525986094,-7.28800930340297,
12.7929588891941));
#83432=CARTESIAN_POINT('Ctrl Pts',(-5.75243434474582,-7.39884430122177,
12.7960843535902));
#83433=CARTESIAN_POINT('Ctrl Pts',(-5.37563497706413,-7.68045733034773,
12.8043496006305));
#83434=CARTESIAN_POINT('Ctrl Pts',(-5.1336580771413,-7.84426104338588,12.8095024459661));
#83435=CARTESIAN_POINT('Ctrl Pts',(-4.83179624496502,-8.0286445717061,12.8156132743452));
#83436=CARTESIAN_POINT('Ctrl Pts',(-4.77884886991007,-8.06027245911707,
12.8166735515385));
#83437=CARTESIAN_POINT('Ctrl Pts',(-4.68913456765904,-8.11266815987354,
12.8184483005386));
#83438=CARTESIAN_POINT('Ctrl Pts',(-4.65253263985235,-8.13371426319955,
12.8191662248213));
#83439=CARTESIAN_POINT('Ctrl Pts',(-4.56676460752064,-8.18226249848533,
12.8208340779508));
#83440=CARTESIAN_POINT('Ctrl Pts',(-4.51749035206061,-8.20956999565315,
12.8217815829397));
#83441=CARTESIAN_POINT('Ctrl Pts',(-4.30322510176282,-8.32580131530933,
12.8258617395966));
#83442=CARTESIAN_POINT('Ctrl Pts',(-4.13583254852035,-8.41020828416124,
12.8289483060192));
#83443=CARTESIAN_POINT('Ctrl Pts',(-3.63894454658943,-8.64233731345837,
12.837950020607));
#83444=CARTESIAN_POINT('Ctrl Pts',(-3.30331186751,-8.77610632138951,12.8438402315696));
#83445=CARTESIAN_POINT('Ctrl Pts',(-2.864535648327,-8.92223712349573,12.8515584681707));
#83446=CARTESIAN_POINT('Ctrl Pts',(-2.76775693789938,-8.95273149575373,
12.8532609156138));
#83447=CARTESIAN_POINT('Ctrl Pts',(-2.59472014175691,-9.00418031141225,
12.8563085481742));
#83448=CARTESIAN_POINT('Ctrl Pts',(-2.51865598712167,-9.02575247163691,
12.8576494791912));
#83449=CARTESIAN_POINT('Ctrl Pts',(-2.35235038248011,-9.07065151074197,
12.8605850445473));
#83450=CARTESIAN_POINT('Ctrl Pts',(-2.2620154449943,-9.09359979454418,12.8621820196724));
#83451=CARTESIAN_POINT('Ctrl Pts',(-1.95656691257297,-9.16636143959714,
12.8675902620821));
#83452=CARTESIAN_POINT('Ctrl Pts',(-1.74003986548826,-9.20991839245714,
12.8714396843452));
#83453=CARTESIAN_POINT('Ctrl Pts',(-1.28603651421049,-9.28466311576228,
12.8795095500928));
#83454=CARTESIAN_POINT('Ctrl Pts',(-1.04849290017805,-9.31447914050837,
12.8837313486381));
#83455=CARTESIAN_POINT('Ctrl Pts',(-0.685190450612173,-9.34600509403241,
12.890108429688));
#83456=CARTESIAN_POINT('Ctrl Pts',(-0.560106606395548,-9.35433471193091,
12.8922891930124));
#83457=CARTESIAN_POINT('Ctrl Pts',(-0.382911040754098,-9.36256760574047,
12.8953422833438));
#83458=CARTESIAN_POINT('Ctrl Pts',(-0.330909614492647,-9.36454974253682,
12.8962338398777));
#83459=CARTESIAN_POINT('Ctrl Pts',(-0.236031105329159,-9.36737493981823,
12.8978508380989));
#83460=CARTESIAN_POINT('Ctrl Pts',(-0.193159726206334,-9.36835702052225,
12.8985777179172));
#83461=CARTESIAN_POINT('Ctrl Pts',(-0.0816155101726701,-9.37014623242085,
12.9004602497299));
#83462=CARTESIAN_POINT('Ctrl Pts',(-0.0129377950548491,-9.37049273811119,
12.9016109239267));
#83463=CARTESIAN_POINT('Ctrl Pts',(0.145080983855336,-9.36955276896177,
12.9042448350719));
#83464=CARTESIAN_POINT('Ctrl Pts',(0.23441232761244,-9.36774351118985,12.9057238227766));
#83465=CARTESIAN_POINT('Ctrl Pts',(0.57638925116337,-9.35592253657426,12.9113663418915));
#83466=CARTESIAN_POINT('Ctrl Pts',(0.82861742339648,-9.33696441907064,12.91549038688));
#83467=CARTESIAN_POINT('Ctrl Pts',(1.2826110092072,-9.28429816204319,12.9230043641579));
#83468=CARTESIAN_POINT('Ctrl Pts',(1.48462839762076,-9.25414293830244,12.926380260416));
#83469=CARTESIAN_POINT('Ctrl Pts',(1.77800053430736,-9.20049683013941,12.9313704623495));
#83470=CARTESIAN_POINT('Ctrl Pts',(1.8702426285614,-9.18219038561656,12.9329520442414));
#83471=CARTESIAN_POINT('Ctrl Pts',(2.03943142549801,-9.14595778687076,12.935878770292));
#83472=CARTESIAN_POINT('Ctrl Pts',(2.11645710575987,-9.12844092187949,12.9372211229269));
#83473=CARTESIAN_POINT('Ctrl Pts',(2.29247750111284,-9.08606341337091,12.9403124241253));
#83474=CARTESIAN_POINT('Ctrl Pts',(2.39130591134677,-9.06055502784747,12.9420654426933));
#83475=CARTESIAN_POINT('Ctrl Pts',(2.54915388756929,-9.01705068641718,12.9448931608116));
#83476=CARTESIAN_POINT('Ctrl Pts',(2.60844678982134,-9.00007744159723,12.9459616812974));
#83477=CARTESIAN_POINT('Ctrl Pts',(2.83203035385175,-8.93367911495131,12.9500140796322));
#83478=CARTESIAN_POINT('Ctrl Pts',(2.99512025600217,-8.88033067454188,12.9530182631492));
#83479=CARTESIAN_POINT('Ctrl Pts',(3.44826668350166,-8.7181974509313,12.961471577699));
#83480=CARTESIAN_POINT('Ctrl Pts',(3.73452808140036,-8.59946569538645,12.9669410724945));
#83481=CARTESIAN_POINT('Ctrl Pts',(4.06280398248845,-8.44381907086855,12.9732123726924));
#83482=CARTESIAN_POINT('Ctrl Pts',(4.11102701454227,-8.42044616418483,12.9741333839756));
#83483=CARTESIAN_POINT('Ctrl Pts',(4.19706122418084,-8.3778315672746,12.9757744599883));
#83484=CARTESIAN_POINT('Ctrl Pts',(4.23494718523305,-8.35874434623318,12.9764962958481));
#83485=CARTESIAN_POINT('Ctrl Pts',(4.32108674439266,-8.3146106335009,12.9781352196089));
#83486=CARTESIAN_POINT('Ctrl Pts',(4.36925449945335,-8.28940020607268,12.9790503031754));
#83487=CARTESIAN_POINT('Ctrl Pts',(4.55516101788885,-8.19002835626909,12.9825816351926));
#83488=CARTESIAN_POINT('Ctrl Pts',(4.69125394763809,-8.11284124380121,12.985166063275));
#83489=CARTESIAN_POINT('Ctrl Pts',(5.1046727407326,-7.86448213000443,12.9930967927187));
#83490=CARTESIAN_POINT('Ctrl Pts',(5.37505129806971,-7.68222537600135,12.9984046178871));
#83491=CARTESIAN_POINT('Ctrl Pts',(5.74433574557468,-7.40424124303973,13.0060647548957));
#83492=CARTESIAN_POINT('Ctrl Pts',(5.85148253379142,-7.31985884805236,13.0083386899635));
#83493=CARTESIAN_POINT('Ctrl Pts',(6.02104684056877,-7.18021712838541,13.0120315384967));
#83494=CARTESIAN_POINT('Ctrl Pts',(6.08463542393567,-7.12641107332891,13.0134385508191));
#83495=CARTESIAN_POINT('Ctrl Pts',(6.20993449032956,-7.01748836042729,13.0162572184229));
#83496=CARTESIAN_POINT('Ctrl Pts',(6.27164926696716,-6.96238785879778,13.0176686529798));
#83497=CARTESIAN_POINT('Ctrl Pts',(6.43032537021254,-6.81689596977543,13.0213592351785));
#83498=CARTESIAN_POINT('Ctrl Pts',(6.52611247782977,-6.72525172832812,13.0236487888546));
#83499=CARTESIAN_POINT('Ctrl Pts',(6.74425156272492,-6.50749696273514,13.0290057971199));
#83500=CARTESIAN_POINT('Ctrl Pts',(6.86506517188461,-6.37991581599831,13.0320832877704));
#83501=CARTESIAN_POINT('Ctrl Pts',(7.18269361790264,-6.02501955053656,13.0404505777085));
#83502=CARTESIAN_POINT('Ctrl Pts',(7.37227181144334,-5.79150730705789,13.0457564438124));
#83503=CARTESIAN_POINT('Ctrl Pts',(7.58240183465557,-5.50560679575271,13.0518826554628));
#83504=CARTESIAN_POINT('Ctrl Pts',(7.6141266033911,-5.46164808974323,13.0528145677359));
#83505=CARTESIAN_POINT('Ctrl Pts',(7.67004182562688,-5.38273629649582,13.0544679764983));
#83506=CARTESIAN_POINT('Ctrl Pts',(7.69437924526506,-5.34788927463507,13.0551913491622));
#83507=CARTESIAN_POINT('Ctrl Pts',(7.74899907637573,-5.26853830235075,13.0568228488166));
#83508=CARTESIAN_POINT('Ctrl Pts',(7.77913672583986,-5.22393667145605,13.0577290878064));
#83509=CARTESIAN_POINT('Ctrl Pts',(7.89178738878311,-5.05408472171865,13.0611442062727));
#83510=CARTESIAN_POINT('Ctrl Pts',(7.97167359667654,-4.9271189225842,13.0636239084289));
#83511=CARTESIAN_POINT('Ctrl Pts',(8.26741873616163,-4.43104675282184,13.0731259570789));
#83512=CARTESIAN_POINT('Ctrl Pts',(8.46096716752743,-4.04924970220302,13.0800750421999));
#83513=CARTESIAN_POINT('Ctrl Pts',(8.66455974168202,-3.56873699642781,13.0888062508559));
#83514=CARTESIAN_POINT('Ctrl Pts',(8.70003898389042,-3.48135044073475,13.0903922939249));
#83515=CARTESIAN_POINT('Ctrl Pts',(8.7627920051014,-3.31983396945678,13.0933231135957));
#83516=CARTESIAN_POINT('Ctrl Pts',(8.7904592948343,-3.24586608804979,13.0946650429543));
#83517=CARTESIAN_POINT('Ctrl Pts',(8.8516080132118,-3.07586766535325,13.0977495036896));
#83518=CARTESIAN_POINT('Ctrl Pts',(8.8844677068294,-2.97962410561035,13.0994960340303));
#83519=CARTESIAN_POINT('Ctrl Pts',(8.99008920548138,-2.65297150767494,13.1054243968104));
#83520=CARTESIAN_POINT('Ctrl Pts',(9.05550432857714,-2.42028973016568,13.1096506692804));
#83521=CARTESIAN_POINT('Ctrl Pts',(9.18324912565045,-1.88765355191921,13.119273402367));
#83522=CARTESIAN_POINT('Ctrl Pts',(9.24001388046839,-1.58664561440863,13.1246774811176));
#83523=CARTESIAN_POINT('Ctrl Pts',(9.28907055922692,-1.23185273654909,13.1308562623385));
#83524=CARTESIAN_POINT('Ctrl Pts',(9.29576844986479,-1.18024656775215,13.1317501245812));
#83525=CARTESIAN_POINT('Ctrl Pts',(9.30712570265132,-1.08663787399349,13.1333611335782));
#83526=CARTESIAN_POINT('Ctrl Pts',(9.31193145695597,-1.0446546177922,13.1340797863737));
#83527=CARTESIAN_POINT('Ctrl Pts',(9.32242962766803,-0.947106437277983,
13.1357403679375));
#83528=CARTESIAN_POINT('Ctrl Pts',(9.32790952965615,-0.89152038246043,13.1366799741992));
#83529=CARTESIAN_POINT('Ctrl Pts',(9.34879909981048,-0.658283431274132,
13.1406003733128));
#83530=CARTESIAN_POINT('Ctrl Pts',(9.35963314326727,-0.48025981470389,13.1435395454143));
#83531=CARTESIAN_POINT('Ctrl Pts',(9.37794377329943,0.0875082831141098,
13.1528676378549));
#83532=CARTESIAN_POINT('Ctrl Pts',(9.3661904525347,0.477455175517611,13.1592207647935));
#83533=CARTESIAN_POINT('Ctrl Pts',(9.32133925177111,0.96093675570428,13.1673404949271));
#83534=CARTESIAN_POINT('Ctrl Pts',(9.31102639980315,1.05619705567807,13.168951083296));
#83535=CARTESIAN_POINT('Ctrl Pts',(9.29053091358485,1.22174528592883,13.1717715166063));
#83536=CARTESIAN_POINT('Ctrl Pts',(9.2810067474086,1.29210677964924,13.172977027119));
#83537=CARTESIAN_POINT('Ctrl Pts',(9.25679874402869,1.4568399459976,13.1758160722478));
#83538=CARTESIAN_POINT('Ctrl Pts',(9.24146996357503,1.55110878714696,13.1774536235183));
#83539=CARTESIAN_POINT('Ctrl Pts',(9.17901015662336,1.90133906214024,13.1835858347068));
#83540=CARTESIAN_POINT('Ctrl Pts',(9.12266314410927,2.15553564234341,13.1881365587494));
#83541=CARTESIAN_POINT('Ctrl Pts',(8.97787556137494,2.70025458588588,13.1980388728562));
#83542=CARTESIAN_POINT('Ctrl Pts',(8.88574909795208,2.98949624088858,13.2033937619685));
#83543=CARTESIAN_POINT('Ctrl Pts',(8.76139256352825,3.32300279817431,13.2095353509837));
#83544=CARTESIAN_POINT('Ctrl Pts',(8.7426164696698,3.37209201074434,13.2104382964981));
#83545=CARTESIAN_POINT('Ctrl Pts',(8.70798289222226,3.46040586687653,13.2120592530836));
#83546=CARTESIAN_POINT('Ctrl Pts',(8.69227088699294,3.49968593709256,13.2127788595037));
#83547=CARTESIAN_POINT('Ctrl Pts',(8.65539685000357,3.59009078517071,13.2144316495641));
#83548=CARTESIAN_POINT('Ctrl Pts',(8.63404696896634,3.64113710720642,13.2153626220637));
#83549=CARTESIAN_POINT('Ctrl Pts',(8.54536381959219,3.84800679678382,13.2191316044131));
#83550=CARTESIAN_POINT('Ctrl Pts',(8.47425412391052,4.00217647000133,13.2219319852535));
#83551=CARTESIAN_POINT('Ctrl Pts',(8.21873165430379,4.51877778819516,13.2314006962793));
#83552=CARTESIAN_POINT('Ctrl Pts',(8.0149380815139,4.87110566085093,13.2380225707983));
#83553=CARTESIAN_POINT('Ctrl Pts',(7.73692410563497,5.28680754316323,13.2463919431851));
#83554=CARTESIAN_POINT('Ctrl Pts',(7.68378153509765,5.36375147471542,13.2479648868423));
#83555=CARTESIAN_POINT('Ctrl Pts',(7.58361418222493,5.50423719684747,13.2508837819991));
#83556=CARTESIAN_POINT('Ctrl Pts',(7.53691978885827,5.56800424267922,13.2522270503616));
#83557=CARTESIAN_POINT('Ctrl Pts',(7.42764431889087,5.71333992846203,13.2553321639237));
#83558=CARTESIAN_POINT('Ctrl Pts',(7.36451637838112,5.79448459369722,13.2570982219685));
#83559=CARTESIAN_POINT('Ctrl Pts',(7.14308511982483,6.0696471600657,13.2631991908054));
#83560=CARTESIAN_POINT('Ctrl Pts',(6.97834851778531,6.25834905152918,13.2675822606507));
#83561=CARTESIAN_POINT('Ctrl Pts',(6.60964995333837,6.64800245765126,13.2770091556841));
#83562=CARTESIAN_POINT('Ctrl Pts',(6.40363534762744,6.84666808760753,13.2820541836698));
#83563=CARTESIAN_POINT('Ctrl Pts',(6.14273390542827,7.07616976783365,13.2880566769176));
#83564=CARTESIAN_POINT('Ctrl Pts',(6.09621340191157,7.11628699528127,13.289112657993));
#83565=CARTESIAN_POINT('Ctrl Pts',(6.01706772419022,7.1831930651257,13.290882901814));
#83566=CARTESIAN_POINT('Ctrl Pts',(5.98465001734411,7.2102240459162,13.29160056726));
#83567=CARTESIAN_POINT('Ctrl Pts',(5.9083911308696,7.27294265078089,13.2932714101589));
#83568=CARTESIAN_POINT('Ctrl Pts',(5.86440754171859,7.30845433464309,13.294222122728));
#83569=CARTESIAN_POINT('Ctrl Pts',(5.66993537020783,7.46258225059225,13.2983753006177));
#83570=CARTESIAN_POINT('Ctrl Pts',(5.51614962886845,7.57696474061692,13.3015295518007));
#83571=CARTESIAN_POINT('Ctrl Pts',(5.06747275471185,7.88977648066575,13.3105053524285));
#83572=CARTESIAN_POINT('Ctrl Pts',(4.76465719249937,8.07625498798875,13.3163052553085));
#83573=CARTESIAN_POINT('Ctrl Pts',(4.39857396922947,8.27392388623823,13.3232478694169));
#83574=CARTESIAN_POINT('Ctrl Pts',(4.34488551263815,8.30224301434379,13.3242640118924));
#83575=CARTESIAN_POINT('Ctrl Pts',(4.29092662791762,8.33003803930856,13.3252837277684));
#83576=CARTESIAN_POINT('Origin',(0.,0.,2.15141010809499));
#83577=CARTESIAN_POINT('',(4.29092664592493,8.33003803003272,14.5226929117958));
#83578=CARTESIAN_POINT('',(4.29092662550047,8.33003804055367,14.3259466798393));
#83579=CARTESIAN_POINT('',(4.29092662815669,8.33003803918541,2.15141010809499));
#83580=CARTESIAN_POINT('Ctrl Pts',(4.29092664592493,8.33003803003272,14.5226929117958));
#83581=CARTESIAN_POINT('Ctrl Pts',(4.41553143336263,8.26585224832338,14.5203910368916));
#83582=CARTESIAN_POINT('Ctrl Pts',(4.53869923662709,8.1988689706793,14.5180966839689));
#83583=CARTESIAN_POINT('Ctrl Pts',(4.80974732334025,8.04348037186033,14.5129714010413));
#83584=CARTESIAN_POINT('Ctrl Pts',(4.95676878350567,7.95372169977639,14.5101388142208));
#83585=CARTESIAN_POINT('Ctrl Pts',(5.1530909291932,7.82630570587419,14.5062565808397));
#83586=CARTESIAN_POINT('Ctrl Pts',(5.20461481983927,7.79213652924653,14.5052281564504));
#83587=CARTESIAN_POINT('Ctrl Pts',(5.34042591853822,7.70012245118076,14.5024901163469));
#83588=CARTESIAN_POINT('Ctrl Pts',(5.4241109934168,7.64140396903468,14.5007746664135));
#83589=CARTESIAN_POINT('Ctrl Pts',(5.57073460871978,7.53490157113011,14.4977146713401));
#83590=CARTESIAN_POINT('Ctrl Pts',(5.6340610406389,7.48766865747195,14.4963745535729));
#83591=CARTESIAN_POINT('Ctrl Pts',(5.77134902899967,7.38254263772988,14.4934272965316));
#83592=CARTESIAN_POINT('Ctrl Pts',(5.8450527417186,7.32432684983428,14.4918176722641));
#83593=CARTESIAN_POINT('Ctrl Pts',(6.22724754380438,7.01300205932098,14.483325113055));
#83594=CARTESIAN_POINT('Ctrl Pts',(6.52021169938399,6.74148691573541,14.4762878326506));
#83595=CARTESIAN_POINT('Ctrl Pts',(6.91561422797623,6.3250740976944,14.466208962389));
#83596=CARTESIAN_POINT('Ctrl Pts',(7.03267048619861,6.19466129951294,14.4631455211113));
#83597=CARTESIAN_POINT('Ctrl Pts',(7.18201270378426,6.01858604658367,14.4591655379477));
#83598=CARTESIAN_POINT('Ctrl Pts',(7.21764473847748,5.9758086420046,14.4582103386609));
#83599=CARTESIAN_POINT('Ctrl Pts',(7.27965813316047,5.89999572049102,14.4565398354746));
#83600=CARTESIAN_POINT('Ctrl Pts',(7.30620094821504,5.86709465966543,14.4558223117547));
#83601=CARTESIAN_POINT('Ctrl Pts',(7.36502958496784,5.79315549761531,14.4542258462433));
#83602=CARTESIAN_POINT('Ctrl Pts',(7.3971967733645,5.75202497548105,14.4533484961273));
#83603=CARTESIAN_POINT('Ctrl Pts',(7.61575329263613,5.46770238935765,14.4473492554394));
#83604=CARTESIAN_POINT('Ctrl Pts',(7.79046114654486,5.21576306877197,14.4423538894095));
#83605=CARTESIAN_POINT('Ctrl Pts',(8.0891311184044,4.73648301312642,14.4330912607407));
#83606=CARTESIAN_POINT('Ctrl Pts',(8.21662561139473,4.51169331703398,14.4288377725612));
#83607=CARTESIAN_POINT('Ctrl Pts',(8.37827401906551,4.19704835303852,14.4229216178048));
#83608=CARTESIAN_POINT('Ctrl Pts',(8.42057988858439,4.11151124284804,14.4213173937684));
#83609=CARTESIAN_POINT('Ctrl Pts',(8.49547003210463,3.95408656582391,14.4183695760692));
#83610=CARTESIAN_POINT('Ctrl Pts',(8.52846670560356,3.88240482873441,14.4170290552328));
#83611=CARTESIAN_POINT('Ctrl Pts',(8.60133125536355,3.71870158749817,14.4139706021536));
#83612=CARTESIAN_POINT('Ctrl Pts',(8.64063516318555,3.62643968251163,14.4122489431954));
#83613=CARTESIAN_POINT('Ctrl Pts',(8.80228287424431,3.22943220904156,14.4048495947702));
#83614=CARTESIAN_POINT('Ctrl Pts',(8.91004183844394,2.91900134520566,14.3990775107848));
#83615=CARTESIAN_POINT('Ctrl Pts',(9.05866365599653,2.40517105667305,14.389674935079));
#83616=CARTESIAN_POINT('Ctrl Pts',(9.10947144826249,2.20494111084259,14.38604955173));
#83617=CARTESIAN_POINT('Ctrl Pts',(9.16760365959272,1.93930547025714,14.3813463270801));
#83618=CARTESIAN_POINT('Ctrl Pts',(9.18091632633381,1.87527011502343,14.3802207141548));
#83619=CARTESIAN_POINT('Ctrl Pts',(9.20170405316214,1.7697468946918,14.3783820031541));
#83620=CARTESIAN_POINT('Ctrl Pts',(9.20957147844763,1.72833872712739,14.3776646376361));
#83621=CARTESIAN_POINT('Ctrl Pts',(9.22679819527974,1.63421139341723,14.3760438498222));
#83622=CARTESIAN_POINT('Ctrl Pts',(9.23598552473437,1.58146236728408,14.3751423213675));
#83623=CARTESIAN_POINT('Ctrl Pts',(9.26724655979226,1.39240542106139,14.3719310383201));
#83624=CARTESIAN_POINT('Ctrl Pts',(9.28675885884841,1.25569174178744,14.3696455056696));
#83625=CARTESIAN_POINT('Ctrl Pts',(9.33774124030956,0.831676988831244,14.3626126174047));
#83626=CARTESIAN_POINT('Ctrl Pts',(9.35894797618795,0.543314996162689,14.3579040089817));
#83627=CARTESIAN_POINT('Ctrl Pts',(9.36902687240109,0.172269232477673,14.3517813640476));
#83628=CARTESIAN_POINT('Ctrl Pts',(9.37017754171549,0.0900779407209574,
14.3504215121783));
#83629=CARTESIAN_POINT('Ctrl Pts',(9.37035024095918,-0.115223120611711,
14.3470111847114));
#83630=CARTESIAN_POINT('Ctrl Pts',(9.36802776886569,-0.238318309557992,
14.3449540587861));
#83631=CARTESIAN_POINT('Ctrl Pts',(9.36014352363104,-0.442624763483723,
14.3415121533339));
#83632=CARTESIAN_POINT('Ctrl Pts',(9.35594784627133,-0.523873387064799,
14.3401361603886));
#83633=CARTESIAN_POINT('Ctrl Pts',(9.34519705755782,-0.690018646916564,
14.337306252971));
#83634=CARTESIAN_POINT('Ctrl Pts',(9.33854173039163,-0.774901339090052,
14.3358518202348));
#83635=CARTESIAN_POINT('Ctrl Pts',(9.31706256520254,-1.00802991795948,14.3318328033841));
#83636=CARTESIAN_POINT('Ctrl Pts',(9.2998586721235,-1.15603098362047,14.3292538033239));
#83637=CARTESIAN_POINT('Ctrl Pts',(9.23416013762911,-1.62369352665651,14.3210257166661));
#83638=CARTESIAN_POINT('Ctrl Pts',(9.1726495594576,-1.94128647176708,14.3153135305538));
#83639=CARTESIAN_POINT('Ctrl Pts',(9.06096294510859,-2.39172768718551,14.3071869788792));
#83640=CARTESIAN_POINT('Ctrl Pts',(9.02400055794059,-2.52761249779053,14.3047334804076));
#83641=CARTESIAN_POINT('Ctrl Pts',(8.96893557800252,-2.71340865089643,14.301396743458));
#83642=CARTESIAN_POINT('Ctrl Pts',(8.95345052841331,-2.76407589645491,14.3004886972824));
#83643=CARTESIAN_POINT('Ctrl Pts',(8.92472210135113,-2.85530041607536,14.298858886342));
#83644=CARTESIAN_POINT('Ctrl Pts',(8.91162989479709,-2.89590360158452,14.2981354757689));
#83645=CARTESIAN_POINT('Ctrl Pts',(8.87732055692088,-2.99987164762169,14.2962873148611));
#83646=CARTESIAN_POINT('Ctrl Pts',(8.85570206141893,-3.06310156585481,14.2951671561396));
#83647=CARTESIAN_POINT('Ctrl Pts',(8.72566871974879,-3.43053688915144,14.2886669335851));
#83648=CARTESIAN_POINT('Ctrl Pts',(8.60226124141433,-3.7292065038023,14.2834122025149));
#83649=CARTESIAN_POINT('Ctrl Pts',(8.36584030670943,-4.2268530833878,14.2743642038139));
#83650=CARTESIAN_POINT('Ctrl Pts',(8.26051643301879,-4.42915780090858,14.2706003591972));
#83651=CARTESIAN_POINT('Ctrl Pts',(8.10163124318907,-4.70892148459844,14.2652164407184));
#83652=CARTESIAN_POINT('Ctrl Pts',(8.05412333252604,-4.78972521546493,14.2636398575589));
#83653=CARTESIAN_POINT('Ctrl Pts',(7.96434743445288,-4.93730676312348,14.2607176836783));
#83654=CARTESIAN_POINT('Ctrl Pts',(7.92243150690984,-5.00428887199618,14.2593748218893));
#83655=CARTESIAN_POINT('Ctrl Pts',(7.82516460160302,-5.15543694010044,14.2563056384726));
#83656=CARTESIAN_POINT('Ctrl Pts',(7.76929352468109,-5.23925654506466,14.2545755227633));
#83657=CARTESIAN_POINT('Ctrl Pts',(7.53614208166534,-5.57710497999386,14.2474867627891));
#83658=CARTESIAN_POINT('Ctrl Pts',(7.34766892289693,-5.82316901339678,14.2420465038897));
#83659=CARTESIAN_POINT('Ctrl Pts',(6.99525451965885,-6.23885589991609,14.2324653663628));
#83660=CARTESIAN_POINT('Ctrl Pts',(6.83645003253995,-6.41247691052005,14.2283323215129));
#83661=CARTESIAN_POINT('Ctrl Pts',(6.63007250681849,-6.6217193702175,14.2232602747088));
#83662=CARTESIAN_POINT('Ctrl Pts',(6.5884720756188,-6.66311223036442,14.2222523428036));
#83663=CARTESIAN_POINT('Ctrl Pts',(6.51929243672265,-6.73066532733789,14.2206018408587));
#83664=CARTESIAN_POINT('Ctrl Pts',(6.49193811252706,-6.75705329093956,14.2199557758819));
#83665=CARTESIAN_POINT('Ctrl Pts',(6.42475116195198,-6.82108209363545,14.2183848887671));
#83666=CARTESIAN_POINT('Ctrl Pts',(6.38474747299337,-6.8585412549335,14.217462848424));
#83667=CARTESIAN_POINT('Ctrl Pts',(6.2213330296312,-7.00889253964606,14.21374449792));
#83668=CARTESIAN_POINT('Ctrl Pts',(6.09523824214875,-7.1188222615964,14.2109846643167));
#83669=CARTESIAN_POINT('Ctrl Pts',(5.76192869360673,-7.3940508719286,14.2038821902126));
#83670=CARTESIAN_POINT('Ctrl Pts',(5.55052295966463,-7.55403901986238,14.1995578552151));
#83671=CARTESIAN_POINT('Ctrl Pts',(5.23548843609199,-7.77207823608147,14.1932335911115));
#83672=CARTESIAN_POINT('Ctrl Pts',(5.13709326449169,-7.83746208810513,14.191274920228));
#83673=CARTESIAN_POINT('Ctrl Pts',(4.9509365725732,-7.95615161802202,14.1875904749214));
#83674=CARTESIAN_POINT('Ctrl Pts',(4.86348396457868,-8.00990918627904,14.1858680962079));
#83675=CARTESIAN_POINT('Ctrl Pts',(4.70717430941078,-8.10248972113392,14.1828007753582));
#83676=CARTESIAN_POINT('Ctrl Pts',(4.63867604494597,-8.14189868375936,14.1814603447239));
#83677=CARTESIAN_POINT('Ctrl Pts',(4.48796000798931,-8.22609042712171,14.1785180404294));
#83678=CARTESIAN_POINT('Ctrl Pts',(4.4055529838738,-8.27051700920359,14.1769137423157));
#83679=CARTESIAN_POINT('Ctrl Pts',(3.96347272233249,-8.50036522412387,14.1683304761735));
#83680=CARTESIAN_POINT('Ctrl Pts',(3.59273783926825,-8.66357640937482,14.1611917970008));
#83681=CARTESIAN_POINT('Ctrl Pts',(3.05185516295581,-8.86098489521453,14.1510878866383));
#83682=CARTESIAN_POINT('Ctrl Pts',(2.88951236659296,-8.91524491032447,14.1480967020569));
#83683=CARTESIAN_POINT('Ctrl Pts',(2.67275125768042,-8.98115010212507,14.1441916059361));
#83684=CARTESIAN_POINT('Ctrl Pts',(2.61958582631218,-8.99680090698764,14.1432408255099));
#83685=CARTESIAN_POINT('Ctrl Pts',(2.52560543177585,-9.02356311271159,14.1415743471479));
#83686=CARTESIAN_POINT('Ctrl Pts',(2.48484846218899,-9.03487145283563,14.1408564824741));
#83687=CARTESIAN_POINT('Ctrl Pts',(2.38330148272883,-9.06230734732912,14.1390793526512));
#83688=CARTESIAN_POINT('Ctrl Pts',(2.3224231313323,-9.07809953902534,14.1380238699629));
#83689=CARTESIAN_POINT('Ctrl Pts',(1.9566946973666,-9.16905186367538,14.1317308710709));
#83690=CARTESIAN_POINT('Ctrl Pts',(1.64838192905665,-9.22946395273604,14.1266174208279));
#83691=CARTESIAN_POINT('Ctrl Pts',(1.13902322594581,-9.30292812518079,14.1181715317708));
#83692=CARTESIAN_POINT('Ctrl Pts',(0.939559463208026,-9.3251848961384,14.1148662869053));
#83693=CARTESIAN_POINT('Ctrl Pts',(0.629275673813051,-9.34975030003893,
14.1096822416045));
#83694=CARTESIAN_POINT('Ctrl Pts',(0.518869910488682,-9.35652673159926,
14.1078296364565));
#83695=CARTESIAN_POINT('Ctrl Pts',(0.328714744639834,-9.36482187551713,
14.1046202270309));
#83696=CARTESIAN_POINT('Ctrl Pts',(0.249018208894852,-9.36727986347498,
14.1032695374666));
#83697=CARTESIAN_POINT('Ctrl Pts',(0.0801230676384112,-9.37033193130456,
14.1003941092843));
#83698=CARTESIAN_POINT('Ctrl Pts',(-0.00907231179823951,-9.3706700856364,
14.0988678714167));
#83699=CARTESIAN_POINT('Ctrl Pts',(-0.277989500013457,-9.36784999826492,
14.0942426997848));
#83700=CARTESIAN_POINT('Ctrl Pts',(-0.457628244701591,-9.36079418651735,
14.0911204785561));
#83701=CARTESIAN_POINT('Ctrl Pts',(-0.692409234804157,-9.344797711926,14.0870059677661));
#83702=CARTESIAN_POINT('Ctrl Pts',(-0.747831548845888,-9.34052583068818,
14.0860322951669));
#83703=CARTESIAN_POINT('Ctrl Pts',(-1.04376177960404,-9.31506514575889,
14.0808226317056));
#83704=CARTESIAN_POINT('Ctrl Pts',(-1.28342109327622,-9.2850798357019,14.076563229374));
#83705=CARTESIAN_POINT('Ctrl Pts',(-1.60810050393344,-9.23164520673233,
14.0708105156161));
#83706=CARTESIAN_POINT('Ctrl Pts',(-1.69434327439867,-9.21620645209041,
14.0692844882224));
#83707=CARTESIAN_POINT('Ctrl Pts',(-1.84686722416187,-9.18668905603141,
14.0665956147054));
#83708=CARTESIAN_POINT('Ctrl Pts',(-1.91323609195933,-9.17309664421673,
14.0654289671049));
#83709=CARTESIAN_POINT('Ctrl Pts',(-2.02125451952012,-9.14975105238991,
14.0635387651339));
#83710=CARTESIAN_POINT('Ctrl Pts',(-2.06299492529017,-9.14043030240214,
14.0628105244323));
#83711=CARTESIAN_POINT('Ctrl Pts',(-2.15582573560471,-9.11903264506006,
14.0611963698826));
#83712=CARTESIAN_POINT('Ctrl Pts',(-2.20688130723002,-9.10681151097122,
14.0603120511362));
#83713=CARTESIAN_POINT('Ctrl Pts',(-2.37210703373872,-9.06579048459115,
14.0574577347068));
#83714=CARTESIAN_POINT('Ctrl Pts',(-2.48583789377713,-9.03526751037888,
14.055504573038));
#83715=CARTESIAN_POINT('Ctrl Pts',(-2.8929529565998,-8.91773745403488,14.0485127964624));
#83716=CARTESIAN_POINT('Ctrl Pts',(-3.1826087914494,-8.81851574618484,14.0435320856308));
#83717=CARTESIAN_POINT('Ctrl Pts',(-3.54519577559341,-8.6741153008183,14.0370971522446));
#83718=CARTESIAN_POINT('Ctrl Pts',(-3.62307690161824,-8.64187497462917,
14.0357033242861));
#83719=CARTESIAN_POINT('Ctrl Pts',(-3.81543564102982,-8.55918709783806,
14.032226584086));
#83720=CARTESIAN_POINT('Ctrl Pts',(-3.92935789753884,-8.5074896005878,14.0301369802971));
#83721=CARTESIAN_POINT('Ctrl Pts',(-4.11586141311511,-8.41830948493116,
14.0266576421233));
#83722=CARTESIAN_POINT('Ctrl Pts',(-4.1890486065118,-8.38213108294013,14.0252771410141));
#83723=CARTESIAN_POINT('Ctrl Pts',(-4.328082189294,-8.31112727242924,14.0226241444642));
#83724=CARTESIAN_POINT('Ctrl Pts',(-4.39400449189261,-8.27646400782297,
14.0213528949536));
#83725=CARTESIAN_POINT('Ctrl Pts',(-4.57594156285564,-8.17801142773907,
14.0178066109427));
#83726=CARTESIAN_POINT('Ctrl Pts',(-4.691027999729,-8.11254388328858,14.0155199107824));
#83727=CARTESIAN_POINT('Ctrl Pts',(-5.08569937248299,-7.87682566338534,
14.0075303317785));
#83728=CARTESIAN_POINT('Ctrl Pts',(-5.35772294839735,-7.69438263699696,
14.0017524467386));
#83729=CARTESIAN_POINT('Ctrl Pts',(-5.74869479152734,-7.40135825181959,
13.9931835222997));
#83730=CARTESIAN_POINT('Ctrl Pts',(-5.87523154447009,-7.30131839634986,
13.9903672980119));
#83731=CARTESIAN_POINT('Ctrl Pts',(-6.04117228970698,-7.16301742965472,
13.9866449361048));
#83732=CARTESIAN_POINT('Ctrl Pts',(-6.08291338559152,-7.12760451297037,
13.9857060951486));
#83733=CARTESIAN_POINT('Ctrl Pts',(-6.15641123895333,-7.06413343204732,
13.9840502928625));
#83734=CARTESIAN_POINT('Ctrl Pts',(-6.18829226972866,-7.03622194613415,
13.9833313090473));
#83735=CARTESIAN_POINT('Ctrl Pts',(-6.26776091341443,-6.96569013772745,
13.9815365549696));
#83736=CARTESIAN_POINT('Ctrl Pts',(-6.31510397482343,-6.92279768425885,
13.9804647710152));
#83737=CARTESIAN_POINT('Ctrl Pts',(-6.52040655012673,-6.73293645606438,
13.9757968909284));
#83738=CARTESIAN_POINT('Ctrl Pts',(-6.67370215175149,-6.5810208221157,13.9722571648482));
#83739=CARTESIAN_POINT('Ctrl Pts',(-6.97282701830862,-6.26337892853039,
13.9651044947037));
#83740=CARTESIAN_POINT('Ctrl Pts',(-7.11832015696917,-6.09752000679087,
13.9614936836005));
#83741=CARTESIAN_POINT('Ctrl Pts',(-7.32698429942988,-5.84198956299416,
13.9560381194012));
#83742=CARTESIAN_POINT('Ctrl Pts',(-7.39465595401591,-5.75609279209739,
13.954221715597));
#83743=CARTESIAN_POINT('Ctrl Pts',(-7.51977380125169,-5.59142968937894,
13.9507652199054));
#83744=CARTESIAN_POINT('Ctrl Pts',(-7.57752447288718,-5.51291273253487,
13.9491276447415));
#83745=CARTESIAN_POINT('Ctrl Pts',(-7.67976947159933,-5.3692592791391,13.9461474813707));
#83746=CARTESIAN_POINT('Ctrl Pts',(-7.72468626654299,-5.30443459696192,
13.9448083749976));
#83747=CARTESIAN_POINT('Ctrl Pts',(-7.82357904406067,-5.15779044241598,
13.9417908055288));
#83748=CARTESIAN_POINT('Ctrl Pts',(-7.87710032031722,-5.0756755005845,13.9401090536203));
#83749=CARTESIAN_POINT('Ctrl Pts',(-8.1155793114134,-4.6969298635971,13.9323882307437));
#83750=CARTESIAN_POINT('Ctrl Pts',(-8.28513585671026,-4.39093376793133,
13.9262383423604));
#83751=CARTESIAN_POINT('Ctrl Pts',(-8.49942070118269,-3.94739055133575,
13.9175816780624));
#83752=CARTESIAN_POINT('Ctrl Pts',(-8.55868626075188,-3.81718928196004,
13.9150720414695));
#83753=CARTESIAN_POINT('Ctrl Pts',(-8.65177061248846,-3.59961305642349,
13.9109524808511));
#83754=CARTESIAN_POINT('Ctrl Pts',(-8.68730131349187,-3.5129965623906,13.9093316048868));
#83755=CARTESIAN_POINT('Ctrl Pts',(-8.73866235313251,-3.38224210000726,
13.9069203213655));
#83756=CARTESIAN_POINT('Ctrl Pts',(-8.7554690546953,-3.33849412008678,13.9061194645881));
#83757=CARTESIAN_POINT('Ctrl Pts',(-8.78593169694011,-3.25738718520531,
13.9046468129294));
#83758=CARTESIAN_POINT('Ctrl Pts',(-8.79967930924727,-3.22006383724469,
13.9039738752412));
#83759=CARTESIAN_POINT('Ctrl Pts',(-8.83931408695079,-3.11030991042829,
13.9020074291811));
#83760=CARTESIAN_POINT('Ctrl Pts',(-8.86454759273273,-3.03764666924492,
13.9007212916723));
#83761=CARTESIAN_POINT('Ctrl Pts',(-9.0023590937942,-2.62445198028432,13.8934771973611));
#83762=CARTESIAN_POINT('Ctrl Pts',(-9.09620752522032,-2.27798771930265,
13.8876565836677));
#83763=CARTESIAN_POINT('Ctrl Pts',(-9.19690587418681,-1.7987964615335,13.8795913462017));
#83764=CARTESIAN_POINT('Ctrl Pts',(-9.22115485537858,-1.67004473007707,
13.8774243699864));
#83765=CARTESIAN_POINT('Ctrl Pts',(-9.26078058992441,-1.43234862053761,
13.8734102385142));
#83766=CARTESIAN_POINT('Ctrl Pts',(-9.27695358451175,-1.32356027968628,
13.8715679342886));
#83767=CARTESIAN_POINT('Ctrl Pts',(-9.30153318469591,-1.13552257876829,
13.8683700018249));
#83768=CARTESIAN_POINT('Ctrl Pts',(-9.31085073514806,-1.05640412072303,
13.8670203593496));
#83769=CARTESIAN_POINT('Ctrl Pts',(-9.32848884955114,-0.888192580895698,
13.8641410870145));
#83770=CARTESIAN_POINT('Ctrl Pts',(-9.33654443321036,-0.799079642526897,
13.8626098962689));
#83771=CARTESIAN_POINT('Ctrl Pts',(-9.35712095283545,-0.528249251967711,
13.8579381253025));
#83772=CARTESIAN_POINT('Ctrl Pts',(-9.36562098330871,-0.346270188238063,
13.8547734871127));
#83773=CARTESIAN_POINT('Ctrl Pts',(-9.36977196277894,-0.109368393421076,
13.8506298389285));
#83774=CARTESIAN_POINT('Ctrl Pts',(-9.37025134270526,-0.0545696691307214,
13.8496697702825));
#83775=CARTESIAN_POINT('Ctrl Pts',(-9.37024410499375,0.240202499639741,
13.8444989748901));
#83776=CARTESIAN_POINT('Ctrl Pts',(-9.36101966834846,0.480085975229739,
13.8402656326414));
#83777=CARTESIAN_POINT('Ctrl Pts',(-9.33338372985667,0.839009173947528,
13.8339726392789));
#83778=CARTESIAN_POINT('Ctrl Pts',(-9.32187231826443,0.958480490726684,
13.8318853256884));
#83779=CARTESIAN_POINT('Ctrl Pts',(-9.30203540768689,1.12981175493476,13.828916184414));
#83780=CARTESIAN_POINT('Ctrl Pts',(-9.29556404183573,1.18187414226275,13.8280172043398));
#83781=CARTESIAN_POINT('Ctrl Pts',(-9.28302299728749,1.2762832362994,13.8263945473307));
#83782=CARTESIAN_POINT('Ctrl Pts',(-9.27709991355352,1.3186478149317,13.82566933824));
#83783=CARTESIAN_POINT('Ctrl Pts',(-9.26103750239161,1.42806444618472,13.8238028578907));
#83784=CARTESIAN_POINT('Ctrl Pts',(-9.25045999356793,1.49504970572261,13.8226663843218));
#83785=CARTESIAN_POINT('Ctrl Pts',(-9.2245315301432,1.64842375461007,13.8200730063592));
#83786=CARTESIAN_POINT('Ctrl Pts',(-9.20869245601344,1.73472364442692,13.8186201685728));
#83787=CARTESIAN_POINT('Ctrl Pts',(-9.14456988660279,2.05842506823737,13.8131770683576));
#83788=CARTESIAN_POINT('Ctrl Pts',(-9.08829808655264,2.29414697965855,13.809223927235));
#83789=CARTESIAN_POINT('Ctrl Pts',(-9.00787157824631,2.58127136314302,13.8043251368891));
#83790=CARTESIAN_POINT('Ctrl Pts',(-8.99230635888001,2.63498359823216,13.8034051992696));
#83791=CARTESIAN_POINT('Ctrl Pts',(-8.92497186402435,2.85979298909571,13.7995370126706));
#83792=CARTESIAN_POINT('Ctrl Pts',(-8.86879299126211,3.02952955320144,13.7965721042473));
#83793=CARTESIAN_POINT('Ctrl Pts',(-8.77739722496202,3.2812828844081,13.7920823504153));
#83794=CARTESIAN_POINT('Ctrl Pts',(-8.74580849991994,3.3645732342173,13.7905816794239));
#83795=CARTESIAN_POINT('Ctrl Pts',(-8.6836921765146,3.52156742356715,13.7877218401226));
#83796=CARTESIAN_POINT('Ctrl Pts',(-8.65340150464513,3.59535663040606,13.7863644077925));
#83797=CARTESIAN_POINT('Ctrl Pts',(-8.5787619580089,3.7707719751039,13.7831047109074));
#83798=CARTESIAN_POINT('Ctrl Pts',(-8.533544168338,3.87201521926783,13.7811966584083));
#83799=CARTESIAN_POINT('Ctrl Pts',(-8.39944085077717,4.15850803882637,13.7757217426879));
#83800=CARTESIAN_POINT('Ctrl Pts',(-8.30624515895175,4.34166864832538,13.7721287101676));
#83801=CARTESIAN_POINT('Ctrl Pts',(-8.05845255641957,4.79143249282006,13.7631112123862));
#83802=CARTESIAN_POINT('Ctrl Pts',(-7.89658530055598,5.05375343474557,13.7576700050687));
#83803=CARTESIAN_POINT('Ctrl Pts',(-7.68632861431998,5.35965707542605,13.7512542474664));
#83804=CARTESIAN_POINT('Ctrl Pts',(-7.6500397832216,5.41132727481883,13.750168299531));
#83805=CARTESIAN_POINT('Ctrl Pts',(-7.58856337718146,5.49700658673556,13.748366327086));
#83806=CARTESIAN_POINT('Ctrl Pts',(-7.56366272111175,5.53121883511605,13.7476465529267));
#83807=CARTESIAN_POINT('Ctrl Pts',(-7.50571931583751,5.6097071804396,13.7459950099833));
#83808=CARTESIAN_POINT('Ctrl Pts',(-7.47251510179593,5.65386196955163,13.745065434287));
#83809=CARTESIAN_POINT('Ctrl Pts',(-7.33648406212632,5.83146357684849,13.7413191909838));
#83810=CARTESIAN_POINT('Ctrl Pts',(-7.23045730687502,5.96242008795891,13.7385395727592));
#83811=CARTESIAN_POINT('Ctrl Pts',(-6.86833710671536,6.38581143121096,13.7293857777355));
#83812=CARTESIAN_POINT('Ctrl Pts',(-6.597585176304,6.66517158078645,13.7230556719449));
#83813=CARTESIAN_POINT('Ctrl Pts',(-6.23617953434901,6.99440452879525,13.7148912824687));
#83814=CARTESIAN_POINT('Ctrl Pts',(-6.16101153239794,7.06070582382147,13.7132085478911));
#83815=CARTESIAN_POINT('Ctrl Pts',(-6.02478838954073,7.17702836814655,13.710182699458));
#83816=CARTESIAN_POINT('Ctrl Pts',(-5.96413747681894,7.22750824696467,13.7088436162022));
#83817=CARTESIAN_POINT('Ctrl Pts',(-5.82871354320694,7.33735630198543,13.7058703777662));
#83818=CARTESIAN_POINT('Ctrl Pts',(-5.75365614288103,7.39635991566899,13.7042334301289));
#83819=CARTESIAN_POINT('Ctrl Pts',(-5.47134176914888,7.61139277225039,13.6981163713023));
#83820=CARTESIAN_POINT('Ctrl Pts',(-5.25853540764957,7.75994105164088,13.6935806175734));
#83821=CARTESIAN_POINT('Ctrl Pts',(-4.78490249907385,8.06211771660023,13.6837104485165));
#83822=CARTESIAN_POINT('Ctrl Pts',(-4.52223913675435,8.21233143266858,13.6783726615362));
#83823=CARTESIAN_POINT('Ctrl Pts',(-4.20524620297512,8.37378852487856,13.6722325124629));
#83824=CARTESIAN_POINT('Ctrl Pts',(-4.15751321550853,8.39758975934428,13.6713158948368));
#83825=CARTESIAN_POINT('Ctrl Pts',(-4.07148282404111,8.43957402324355,13.6696797521683));
#83826=CARTESIAN_POINT('Ctrl Pts',(-4.03326036959856,8.4579071222804,13.668958498521));
#83827=CARTESIAN_POINT('Ctrl Pts',(-3.94553406769704,8.49925444428757,13.6673163981042));
#83828=CARTESIAN_POINT('Ctrl Pts',(-3.89595097587032,8.52209664343502,13.6663976042258));
#83829=CARTESIAN_POINT('Ctrl Pts',(-3.70089060088279,8.60989993093465,13.6628144775688));
#83830=CARTESIAN_POINT('Ctrl Pts',(-3.55396547309669,8.67157988848993,13.6601831845256));
#83831=CARTESIAN_POINT('Ctrl Pts',(-3.02974909658397,8.87608674710629,13.6509321499499));
#83832=CARTESIAN_POINT('Ctrl Pts',(-2.64488564121107,8.99827071226635,13.6443685991963));
#83833=CARTESIAN_POINT('Ctrl Pts',(-2.1574835876537,9.11902428057033,13.6359792982354));
#83834=CARTESIAN_POINT('Ctrl Pts',(-2.06124918664057,9.14125762625234,13.6343204519353));
#83835=CARTESIAN_POINT('Ctrl Pts',(-1.88756472396255,9.17850232539342,13.631319006617));
#83836=CARTESIAN_POINT('Ctrl Pts',(-1.8102423634587,9.19406482881105,13.6299801483228));
#83837=CARTESIAN_POINT('Ctrl Pts',(-1.63765413609716,9.22653965598941,13.6269848413324));
#83838=CARTESIAN_POINT('Ctrl Pts',(-1.54230420375037,9.24295638718684,13.6253253495142));
#83839=CARTESIAN_POINT('Ctrl Pts',(-1.39055284394043,9.26667034765137,13.6226768121504));
#83840=CARTESIAN_POINT('Ctrl Pts',(-1.33430969910463,9.27493580352531,13.6216935997887));
#83841=CARTESIAN_POINT('Ctrl Pts',(-1.19900741971246,9.29356355473358,13.6193248381689));
#83842=CARTESIAN_POINT('Ctrl Pts',(-1.11988446667426,9.30342953395587,13.617936755534));
#83843=CARTESIAN_POINT('Ctrl Pts',(-0.771594301594879,9.34235086819596,
13.6118172990465));
#83844=CARTESIAN_POINT('Ctrl Pts',(-0.501366810691159,9.36074293800375,
13.6070410959149));
#83845=CARTESIAN_POINT('Ctrl Pts',(-0.0707876889876929,9.37134831852746,
13.5994875825991));
#83846=CARTESIAN_POINT('Ctrl Pts',(0.0892237044766844,9.3711909369757,13.5966940444714));
#83847=CARTESIAN_POINT('Ctrl Pts',(0.303562747941404,9.3654896971273,13.5929988984837));
#83848=CARTESIAN_POINT('Ctrl Pts',(0.357959227598983,9.36356838061255,13.5920652172544));
#83849=CARTESIAN_POINT('Ctrl Pts',(0.450334831579198,9.3594994694455,13.5904883042248));
#83850=CARTESIAN_POINT('Ctrl Pts',(0.488323042781744,9.35759436977103,13.5898424226135));
#83851=CARTESIAN_POINT('Ctrl Pts',(0.585353674315503,9.35213583389683,13.5881990380156));
#83852=CARTESIAN_POINT('Ctrl Pts',(0.64437588747053,9.34825455996213,13.587205186828));
#83853=CARTESIAN_POINT('Ctrl Pts',(0.741139622399783,9.34097065095967,13.5855827060884));
#83854=CARTESIAN_POINT('Ctrl Pts',(0.778904206077944,9.33789745523028,13.5849512155016));
#83855=CARTESIAN_POINT('Ctrl Pts',(0.925824708121688,9.325043925158,13.5824996066932));
#83856=CARTESIAN_POINT('Ctrl Pts',(1.03482449804371,9.3135779338721,13.5806917763604));
#83857=CARTESIAN_POINT('Ctrl Pts',(1.46760170511265,9.26036154279829,13.5735225127501));
#83858=CARTESIAN_POINT('Ctrl Pts',(1.78930156091811,9.20361618019595,13.5682045452544));
#83859=CARTESIAN_POINT('Ctrl Pts',(2.23876338725272,9.09987384593492,13.5605580647563));
#83860=CARTESIAN_POINT('Ctrl Pts',(2.369473878563,9.06671709686617,13.5583091919493));
#83861=CARTESIAN_POINT('Ctrl Pts',(2.57948071776047,9.00859392337947,13.5546454349429));
#83862=CARTESIAN_POINT('Ctrl Pts',(2.65924012028335,8.9853729579693,13.5532420754153));
#83863=CARTESIAN_POINT('Ctrl Pts',(2.81800442582266,8.93685158160099,13.5504232560687));
#83864=CARTESIAN_POINT('Ctrl Pts',(2.89700323087115,8.91155639475026,13.5490079416203));
#83865=CARTESIAN_POINT('Ctrl Pts',(3.10273509008446,8.84265686678181,13.5452880202451));
#83866=CARTESIAN_POINT('Ctrl Pts',(3.22888655714876,8.79737670857217,13.5429726688563));
#83867=CARTESIAN_POINT('Ctrl Pts',(3.5210834338707,8.68536510333768,13.53753254773));
#83868=CARTESIAN_POINT('Ctrl Pts',(3.68627499020414,8.61655220993656,13.5343972276331));
#83869=CARTESIAN_POINT('Ctrl Pts',(3.99842497119523,8.47590125834029,13.5283814288471));
#83870=CARTESIAN_POINT('Ctrl Pts',(4.14565216786008,8.40487107718726,13.5255038955705));
#83871=CARTESIAN_POINT('Ctrl Pts',(4.29092664483271,8.33003803059534,13.5226410022223));
#83872=CARTESIAN_POINT('',(-9.37024987374761,-0.000112039410554904,13.6510063850557));
#83873=CARTESIAN_POINT('Ctrl Pts',(4.29092662791762,8.33003803930856,13.3252837277684));
#83874=CARTESIAN_POINT('Ctrl Pts',(4.25433914434803,8.34888479688114,13.3259751586246));
#83875=CARTESIAN_POINT('Ctrl Pts',(4.21762732641183,8.36749058838333,13.3266682295477));
#83876=CARTESIAN_POINT('Ctrl Pts',(4.11001364099518,8.42114172422255,13.3286980998132));
#83877=CARTESIAN_POINT('Ctrl Pts',(4.03878991457186,8.45553168409844,13.3300394013147));
#83878=CARTESIAN_POINT('Ctrl Pts',(3.88295348583062,8.52835812967984,13.3329705620834));
#83879=CARTESIAN_POINT('Ctrl Pts',(3.79818706397135,8.56644588695825,13.3345627067117));
#83880=CARTESIAN_POINT('Ctrl Pts',(3.51333351220943,8.6893786974053,13.3399059043401));
#83881=CARTESIAN_POINT('Ctrl Pts',(3.3108640048278,8.76852287938427,13.3436937119541));
#83882=CARTESIAN_POINT('Ctrl Pts',(2.8807517340493,8.91962812301239,13.3516877117272));
#83883=CARTESIAN_POINT('Ctrl Pts',(2.65273902985008,8.9900763044122,13.3558960421617));
#83884=CARTESIAN_POINT('Ctrl Pts',(2.29803065092168,9.08499782782943,13.3623198403822));
#83885=CARTESIAN_POINT('Ctrl Pts',(2.17310234121991,9.11568739968306,13.3645587888549));
#83886=CARTESIAN_POINT('Ctrl Pts',(1.99611700393168,9.1553199506668,13.3676814064442));
#83887=CARTESIAN_POINT('Ctrl Pts',(1.94455584931509,9.16640982381599,13.3685852419767));
#83888=CARTESIAN_POINT('Ctrl Pts',(1.85531382107322,9.18481729852027,13.3701378910811));
#83889=CARTESIAN_POINT('Ctrl Pts',(1.81767668326768,9.19233972702623,13.3707890017838));
#83890=CARTESIAN_POINT('Ctrl Pts',(1.71820388056441,9.21158626296818,13.372500725644));
#83891=CARTESIAN_POINT('Ctrl Pts',(1.65629445430179,9.22291899359172,13.3735569462511));
#83892=CARTESIAN_POINT('Ctrl Pts',(1.51652562678216,9.24705144006855,13.3759253234861));
#83893=CARTESIAN_POINT('Ctrl Pts',(1.43860920456866,9.25949317755083,13.3772343595031));
#83894=CARTESIAN_POINT('Ctrl Pts',(1.17029444650478,9.29886932455034,13.3817155947945));
#83895=CARTESIAN_POINT('Ctrl Pts',(0.979229412805784,9.32092644435171,13.3848616491889));
#83896=CARTESIAN_POINT('Ctrl Pts',(0.635871400396342,9.34989007814254,13.390510587555));
#83897=CARTESIAN_POINT('Ctrl Pts',(0.483832263893323,9.35898943108613,13.3930100647453));
#83898=CARTESIAN_POINT('Ctrl Pts',(0.171616570313395,9.37004654132625,13.3981701871388));
#83899=CARTESIAN_POINT('Ctrl Pts',(0.0114753247046249,9.37161098934903,
13.4008317258371));
#83900=CARTESIAN_POINT('Ctrl Pts',(-0.235314128884163,9.36769602938699,
13.4049736159322));
#83901=CARTESIAN_POINT('Ctrl Pts',(-0.321978008241194,9.36511781864869,
13.406435648632));
#83902=CARTESIAN_POINT('Ctrl Pts',(-0.489080552862117,9.357824308307,13.4092711335111));
#83903=CARTESIAN_POINT('Ctrl Pts',(-0.56951884636652,9.35327342806366,13.4106434099543));
#83904=CARTESIAN_POINT('Ctrl Pts',(-0.766973779805546,9.33954557521882,
13.4140308856371));
#83905=CARTESIAN_POINT('Ctrl Pts',(-0.883895705368397,9.32920621531617,
13.4160531862818));
#83906=CARTESIAN_POINT('Ctrl Pts',(-1.14444585285477,9.30122364509327,13.4205950135276));
#83907=CARTESIAN_POINT('Ctrl Pts',(-1.28792203176478,9.28244441389174,13.4231202465825));
#83908=CARTESIAN_POINT('Ctrl Pts',(-1.77496948206278,9.2071860483114,13.4317572321618));
#83909=CARTESIAN_POINT('Ctrl Pts',(-2.11580271625539,9.13488753207197,13.4379213658748));
#83910=CARTESIAN_POINT('Ctrl Pts',(-2.51590364716088,9.02641802794577,13.445093518079));
#83911=CARTESIAN_POINT('Ctrl Pts',(-2.57980068845243,9.0083640032538,13.4462365482159));
#83912=CARTESIAN_POINT('Ctrl Pts',(-2.68438407198202,8.97761010597331,13.448100592264));
#83913=CARTESIAN_POINT('Ctrl Pts',(-2.72518514955378,8.96530908456337,13.4488260173978));
#83914=CARTESIAN_POINT('Ctrl Pts',(-2.81674254388668,8.93702288651081,13.4504492977752));
#83915=CARTESIAN_POINT('Ctrl Pts',(-2.86744935859713,8.92088285012275,13.4513453995999));
#83916=CARTESIAN_POINT('Ctrl Pts',(-3.05411120213506,8.85971223272662,13.4546376995935));
#83917=CARTESIAN_POINT('Ctrl Pts',(-3.18916641099927,8.81199829225072,13.4570073764402));
#83918=CARTESIAN_POINT('Ctrl Pts',(-3.63963761670756,8.6411371821161,13.4649387472786));
#83919=CARTESIAN_POINT('Ctrl Pts',(-3.94945969166991,8.50399802181716,13.4704483143879));
#83920=CARTESIAN_POINT('Ctrl Pts',(-4.37440080033387,8.28766080376121,13.4783483641807));
#83921=CARTESIAN_POINT('Ctrl Pts',(-4.4962185495701,8.22220910492731,13.4806533717839));
#83922=CARTESIAN_POINT('Ctrl Pts',(-4.68927174158877,8.1129095002676,13.4843822928311));
#83923=CARTESIAN_POINT('Ctrl Pts',(-4.76144623391158,8.07076203021758,13.4857938321148));
#83924=CARTESIAN_POINT('Ctrl Pts',(-4.90370752894744,7.98511366048696,13.4886126039226));
#83925=CARTESIAN_POINT('Ctrl Pts',(-4.97380307506328,7.94164155779215,13.4900195251673));
#83926=CARTESIAN_POINT('Ctrl Pts',(-5.15359399022164,7.82682408025446,13.4936759768804));
#83927=CARTESIAN_POINT('Ctrl Pts',(-5.26238501085859,7.75409634032873,13.4959355242761));
#83928=CARTESIAN_POINT('Ctrl Pts',(-5.51054458422183,7.58057087901413,13.5011969569443));
#83929=CARTESIAN_POINT('Ctrl Pts',(-5.64873244267406,7.47816675660149,13.504208304193));
#83930=CARTESIAN_POINT('Ctrl Pts',(-6.02629836797052,7.18193170602994,13.5126377322141));
#83931=CARTESIAN_POINT('Ctrl Pts',(-6.2590553988498,6.98001725548903,13.5180755394343));
#83932=CARTESIAN_POINT('Ctrl Pts',(-6.52045378298172,6.72964967995398,13.5243245926291));
#83933=CARTESIAN_POINT('Ctrl Pts',(-6.55913643633165,6.69195274769418,13.5252530369555));
#83934=CARTESIAN_POINT('Ctrl Pts',(-6.62765443832374,6.62401585158094,13.5269025077077));
#83935=CARTESIAN_POINT('Ctrl Pts',(-6.65761412518977,6.59390351270326,13.5276253769656));
#83936=CARTESIAN_POINT('Ctrl Pts',(-6.70652647631659,6.5440687451038,13.5288079280013));
#83937=CARTESIAN_POINT('Ctrl Pts',(-6.72559924420123,6.52446533648689,13.5292697246983));
#83938=CARTESIAN_POINT('Ctrl Pts',(-6.74588871697685,6.50342786556879,13.529761878767));
#83939=CARTESIAN_POINT('Ctrl Pts',(-6.74719110455674,6.50207665158473,13.5297934742631));
#83940=CARTESIAN_POINT('Ctrl Pts',(-6.74986273210688,6.4993031978665,13.5298582953334));
#83941=CARTESIAN_POINT('Ctrl Pts',(-6.7512319287222,6.49788091647469,13.5298915202851));
#83942=CARTESIAN_POINT('Ctrl Pts',(-6.75404628966078,6.49495559086128,13.529959822912));
#83943=CARTESIAN_POINT('Ctrl Pts',(-6.75549140199688,6.49345249676073,13.5299948998474));
#83944=CARTESIAN_POINT('Ctrl Pts',(-6.75846753347835,6.49035488613068,13.5300671494523));
#83945=CARTESIAN_POINT('Ctrl Pts',(-6.75999849034144,6.4887603099193,13.5301043212438));
#83946=CARTESIAN_POINT('Ctrl Pts',(-6.76315719485408,6.48546801333634,13.5301810269608));
#83947=CARTESIAN_POINT('Ctrl Pts',(-6.76478486786365,6.48377022154854,13.5302205598446));
#83948=CARTESIAN_POINT('Ctrl Pts',(-6.76814896026576,6.48025856115504,13.5303022807183));
#83949=CARTESIAN_POINT('Ctrl Pts',(-6.7698852901399,6.47844460701169,13.5303444674724));
#83950=CARTESIAN_POINT('Ctrl Pts',(-6.77211693355532,6.47611131897801,13.5303986986174));
#83951=CARTESIAN_POINT('Ctrl Pts',(-6.77261291676864,6.47559262594246,13.5304107521363));
#83952=CARTESIAN_POINT('Ctrl Pts',(-6.77370170220674,6.47445372584381,13.5304372134979));
#83953=CARTESIAN_POINT('Ctrl Pts',(-6.77429447885283,6.47383349433359,13.530451620993));
#83954=CARTESIAN_POINT('Ctrl Pts',(-6.77559762132539,6.47246962094165,13.5304832960176));
#83955=CARTESIAN_POINT('Ctrl Pts',(-6.77630794992216,6.47172594351342,13.5305005630431));
#83956=CARTESIAN_POINT('Ctrl Pts',(-6.77787205860917,6.47008786250413,13.5305385871085));
#83957=CARTESIAN_POINT('Ctrl Pts',(-6.7787257841355,6.46919340682398,13.5305593434135));
#83958=CARTESIAN_POINT('Ctrl Pts',(-6.78060907252633,6.46721948702191,13.5306051353573));
#83959=CARTESIAN_POINT('Ctrl Pts',(-6.78163855472392,6.46613994596658,13.5306301699158));
#83960=CARTESIAN_POINT('Ctrl Pts',(-6.78391412917726,6.46375257985646,13.5306855127569));
#83961=CARTESIAN_POINT('Ctrl Pts',(-6.78516010114829,6.4624446401836,13.5307158194399));
#83962=CARTESIAN_POINT('Ctrl Pts',(-6.78792022660939,6.45954556327803,13.5307829653193));
#83963=CARTESIAN_POINT('Ctrl Pts',(-6.78943419904825,6.45795425376123,13.5308198021282));
#83964=CARTESIAN_POINT('Ctrl Pts',(-6.79279577912509,6.45441846801403,13.5309016075294));
#83965=CARTESIAN_POINT('Ctrl Pts',(-6.79464311168072,6.45247373044106,13.5309465725318));
#83966=CARTESIAN_POINT('Ctrl Pts',(-6.79875460407693,6.44814172622635,13.5310466696401));
#83967=CARTESIAN_POINT('Ctrl Pts',(-6.80101834215558,6.44575405966016,13.5311017963118));
#83968=CARTESIAN_POINT('Ctrl Pts',(-6.8060682203297,6.4404221037233,13.5312248040075));
#83969=CARTESIAN_POINT('Ctrl Pts',(-6.80885370850797,6.43747719763367,13.5312926767637));
#83970=CARTESIAN_POINT('Ctrl Pts',(-6.81508028691074,6.43088569982227,13.5314444481101));
#83971=CARTESIAN_POINT('Ctrl Pts',(-6.81852036315749,6.427238151682,13.5315283340916));
#83972=CARTESIAN_POINT('Ctrl Pts',(-6.82622218909576,6.41905868397918,13.5317162230106));
#83973=CARTESIAN_POINT('Ctrl Pts',(-6.83048235678544,6.41452527759748,13.5318202067563));
#83974=CARTESIAN_POINT('Ctrl Pts',(-6.83581736602381,6.4088367501763,13.5319504973718));
#83975=CARTESIAN_POINT('Ctrl Pts',(-6.83689643411496,6.40768559631603,13.5319768538595));
#83976=CARTESIAN_POINT('Ctrl Pts',(-6.83991637373446,6.40446228216286,13.5320506269842));
#83977=CARTESIAN_POINT('Ctrl Pts',(-6.84185659370975,6.40238951286484,13.5320980360213));
#83978=CARTESIAN_POINT('Ctrl Pts',(-6.84727134802902,6.39659956842215,13.5322303789693));
#83979=CARTESIAN_POINT('Ctrl Pts',(-6.85074379732056,6.3928804443511,13.5323152889368));
#83980=CARTESIAN_POINT('Ctrl Pts',(-6.8603721072006,6.38255130806522,13.5325508365931));
#83981=CARTESIAN_POINT('Ctrl Pts',(-6.86652144271549,6.37593521972591,13.5327014013063));
#83982=CARTESIAN_POINT('Ctrl Pts',(-6.93615342164577,6.30080039642089,13.5344078235381));
#83983=CARTESIAN_POINT('Ctrl Pts',(-6.99861778938336,6.23134488018772,13.5359528434712));
#83984=CARTESIAN_POINT('Ctrl Pts',(-7.24561567658521,5.94830273481953,13.5421431376852));
#83985=CARTESIAN_POINT('Ctrl Pts',(-7.42149442495577,5.72736176771968,13.5467423619323));
#83986=CARTESIAN_POINT('Ctrl Pts',(-7.69108316605216,5.355390062222,13.5543121666704));
#83987=CARTESIAN_POINT('Ctrl Pts',(-7.79094626176988,5.20904204871112,13.5572487189054));
#83988=CARTESIAN_POINT('Ctrl Pts',(-7.93564574326462,4.98350886893447,13.5617375451873));
#83989=CARTESIAN_POINT('Ctrl Pts',(-7.98357661967185,4.9063569293355,13.56326670701));
#83990=CARTESIAN_POINT('Ctrl Pts',(-8.0607747123919,4.77796773001299,13.5658029458229));
#83991=CARTESIAN_POINT('Ctrl Pts',(-8.09069311721066,4.72712909301443,13.5668050708216));
#83992=CARTESIAN_POINT('Ctrl Pts',(-8.15750155968644,4.61111286571039,13.5690875019796));
#83993=CARTESIAN_POINT('Ctrl Pts',(-8.19409423277976,4.54576871744796,13.5703698976355));
#83994=CARTESIAN_POINT('Ctrl Pts',(-8.2753842187533,4.39643624774469,13.5732936553552));
#83995=CARTESIAN_POINT('Ctrl Pts',(-8.31959361320003,4.31219175204795,13.5749381984306));
#83996=CARTESIAN_POINT('Ctrl Pts',(-8.43663871818134,4.08065064213426,13.5794432985791));
#83997=CARTESIAN_POINT('Ctrl Pts',(-8.50689503605345,3.93208839828071,13.5823181862141));
#83998=CARTESIAN_POINT('Ctrl Pts',(-8.70144067558025,3.4910551139186,13.5907809104323));
#83999=CARTESIAN_POINT('Ctrl Pts',(-8.81480414028925,3.19402000867285,13.5963957164846));
#84000=CARTESIAN_POINT('Ctrl Pts',(-8.93197983695458,2.83287127004801,13.6029556739764));
#84001=CARTESIAN_POINT('Ctrl Pts',(-8.95051508756268,2.77375253638042,13.6040208854829));
#84002=CARTESIAN_POINT('Ctrl Pts',(-8.98069810694544,2.67402888723112,13.6058008279254));
#84003=CARTESIAN_POINT('Ctrl Pts',(-8.99266003679972,2.63352130335847,13.6065190684839));
#84004=CARTESIAN_POINT('Ctrl Pts',(-9.01571346782891,2.55346484677153,13.6079290138334));
#84005=CARTESIAN_POINT('Ctrl Pts',(-9.02681957508127,2.51392132425797,13.6086210345943));
#84006=CARTESIAN_POINT('Ctrl Pts',(-9.06586012559356,2.37132156994564,13.61110265384));
#84007=CARTESIAN_POINT('Ctrl Pts',(-9.09229265372062,2.26786247488045,13.612877129768));
#84008=CARTESIAN_POINT('Ctrl Pts',(-9.1726701409767,1.92922735115369,13.6186296391887));
#84009=CARTESIAN_POINT('Ctrl Pts',(-9.21930174663869,1.69241584346927,13.6225678326773));
#84010=CARTESIAN_POINT('Ctrl Pts',(-9.29374705406242,1.21848989243408,13.6304422903755));
#84011=CARTESIAN_POINT('Ctrl Pts',(-9.32174570217052,0.981584683065158,
13.6343752900242));
#84012=CARTESIAN_POINT('Ctrl Pts',(-9.34803975904847,0.651413976895667,
13.6399165415983));
#84013=CARTESIAN_POINT('Ctrl Pts',(-9.35402963813424,0.558853275222426,
13.6414761429096));
#84014=CARTESIAN_POINT('Ctrl Pts',(-9.36253092642073,0.388202739958158,
13.6443654091715));
#84015=CARTESIAN_POINT('Ctrl Pts',(-9.36544175453,0.310140976588955,13.6456923957318));
#84016=CARTESIAN_POINT('Ctrl Pts',(-9.36929292215148,0.154678726856719,
13.6483465531186));
#84017=CARTESIAN_POINT('Ctrl Pts',(-9.37025092521758,0.0772847412573868,
13.649673507729));
#84018=CARTESIAN_POINT('Ctrl Pts',(-9.37024999932951,-0.000112095055203477,
13.6510061684742));
#84019=CARTESIAN_POINT('Ctrl Pts',(-9.37024999933013,-0.000112043156642308,
13.6510061675806));
#84020=CARTESIAN_POINT('Ctrl Pts',(-9.3702488395512,-0.0971051916695123,
13.6526762482647));
#84021=CARTESIAN_POINT('Ctrl Pts',(-9.36874168983789,-0.194092347865134,
13.6543551374663));
#84022=CARTESIAN_POINT('Ctrl Pts',(-9.35727739558263,-0.563017704195856,
13.6607723877306));
#84023=CARTESIAN_POINT('Ctrl Pts',(-9.33698236069871,-0.834499158935258,
13.6655627546302));
#84024=CARTESIAN_POINT('Ctrl Pts',(-9.28821281498095,-1.24528170400177,
13.6728319962421));
#84025=CARTESIAN_POINT('Ctrl Pts',(-9.26834038644242,-1.38545674867222,
13.6753153670229));
#84026=CARTESIAN_POINT('Ctrl Pts',(-9.23433930152131,-1.59157077577059,
13.6789514452263));
#84027=CARTESIAN_POINT('Ctrl Pts',(-9.22266274298759,-1.65789379164598,
13.680119019226));
#84028=CARTESIAN_POINT('Ctrl Pts',(-9.20210088476301,-1.76773772935149,
13.6820458455685));
#84029=CARTESIAN_POINT('Ctrl Pts',(-9.19361926202526,-1.81133162275184,
13.6828087302879));
#84030=CARTESIAN_POINT('Ctrl Pts',(-9.17665669737404,-1.89532606738809,
13.6842740739909));
#84031=CARTESIAN_POINT('Ctrl Pts',(-9.16821806360247,-1.93573412450207,
13.6849769243828));
#84032=CARTESIAN_POINT('Ctrl Pts',(-9.1485064433321,-2.02710104929343,13.6865608217591));
#84033=CARTESIAN_POINT('Ctrl Pts',(-9.13707419514622,-2.07802405580281,
13.6874400801842));
#84034=CARTESIAN_POINT('Ctrl Pts',(-9.09652690156851,-2.25182823997268,
13.690432805628));
#84035=CARTESIAN_POINT('Ctrl Pts',(-9.06535349208769,-2.37421530471821,
13.6925261731818));
#84036=CARTESIAN_POINT('Ctrl Pts',(-8.9680224060908,-2.72641465877341,13.6985511172254));
#84037=CARTESIAN_POINT('Ctrl Pts',(-8.89552976691311,-2.95437188039995,
13.702453500911));
#84038=CARTESIAN_POINT('Ctrl Pts',(-8.73978894374367,-3.38615207178213,
13.7099950089209));
#84039=CARTESIAN_POINT('Ctrl Pts',(-8.65792305638591,-3.5903070277325,13.7136275092206));
#84040=CARTESIAN_POINT('Ctrl Pts',(-8.53260618597959,-3.87353655356323,
13.7188113975454));
#84041=CARTESIAN_POINT('Ctrl Pts',(-8.49508156019532,-3.95515397870763,
13.7203223247542));
#84042=CARTESIAN_POINT('Ctrl Pts',(-8.42516410698837,-4.10163988209509,
13.7230674668507));
#84043=CARTESIAN_POINT('Ctrl Pts',(-8.39318082495865,-4.16669600109397,
13.7242987057597));
#84044=CARTESIAN_POINT('Ctrl Pts',(-8.31763183327126,-4.3159674212755,13.7271526156484));
#84045=CARTESIAN_POINT('Ctrl Pts',(-8.27353638210375,-4.39990565492697,
13.7287789468099));
#84046=CARTESIAN_POINT('Ctrl Pts',(-8.05299790657777,-4.80467128592429,
13.7367269244048));
#84047=CARTESIAN_POINT('Ctrl Pts',(-7.85912786791901,-5.11563760000234,
13.7431734173052));
#84048=CARTESIAN_POINT('Ctrl Pts',(-7.56927819585957,-5.52503098289925,
13.7519857710494));
#84049=CARTESIAN_POINT('Ctrl Pts',(-7.48860440561291,-5.63389243082866,
13.7543611222191));
#84050=CARTESIAN_POINT('Ctrl Pts',(-7.36531764093396,-5.79292702966547,
13.7578620449607));
#84051=CARTESIAN_POINT('Ctrl Pts',(-7.32449091579521,-5.84446236802974,
13.7590014404581));
#84052=CARTESIAN_POINT('Ctrl Pts',(-7.25553149641298,-5.92965185922325,
13.7608904811255));
#84053=CARTESIAN_POINT('Ctrl Pts',(-7.22769881137141,-5.96354578823632,
13.7616435645954));
#84054=CARTESIAN_POINT('Ctrl Pts',(-7.19084388313023,-6.00778975364928,
13.7626279164477));
#84055=CARTESIAN_POINT('Ctrl Pts',(-7.18203542694448,-6.01831709051949,
13.7628622290497));
#84056=CARTESIAN_POINT('Ctrl Pts',(-7.14583761409164,-6.06138589571277,
13.7638211676936));
#84057=CARTESIAN_POINT('Ctrl Pts',(-7.11825003917088,-6.09375996931984,
13.7645426017951));
#84058=CARTESIAN_POINT('Ctrl Pts',(-7.05486366659474,-6.16712619217975,
13.7661796906556));
#84059=CARTESIAN_POINT('Ctrl Pts',(-7.01892625268463,-6.20799654486537,
13.7670933757751));
#84060=CARTESIAN_POINT('Ctrl Pts',(-6.7951602908998,-6.45805065350713,13.772701764963));
#84061=CARTESIAN_POINT('Ctrl Pts',(-6.59835168244718,-6.65900727849565,
13.7772929655006));
#84062=CARTESIAN_POINT('Ctrl Pts',(-6.19073253694149,-7.03937538634662,
13.7864335172351));
#84063=CARTESIAN_POINT('Ctrl Pts',(-5.98041546821213,-7.21890610815664,
13.7909780570726));
#84064=CARTESIAN_POINT('Ctrl Pts',(-5.68674279324379,-7.44793692484547,
13.7972054426393));
#84065=CARTESIAN_POINT('Ctrl Pts',(-5.61011036175369,-7.50582904846296,
13.7988197056933));
#84066=CARTESIAN_POINT('Ctrl Pts',(-5.46893391151629,-7.60911098911496,
13.8017771181343));
#84067=CARTESIAN_POINT('Ctrl Pts',(-5.40468054243189,-7.65488317179611,
13.8031170710849));
#84068=CARTESIAN_POINT('Ctrl Pts',(-5.25804851565517,-7.75657284362428,
13.8061623786707));
#84069=CARTESIAN_POINT('Ctrl Pts',(-5.17534124270567,-7.81199970732012,
13.8078713206606));
#84070=CARTESIAN_POINT('Ctrl Pts',(-4.7596988949833,-8.08104718565987,13.8164162478065));
#84071=CARTESIAN_POINT('Ctrl Pts',(-4.41435408850214,-8.27475268583837,
13.8233990795122));
#84072=CARTESIAN_POINT('Ctrl Pts',(-3.90989542643503,-8.51711398219828,
13.8332160880435));
#84073=CARTESIAN_POINT('Ctrl Pts',(-3.76014205512594,-8.58427893381587,
13.8360823078156));
#84074=CARTESIAN_POINT('Ctrl Pts',(-3.55799656371564,-8.66863681984948,
13.8398570956303));
#84075=CARTESIAN_POINT('Ctrl Pts',(-3.50710581689088,-8.68935053209578,
13.8407995335197));
#84076=CARTESIAN_POINT('Ctrl Pts',(-3.41667362048382,-8.72523465420003,
13.8424585232164));
#84077=CARTESIAN_POINT('Ctrl Pts',(-3.37720621963715,-8.74058673958096,
13.8431771410749));
#84078=CARTESIAN_POINT('Ctrl Pts',(-3.27822944408186,-8.77831639459607,
13.8449664362186));
#84079=CARTESIAN_POINT('Ctrl Pts',(-3.21859394449918,-8.80035681431302,
13.8460331901405));
#84080=CARTESIAN_POINT('Ctrl Pts',(-2.98775606263299,-8.88301086273159,
13.850126468475));
#84081=CARTESIAN_POINT('Ctrl Pts',(-2.81502917382757,-8.93924937499039,
13.853114253816));
#84082=CARTESIAN_POINT('Ctrl Pts',(-2.40764319637441,-9.05891163475776,
13.8600807134449));
#84083=CARTESIAN_POINT('Ctrl Pts',(-2.17193396774468,-9.11829636181049,
13.8640517689999));
#84084=CARTESIAN_POINT('Ctrl Pts',(-1.82261311485674,-9.19198936923752,
13.8699496450467));
#84085=CARTESIAN_POINT('Ctrl Pts',(-1.71062202561537,-9.21348790309958,
13.8718419071577));
#84086=CARTESIAN_POINT('Ctrl Pts',(-1.49949240640433,-9.25003547556912,
13.8754201945896));
#84087=CARTESIAN_POINT('Ctrl Pts',(-1.40045027589751,-9.26554762206088,
13.8771032457719));
#84088=CARTESIAN_POINT('Ctrl Pts',(-1.22376658372984,-9.29032242952756,
13.8801169522891));
#84089=CARTESIAN_POINT('Ctrl Pts',(-1.14622196893779,-9.30020809774215,
13.8814434576106));
#84090=CARTESIAN_POINT('Ctrl Pts',(-0.974101705526609,-9.31996520418596,
13.8843972734573));
#84091=CARTESIAN_POINT('Ctrl Pts',(-0.87948115784808,-9.32936966655224,
13.8860274224552));
#84092=CARTESIAN_POINT('Ctrl Pts',(-0.411906267705348,-9.36866589391062,
13.8941143850369));
#84093=CARTESIAN_POINT('Ctrl Pts',(-0.0375377533519839,-9.37764125779603,
13.9007032140654));
#84094=CARTESIAN_POINT('Ctrl Pts',(0.530470229929351,-9.35723858627385,
13.910687297424));
#84095=CARTESIAN_POINT('Ctrl Pts',(0.724317669826966,-9.34423227924921,
13.9140890615151));
#84096=CARTESIAN_POINT('Ctrl Pts',(0.973991234309995,-9.31966386376122,
13.9184154491261));
#84097=CARTESIAN_POINT('Ctrl Pts',(1.03031031349024,-9.31360586110844,13.9193876386048));
#84098=CARTESIAN_POINT('Ctrl Pts',(1.1284880250913,-9.30214388292615,13.9210739559138));
#84099=CARTESIAN_POINT('Ctrl Pts',(1.1703712791237,-9.2969670923339,13.9217905062967));
#84100=CARTESIAN_POINT('Ctrl Pts',(1.27298962079049,-9.28357897025028,13.9235395637917));
#84101=CARTESIAN_POINT('Ctrl Pts',(1.33368174977877,-9.27505439803486,13.9245686187555));
#84102=CARTESIAN_POINT('Ctrl Pts',(1.66110742052958,-9.22578521844333,13.9301006027028));
#84103=CARTESIAN_POINT('Ctrl Pts',(1.92607114230827,-9.17412893969969,13.9345104140168));
#84104=CARTESIAN_POINT('Ctrl Pts',(2.45141032152367,-9.04794549424095,13.9433670959542));
#84105=CARTESIAN_POINT('Ctrl Pts',(2.71152595300367,-8.97342502698393,13.9478102729578));
#84106=CARTESIAN_POINT('Ctrl Pts',(3.06426236312623,-8.8556292745728,13.9540186405165));
#84107=CARTESIAN_POINT('Ctrl Pts',(3.15994399790798,-8.82194012349555,13.9557211508394));
#84108=CARTESIAN_POINT('Ctrl Pts',(3.3290995586658,-8.75927596397847,13.9587675531186));
#84109=CARTESIAN_POINT('Ctrl Pts',(3.40278973355542,-8.73091296945605,13.9601071747271));
#84110=CARTESIAN_POINT('Ctrl Pts',(3.56387414860746,-8.66656317947355,13.9630641893285));
#84111=CARTESIAN_POINT('Ctrl Pts',(3.6511002022442,-8.63017865095102,13.9646841845423));
#84112=CARTESIAN_POINT('Ctrl Pts',(4.0928654372712,-8.43800915099113,13.972985525147));
#84113=CARTESIAN_POINT('Ctrl Pts',(4.43805154466072,-8.26167303368647,13.9798103564765));
#84114=CARTESIAN_POINT('Ctrl Pts',(4.92969813772146,-7.97079169099115,13.9898410155151));
#84115=CARTESIAN_POINT('Ctrl Pts',(5.08527017036665,-7.87245016012284,13.993060849823));
#84116=CARTESIAN_POINT('Ctrl Pts',(5.28441488240712,-7.7381973806287,13.9972018092981));
#84117=CARTESIAN_POINT('Ctrl Pts',(5.33070084992959,-7.70638487354804,13.9981656001143));
#84118=CARTESIAN_POINT('Ctrl Pts',(5.41128651810698,-7.64992463386581,13.9998440371506));
#84119=CARTESIAN_POINT('Ctrl Pts',(5.44571059389155,-7.62545767918514,14.0005610059473));
#84120=CARTESIAN_POINT('Ctrl Pts',(5.53017262909851,-7.56456253831623,14.0023205816138));
#84121=CARTESIAN_POINT('Ctrl Pts',(5.58001722997495,-7.52786978116809,14.0033596116509));
#84122=CARTESIAN_POINT('Ctrl Pts',(5.83940258885416,-7.33293322436741,14.0087794992078));
#84123=CARTESIAN_POINT('Ctrl Pts',(6.04258754219039,-7.16642651979467,14.0130729547129));
#84124=CARTESIAN_POINT('Ctrl Pts',(6.44999944221824,-6.80289865363994,14.0220231254108));
#84125=CARTESIAN_POINT('Ctrl Pts',(6.65281593973745,-6.60469245245984,14.0266781392838));
#84126=CARTESIAN_POINT('Ctrl Pts',(6.91380466829742,-6.32539763868048,14.0330644744242));
#84127=CARTESIAN_POINT('Ctrl Pts',(6.98012755157119,-6.25213320242099,14.034724232765));
#84128=CARTESIAN_POINT('Ctrl Pts',(7.09727898347821,-6.11853223684106,14.0377266047631));
#84129=CARTESIAN_POINT('Ctrl Pts',(7.14852801491084,-6.05857680392513,14.0390654666562));
#84130=CARTESIAN_POINT('Ctrl Pts',(7.26091022182691,-5.9236912495488,14.0420598927709));
#84131=CARTESIAN_POINT('Ctrl Pts',(7.3216527215268,-5.84844736953184,14.0437184901695));
#84132=CARTESIAN_POINT('Ctrl Pts',(7.53089780984262,-5.58087809637662,14.0495756486846));
#84133=CARTESIAN_POINT('Ctrl Pts',(7.67307420248443,-5.38373046035281,14.0538211947711));
#84134=CARTESIAN_POINT('Ctrl Pts',(7.95181649890856,-4.96370691945652,14.0626739870144));
#84135=CARTESIAN_POINT('Ctrl Pts',(8.08704835178767,-4.7401920944263,14.0672809942824));
#84136=CARTESIAN_POINT('Ctrl Pts',(8.23335724525742,-4.47383977677964,14.0725662094236));
#84137=CARTESIAN_POINT('Ctrl Pts',(8.25368952862727,-4.43621720024175,14.0733080496746));
#84138=CARTESIAN_POINT('Ctrl Pts',(8.30398373691876,-4.34161074761176,14.0751606629056));
#84139=CARTESIAN_POINT('Ctrl Pts',(8.33361731162677,-4.28445472821126,14.0762683510741));
#84140=CARTESIAN_POINT('Ctrl Pts',(8.38179337469239,-4.1891435795849,14.0780937440536));
#84141=CARTESIAN_POINT('Ctrl Pts',(8.40066995091835,-4.1511598981866,14.0788154501327));
#84142=CARTESIAN_POINT('Ctrl Pts',(8.44317316453484,-4.0641570969368,14.0804550654945));
#84143=CARTESIAN_POINT('Ctrl Pts',(8.46663195944546,-4.01505781731479,14.0813709598252));
#84144=CARTESIAN_POINT('Ctrl Pts',(8.55359693070508,-3.82888826466691,14.0848131214733));
#84145=CARTESIAN_POINT('Ctrl Pts',(8.61421307191322,-3.69049308303046,14.0873100183094));
#84146=CARTESIAN_POINT('Ctrl Pts',(8.77682263964054,-3.29337005745303,14.0943690361267));
#84147=CARTESIAN_POINT('Ctrl Pts',(8.87068213815949,-3.03148488040831,14.0989026590275));
#84148=CARTESIAN_POINT('Ctrl Pts',(9.00261858105593,-2.60441539438768,14.106277952206));
#84149=CARTESIAN_POINT('Ctrl Pts',(9.04810650261124,-2.44169804349248,14.1090828817782));
#84150=CARTESIAN_POINT('Ctrl Pts',(9.11052904981039,-2.19261599338061,14.113389709835));
#84151=CARTESIAN_POINT('Ctrl Pts',(9.13068745996118,-2.10709537645805,14.1148706167864));
#84152=CARTESIAN_POINT('Ctrl Pts',(9.16692374633916,-1.94306810944073,14.1177171346256));
#84153=CARTESIAN_POINT('Ctrl Pts',(9.18320314125478,-1.86461381532694,14.119081289081));
#84154=CARTESIAN_POINT('Ctrl Pts',(9.21667915248794,-1.69219778039077,14.1220858188662));
#84155=CARTESIAN_POINT('Ctrl Pts',(9.23344924686129,-1.59816234354427,14.123728760266));
#84156=CARTESIAN_POINT('Ctrl Pts',(9.27289931150107,-1.35554778126336,14.1279780411825));
#84157=CARTESIAN_POINT('Ctrl Pts',(9.29344754055521,-1.20664993231808,14.1305961902874));
#84158=CARTESIAN_POINT('Ctrl Pts',(9.3132197589559,-1.03254285440637,14.1336636038634));
#84159=CARTESIAN_POINT('Ctrl Pts',(9.31593491146598,-1.00775182936722,14.1341005010924));
#84160=CARTESIAN_POINT('Ctrl Pts',(9.3448111886594,-0.733999359204234,14.1389259176537));
#84161=CARTESIAN_POINT('Ctrl Pts',(9.3610844354928,-0.484096357613643,14.1433433977092));
#84162=CARTESIAN_POINT('Ctrl Pts',(9.36955204471279,-0.144898352261821,
14.149276784836));
#84163=CARTESIAN_POINT('Ctrl Pts',(9.37050549716812,-0.0559269650014783,
14.1508269401777));
#84164=CARTESIAN_POINT('Ctrl Pts',(9.3699502470512,0.101520915351514,14.1535526357441));
#84165=CARTESIAN_POINT('Ctrl Pts',(9.36895814132929,0.169992668069073,14.1547321204751));
#84166=CARTESIAN_POINT('Ctrl Pts',(9.36612498950733,0.281290733248407,14.1566366368255));
#84167=CARTESIAN_POINT('Ctrl Pts',(9.36474047270412,0.32412605040461,14.1573665048075));
#84168=CARTESIAN_POINT('Ctrl Pts',(9.36102048436284,0.419044783592841,14.1589762348358));
#84169=CARTESIAN_POINT('Ctrl Pts',(9.35854411329062,0.471121147066671,14.1598545829335));
#84170=CARTESIAN_POINT('Ctrl Pts',(9.34873889424838,0.64646242697372,14.1627994941332));
#84171=CARTESIAN_POINT('Ctrl Pts',(9.33940814390406,0.769602657850774,14.1648469957626));
#84172=CARTESIAN_POINT('Ctrl Pts',(9.2988415187647,1.19355954943503,14.1718712139198));
#84173=CARTESIAN_POINT('Ctrl Pts',(9.25548015963627,1.49302562623371,14.1767946298674));
#84174=CARTESIAN_POINT('Ctrl Pts',(9.18169541596998,1.87218780738994,14.18316402135));
#84175=CARTESIAN_POINT('Ctrl Pts',(9.16457205598315,1.95428680130627,14.1845509462329));
#84176=CARTESIAN_POINT('Ctrl Pts',(9.13357936896066,2.09350574812983,14.186919457915));
#84177=CARTESIAN_POINT('Ctrl Pts',(9.1202704541596,2.15074527503112,14.187898074138));
#84178=CARTESIAN_POINT('Ctrl Pts',(9.0831273777399,2.30394396110407,14.1905316590833));
#84179=CARTESIAN_POINT('Ctrl Pts',(9.05831142265086,2.39965723480705,14.1921922824883));
#84180=CARTESIAN_POINT('Ctrl Pts',(9.01098471015623,2.57098432400586,14.1951955301113));
#84181=CARTESIAN_POINT('Ctrl Pts',(8.98902495323411,2.6467406744008,14.1965343920573));
#84182=CARTESIAN_POINT('Ctrl Pts',(8.93803365229024,2.8146900901836,14.1995279718484));
#84183=CARTESIAN_POINT('Ctrl Pts',(8.90852680445793,2.90672943133771,14.2011857133898));
#84184=CARTESIAN_POINT('Ctrl Pts',(8.75897239000766,3.3495424961027,14.2092450097335));
#84185=CARTESIAN_POINT('Ctrl Pts',(8.61960232405398,3.69343815297207,14.2157747011192));
#84186=CARTESIAN_POINT('Ctrl Pts',(8.37720385009096,4.20253959151443,14.2256791512094));
#84187=CARTESIAN_POINT('Ctrl Pts',(8.28880911021248,4.37430305825597,14.2290611951622));
#84188=CARTESIAN_POINT('Ctrl Pts',(8.16772926763208,4.59271016896832,14.233367575451));
#84189=CARTESIAN_POINT('Ctrl Pts',(8.13984085144974,4.64195853262973,14.2343389341716));
#84190=CARTESIAN_POINT('Ctrl Pts',(8.09037949166492,4.72748621960444,14.2360244666473));
#84191=CARTESIAN_POINT('Ctrl Pts',(8.06900452681866,4.76387785604273,14.2367410530863));
#84192=CARTESIAN_POINT('Ctrl Pts',(8.01595898686053,4.85280844276493,14.2384911239669));
#84193=CARTESIAN_POINT('Ctrl Pts',(7.98401698954685,4.90518307472376,14.2395211441924));
#84194=CARTESIAN_POINT('Ctrl Pts',(7.7966041232852,5.20579896216548,14.2454395942777));
#84195=CARTESIAN_POINT('Ctrl Pts',(7.63007535076783,5.44695604864743,14.2502180831965));
#84196=CARTESIAN_POINT('Ctrl Pts',(7.34446345513417,5.8217026768721,14.257945259275));
#84197=CARTESIAN_POINT('Ctrl Pts',(7.23237792301404,5.96037540087566,14.2608753367251));
#84198=CARTESIAN_POINT('Ctrl Pts',(7.07530787708384,6.14374433227486,14.2648784138511));
#84199=CARTESIAN_POINT('Ctrl Pts',(7.03372646838804,6.19130583399345,14.2659288374536));
#84200=CARTESIAN_POINT('Ctrl Pts',(6.92263394212747,6.31581157447978,14.2687127816063));
#84201=CARTESIAN_POINT('Ctrl Pts',(6.85232123332965,6.39202864401884,14.2704522117669));
#84202=CARTESIAN_POINT('Ctrl Pts',(6.72617230220585,6.52429663206588,14.2735376890089));
#84203=CARTESIAN_POINT('Ctrl Pts',(6.67086401812933,6.58083684648114,14.2748790172971));
#84204=CARTESIAN_POINT('Ctrl Pts',(6.54904381618991,6.70225646738273,14.277809876534));
#84205=CARTESIAN_POINT('Ctrl Pts',(6.48226928993804,6.76686053200486,14.2794016890251));
#84206=CARTESIAN_POINT('Ctrl Pts',(6.25875292759917,6.97676669420283,14.2846824856896));
#84207=CARTESIAN_POINT('Ctrl Pts',(6.09800125886097,7.11769919408694,14.28840670949));
#84208=CARTESIAN_POINT('Ctrl Pts',(5.74040957320299,7.41018991821878,14.2965061155114));
#84209=CARTESIAN_POINT('Ctrl Pts',(5.5420765222233,7.55966959651852,14.3008867212513));
#84210=CARTESIAN_POINT('Ctrl Pts',(5.26517628984571,7.75160397355025,14.306778053449));
#84211=CARTESIAN_POINT('Ctrl Pts',(5.19159691751922,7.80107473482848,14.3083226731288));
#84212=CARTESIAN_POINT('Ctrl Pts',(5.06010362839054,7.88679925441331,14.3110399292378));
#84213=CARTESIAN_POINT('Ctrl Pts',(5.00247442135708,7.92347782893592,14.3122164771855));
#84214=CARTESIAN_POINT('Ctrl Pts',(4.90806201162543,7.98212674103074,14.3141177138571));
#84215=CARTESIAN_POINT('Ctrl Pts',(4.87152017484449,8.00448069694584,14.314847204581));
#84216=CARTESIAN_POINT('Ctrl Pts',(4.79009800143786,8.05352548169367,14.3164579180339));
#84217=CARTESIAN_POINT('Ctrl Pts',(4.74514534138318,8.08009327007958,14.3173376085199));
#84218=CARTESIAN_POINT('Ctrl Pts',(4.59384622702819,8.16781555331623,14.3202702504623));
#84219=CARTESIAN_POINT('Ctrl Pts',(4.48652115299682,8.22725726828478,14.3223044718701));
#84220=CARTESIAN_POINT('Ctrl Pts',(4.34909343642689,8.299882210852,14.3248682218991));
#84221=CARTESIAN_POINT('Ctrl Pts',(4.32004864042978,8.31503685704886,14.3254077642749));
#84222=CARTESIAN_POINT('Ctrl Pts',(4.29092662550047,8.33003804055367,14.3259466798393));
#84223=CARTESIAN_POINT('Origin',(0.,0.,2.15141010809499));
#84224=CARTESIAN_POINT('',(4.29092662820214,8.330038039162,15.5233208859591));
#84225=CARTESIAN_POINT('',(4.29092660882816,8.33003804914182,15.3259008099036));
#84226=CARTESIAN_POINT('',(4.29092662815669,8.33003803918541,2.15141010809499));
#84227=CARTESIAN_POINT('',(-9.37025014160435,-4.63021129950685E-5,14.8481494226183));
#84228=CARTESIAN_POINT('Ctrl Pts',(4.29092662820214,8.330038039162,15.5233208859591));
#84229=CARTESIAN_POINT('Ctrl Pts',(4.33935081577568,8.30509401910726,15.5224026034553));
#84230=CARTESIAN_POINT('Ctrl Pts',(4.38755686544741,8.27972807481678,15.5214813896534));
#84231=CARTESIAN_POINT('Ctrl Pts',(4.50754295733572,8.2152494349333,15.5191702036362));
#84232=CARTESIAN_POINT('Ctrl Pts',(4.5790371221348,8.17561531550437,15.517776531901));
#84233=CARTESIAN_POINT('Ctrl Pts',(4.75923231172826,8.07261556020889,15.5142208310236));
#84234=CARTESIAN_POINT('Ctrl Pts',(4.86719237865973,8.00798678832569,15.5120499065674));
#84235=CARTESIAN_POINT('Ctrl Pts',(5.0459017858884,7.89605563927071,15.5083892081614));
#84236=CARTESIAN_POINT('Ctrl Pts',(5.11736736903765,7.8499280678712,15.5069068274078));
#84237=CARTESIAN_POINT('Ctrl Pts',(5.44855282337396,7.62971901269379,15.4999546733999));
#84238=CARTESIAN_POINT('Ctrl Pts',(5.70008238239256,7.44368190771533,15.4944268838185));
#84239=CARTESIAN_POINT('Ctrl Pts',(6.02999976377421,7.17312254237613,15.4869753909228));
#84240=CARTESIAN_POINT('Ctrl Pts',(6.11683257009331,7.09922133635338,15.4849947019738));
#84241=CARTESIAN_POINT('Ctrl Pts',(6.24021474873496,6.99026924087005,15.4821636193275));
#84242=CARTESIAN_POINT('Ctrl Pts',(6.27786250450247,6.95647802841728,15.4812974748673));
#84243=CARTESIAN_POINT('Ctrl Pts',(6.34725010961787,6.89317627459973,15.4796983208853));
#84244=CARTESIAN_POINT('Ctrl Pts',(6.37906234436655,6.86374727904147,15.4789642024782));
#84245=CARTESIAN_POINT('Ctrl Pts',(6.46320769282369,6.7848154358819,15.4770184824566));
#84246=CARTESIAN_POINT('Ctrl Pts',(6.51517613150117,6.73492792778792,15.4758125673697));
#84247=CARTESIAN_POINT('Ctrl Pts',(6.6348602640968,6.61735445414581,15.4730187587819));
#84248=CARTESIAN_POINT('Ctrl Pts',(6.70212417354252,6.54921997759249,15.4714358714828));
#84249=CARTESIAN_POINT('Ctrl Pts',(6.97662312607475,6.26250994682324,15.4648975382805));
#84250=CARTESIAN_POINT('Ctrl Pts',(7.17430341899172,6.03503702676669,15.4599923135375));
#84251=CARTESIAN_POINT('Ctrl Pts',(7.46337372856823,5.66808391348065,15.4522819256152));
#84252=CARTESIAN_POINT('Ctrl Pts',(7.56258128798143,5.53502363960272,15.4495255390682));
#84253=CARTESIAN_POINT('Ctrl Pts',(7.70860770660702,5.32790803044528,15.4452744539986));
#84254=CARTESIAN_POINT('Ctrl Pts',(7.75800899646399,5.25571433029615,15.4437998234166));
#84255=CARTESIAN_POINT('Ctrl Pts',(7.85078361579663,5.11597721535241,15.4409571854984));
#84256=CARTESIAN_POINT('Ctrl Pts',(7.89431416618906,5.04854732176828,15.4395905430191));
#84257=CARTESIAN_POINT('Ctrl Pts',(7.99810124856001,4.88315343516171,15.4362498024808));
#84258=CARTESIAN_POINT('Ctrl Pts',(8.0574307707709,4.78462332153161,15.4342690870405));
#84259=CARTESIAN_POINT('Ctrl Pts',(8.15191612657592,4.62096528971853,15.4309953821624));
#84260=CARTESIAN_POINT('Ctrl Pts',(8.18814084867399,4.55646860669659,15.4297093190472));
#84261=CARTESIAN_POINT('Ctrl Pts',(8.33561394386875,4.2864594783281,15.4243444427109));
#84262=CARTESIAN_POINT('Ctrl Pts',(8.43991826323459,4.07725078992402,15.4202309488007));
#84263=CARTESIAN_POINT('Ctrl Pts',(8.57547336090902,3.77781256878966,15.4144545626041));
#84264=CARTESIAN_POINT('Ctrl Pts',(8.61333593996565,3.69067137232837,15.4127867276333));
#84265=CARTESIAN_POINT('Ctrl Pts',(8.69855566968307,3.48607921000245,15.4089104043076));
#84266=CARTESIAN_POINT('Ctrl Pts',(8.74487023235722,3.36821373453112,15.4067070338864));
#84267=CARTESIAN_POINT('Ctrl Pts',(8.80690215932029,3.20043586511774,15.40362797199));
#84268=CARTESIAN_POINT('Ctrl Pts',(8.82461216202641,3.15127523024656,15.4027326645201));
#84269=CARTESIAN_POINT('Ctrl Pts',(8.85608776180026,3.06155659512679,15.4011128316326));
#84270=CARTESIAN_POINT('Ctrl Pts',(8.86998820694999,3.02104757272192,15.4003868204502));
#84271=CARTESIAN_POINT('Ctrl Pts',(8.90531397794677,2.91575442730613,15.3985125285794));
#84272=CARTESIAN_POINT('Ctrl Pts',(8.92631027422995,2.85082897538292,15.3973691332845));
#84273=CARTESIAN_POINT('Ctrl Pts',(8.97291138126556,2.70116308632557,15.3947560261009));
#84274=CARTESIAN_POINT('Ctrl Pts',(8.99802827712394,2.61627747889864,15.3932904692535));
#84275=CARTESIAN_POINT('Ctrl Pts',(9.08874712726964,2.29290957289445,15.3877514901989));
#84276=CARTESIAN_POINT('Ctrl Pts',(9.14610071108229,2.0522184935753,15.3837163239251));
#84277=CARTESIAN_POINT('Ctrl Pts',(9.20263711253572,1.76496990078625,15.3789049621883));
#84278=CARTESIAN_POINT('Ctrl Pts',(9.21108532995398,1.72033590238561,15.378157568222));
#84279=CARTESIAN_POINT('Ctrl Pts',(9.25165391299683,1.4971317965843,15.3744191913772));
#84280=CARTESIAN_POINT('Ctrl Pts',(9.27890753717816,1.3177171056856,15.3714107107534));
#84281=CARTESIAN_POINT('Ctrl Pts',(9.31178783815821,1.04889604943718,15.3668713480873));
#84282=CARTESIAN_POINT('Ctrl Pts',(9.3213702803212,0.960016518343662,15.3653655449496));
#84283=CARTESIAN_POINT('Ctrl Pts',(9.33708638277133,0.791676790400857,15.3625019975769));
#84284=CARTESIAN_POINT('Ctrl Pts',(9.34348092839117,0.712248808982456,15.3611460599758));
#84285=CARTESIAN_POINT('Ctrl Pts',(9.35630024015266,0.522843592754961,15.3579003228717));
#84286=CARTESIAN_POINT('Ctrl Pts',(9.36180018442812,0.412815728414672,15.3560048774186));
#84287=CARTESIAN_POINT('Ctrl Pts',(9.36960160727936,0.171457652376472,15.3518259888494));
#84288=CARTESIAN_POINT('Ctrl Pts',(9.37108435235863,0.0401241521074494,
15.3495383777897));
#84289=CARTESIAN_POINT('Ctrl Pts',(9.36628490606437,-0.452983999286923,
15.3409106620924));
#84290=CARTESIAN_POINT('Ctrl Pts',(9.34181261882488,-0.814262715226743,
15.3344996789749));
#84291=CARTESIAN_POINT('Ctrl Pts',(9.28715851549517,-1.24733834440628,15.3269306623763));
#84292=CARTESIAN_POINT('Ctrl Pts',(9.27691856474018,-1.3213433396882,15.3256419266638));
#84293=CARTESIAN_POINT('Ctrl Pts',(9.25991983117765,-1.43423377531867,15.3236869620909));
#84294=CARTESIAN_POINT('Ctrl Pts',(9.25379857205968,-1.47321207019614,15.3230139685745));
#84295=CARTESIAN_POINT('Ctrl Pts',(9.23976889032109,-1.55900942102823,15.3215378638506));
#84296=CARTESIAN_POINT('Ctrl Pts',(9.23175041975164,-1.6058093665504,15.3207360657735));
#84297=CARTESIAN_POINT('Ctrl Pts',(9.20618895917069,-1.74847584563897,15.3182995616863));
#84298=CARTESIAN_POINT('Ctrl Pts',(9.18750575039273,-1.84413153076017,15.3166765496582));
#84299=CARTESIAN_POINT('Ctrl Pts',(9.11373699811146,-2.19281432008148,15.3107744611561));
#84300=CARTESIAN_POINT('Ctrl Pts',(9.04966192038923,-2.44382004581928,15.3065500884788));
#84301=CARTESIAN_POINT('Ctrl Pts',(8.90794165483375,-2.91634949553053,15.2984525425213));
#84302=CARTESIAN_POINT('Ctrl Pts',(8.83221064078816,-3.13824371771744,15.2945872632762));
#84303=CARTESIAN_POINT('Ctrl Pts',(8.71394455913219,-3.44643566001338,15.2890669377829));
#84304=CARTESIAN_POINT('Ctrl Pts',(8.67828149669257,-3.53527633230051,15.2874577450569));
#84305=CARTESIAN_POINT('Ctrl Pts',(8.61380597216685,-3.68903418287639,15.2846386608485));
#84306=CARTESIAN_POINT('Ctrl Pts',(8.58560507004405,-3.75419926020087,15.2834330868386));
#84307=CARTESIAN_POINT('Ctrl Pts',(8.5177079037643,-3.90632486886088,15.2805924913161));
#84308=CARTESIAN_POINT('Ctrl Pts',(8.47741621957076,-3.99301090612813,15.2789534373301));
#84309=CARTESIAN_POINT('Ctrl Pts',(8.32156185013121,-4.31532915353274,15.272782004556));
#84310=CARTESIAN_POINT('Ctrl Pts',(8.19744350193355,-4.54668850934292,15.2681924599812));
#84311=CARTESIAN_POINT('Ctrl Pts',(7.91048751387181,-5.03153593599281,15.2582935960347));
#84312=CARTESIAN_POINT('Ctrl Pts',(7.74480648804397,-5.28300477363558,15.2529821099818));
#84313=CARTESIAN_POINT('Ctrl Pts',(7.5363222263582,-5.56850011965685,15.2468823245477));
#84314=CARTESIAN_POINT('Ctrl Pts',(7.50497621543816,-5.61067538747026,15.2459795401482));
#84315=CARTESIAN_POINT('Ctrl Pts',(7.44775700661573,-5.68632484975614,15.2443587630593));
#84316=CARTESIAN_POINT('Ctrl Pts',(7.42200876565529,-5.71989166203922,15.2436391765799));
#84317=CARTESIAN_POINT('Ctrl Pts',(7.36205630105453,-5.79696251956892,15.2419862623234));
#84318=CARTESIAN_POINT('Ctrl Pts',(7.32769231179728,-5.84034013014577,15.2410551475539));
#84319=CARTESIAN_POINT('Ctrl Pts',(7.18628106290558,-6.01563038867596,15.2372837973001));
#84320=CARTESIAN_POINT('Ctrl Pts',(7.07603979912934,-6.14492518965123,15.2344812515384));
#84321=CARTESIAN_POINT('Ctrl Pts',(6.69035300379286,-6.57312154815875,15.2250135059318));
#84322=CARTESIAN_POINT('Ctrl Pts',(6.39900494690285,-6.85707561528014,15.2183945960659));
#84323=CARTESIAN_POINT('Ctrl Pts',(6.01907309668896,-7.18199760461406,15.2100282214637));
#84324=CARTESIAN_POINT('Ctrl Pts',(5.94709592123443,-7.24171116424869,15.2084551101879));
#84325=CARTESIAN_POINT('Ctrl Pts',(5.81266409366925,-7.34988211675825,15.2055360691962));
#84326=CARTESIAN_POINT('Ctrl Pts',(5.75046682254399,-7.39864597646568,15.2041928247729));
#84327=CARTESIAN_POINT('Ctrl Pts',(5.60597515164211,-7.50900743532391,15.2010880060906));
#84328=CARTESIAN_POINT('Ctrl Pts',(5.52326920004079,-7.57004936155757,15.1993222219529));
#84329=CARTESIAN_POINT('Ctrl Pts',(5.24105648381663,-7.77125174732075,15.193335314287));
#84330=CARTESIAN_POINT('Ctrl Pts',(5.03708944676859,-7.90498298287792,15.1890691484747));
#84331=CARTESIAN_POINT('Ctrl Pts',(4.57742676264317,-8.18134018628447,15.1796454357825));
#84332=CARTESIAN_POINT('Ctrl Pts',(4.31979155718149,-8.32025025313945,15.1744838599681));
#84333=CARTESIAN_POINT('Ctrl Pts',(4.00064797383993,-8.47349881940574,15.1683680291139));
#84334=CARTESIAN_POINT('Ctrl Pts',(3.94495386638531,-8.49957089916678,15.1673109028652));
#84335=CARTESIAN_POINT('Ctrl Pts',(3.85060289873225,-8.54261225784336,15.1655394618291));
#84336=CARTESIAN_POINT('Ctrl Pts',(3.81208082364247,-8.55987188454036,15.1648217310514));
#84337=CARTESIAN_POINT('Ctrl Pts',(3.72174907090171,-8.59961385488393,15.1631517020717));
#84338=CARTESIAN_POINT('Ctrl Pts',(3.66985026084444,-8.62188921773207,15.1622018576813));
#84339=CARTESIAN_POINT('Ctrl Pts',(3.44207158677377,-8.71722426960827,15.1580689763533));
#84340=CARTESIAN_POINT('Ctrl Pts',(3.26418849650919,-8.7853815902678,15.1549335562591));
#84341=CARTESIAN_POINT('Ctrl Pts',(2.74733699008249,-8.96555102199639,15.1459507960855));
#84342=CARTESIAN_POINT('Ctrl Pts',(2.40388622295269,-9.06368007285904,15.1401259874661));
#84343=CARTESIAN_POINT('Ctrl Pts',(1.95640495745719,-9.16430127891586,15.13247203829));
#84344=CARTESIAN_POINT('Ctrl Pts',(1.85677610714491,-9.18500521010514,15.1307648799918));
#84345=CARTESIAN_POINT('Ctrl Pts',(1.67915162220254,-9.21890929897867,15.1277122160855));
#84346=CARTESIAN_POINT('Ctrl Pts',(1.60128874887153,-9.23275219759082,15.1263710207339));
#84347=CARTESIAN_POINT('Ctrl Pts',(1.43149948503482,-9.2607258274759,15.1234387035838));
#84348=CARTESIAN_POINT('Ctrl Pts',(1.33951905329488,-9.27447692751331,15.1218452817024));
#84349=CARTESIAN_POINT('Ctrl Pts',(1.03106221792878,-9.31590681595326,15.1164850990747));
#84350=CARTESIAN_POINT('Ctrl Pts',(0.813826998264375,-9.33739225592145,
15.1126812210327));
#84351=CARTESIAN_POINT('Ctrl Pts',(0.357768902005902,-9.36646094808392,
15.1046674866449));
#84352=CARTESIAN_POINT('Ctrl Pts',(0.119003646567082,-9.37253580038925,
15.1004556988116));
#84353=CARTESIAN_POINT('Ctrl Pts',(-0.247577994081873,-9.36785126926592,
15.0940426829013));
#84354=CARTESIAN_POINT('Ctrl Pts',(-0.375377232773101,-9.36360103526062,
15.0918174741581));
#84355=CARTESIAN_POINT('Ctrl Pts',(-0.555496136424005,-9.35391723791089,
15.0887121957051));
#84356=CARTESIAN_POINT('Ctrl Pts',(-0.607918110990462,-9.35065662069869,
15.0878121606238));
#84357=CARTESIAN_POINT('Ctrl Pts',(-0.702965723866272,-9.34394204004306,
15.0861886842621));
#84358=CARTESIAN_POINT('Ctrl Pts',(-0.745600266551923,-9.3406366965886,
15.0854636975381));
#84359=CARTESIAN_POINT('Ctrl Pts',(-0.855665183063269,-9.33134527720796,
15.083599418309));
#84360=CARTESIAN_POINT('Ctrl Pts',(-0.923056049086309,-9.32492011494468,
15.0824648987653));
#84361=CARTESIAN_POINT('Ctrl Pts',(-1.07739796879355,-9.30851534093726,
15.0798770807735));
#84362=CARTESIAN_POINT('Ctrl Pts',(-1.16429075373411,-9.29804664016778,
15.0784278241706));
#84363=CARTESIAN_POINT('Ctrl Pts',(-1.48971480386679,-9.25420672114131,
15.0730113504534));
#84364=CARTESIAN_POINT('Ctrl Pts',(-1.72707711171348,-9.21286042357409,
15.0690809404721));
#84365=CARTESIAN_POINT('Ctrl Pts',(-2.01670252623431,-9.15082287834424,
15.0642151143947));
#84366=CARTESIAN_POINT('Ctrl Pts',(-2.07071879989919,-9.13875112237347,
15.0633047191856));
#84367=CARTESIAN_POINT('Ctrl Pts',(-2.29832845694405,-9.08576246673031,
15.059453337675));
#84368=CARTESIAN_POINT('Ctrl Pts',(-2.47084160092836,-9.0403724926916,15.0564959515221));
#84369=CARTESIAN_POINT('Ctrl Pts',(-2.72816795555704,-8.96475094425637,
15.0520012975801));
#84370=CARTESIAN_POINT('Ctrl Pts',(-2.8140131811171,-8.93817596912533,15.0504878415896));
#84371=CARTESIAN_POINT('Ctrl Pts',(-2.97513025740711,-8.88574796245285,
15.0476185979804));
#84372=CARTESIAN_POINT('Ctrl Pts',(-3.05048094698526,-8.86016268802724,
15.0462647211034));
#84373=CARTESIAN_POINT('Ctrl Pts',(-3.22838460551438,-8.79721712208813,
15.0430387594063));
#84374=CARTESIAN_POINT('Ctrl Pts',(-3.33062864280929,-8.75901872430125,
15.0411612295487));
#84375=CARTESIAN_POINT('Ctrl Pts',(-3.49572151098055,-8.69403123188319,
15.0380916394055));
#84376=CARTESIAN_POINT('Ctrl Pts',(-3.558985784548,-8.66832556556886,15.0369061873254));
#84377=CARTESIAN_POINT('Ctrl Pts',(-3.80894683168125,-8.56356312493695,
15.0321872949181));
#84378=CARTESIAN_POINT('Ctrl Pts',(-3.99333727966357,-8.47914774197705,
15.0286267220198));
#84379=CARTESIAN_POINT('Ctrl Pts',(-4.39568130863915,-8.27891412341059,
15.020725365523));
#84380=CARTESIAN_POINT('Ctrl Pts',(-4.61209346458263,-8.16033256116785,
15.0163849802468));
#84381=CARTESIAN_POINT('Ctrl Pts',(-4.87760027625507,-8.00091068312191,
15.0110324338467));
#84382=CARTESIAN_POINT('Ctrl Pts',(-4.93129787019399,-7.96792680413757,
15.0099486129987));
#84383=CARTESIAN_POINT('Ctrl Pts',(-5.02048133033249,-7.91189876113124,
15.0081489150559));
#84384=CARTESIAN_POINT('Ctrl Pts',(-5.05615109013546,-7.88915147304997,
15.0074293129255));
#84385=CARTESIAN_POINT('Ctrl Pts',(-5.13811500259475,-7.83609729257674,
15.0057765148429));
#84386=CARTESIAN_POINT('Ctrl Pts',(-5.18429710298221,-7.80562041900588,
15.0048455302148));
#84387=CARTESIAN_POINT('Ctrl Pts',(-5.3710606590213,-7.67998117484013,15.001076323176));
#84388=CARTESIAN_POINT('Ctrl Pts',(-5.50931414247387,-7.58141553172918,
14.9982757355824));
#84389=CARTESIAN_POINT('Ctrl Pts',(-5.96933379448044,-7.23422021752676,
14.9888071174083));
#84390=CARTESIAN_POINT('Ctrl Pts',(-6.27756778527526,-6.96843102223886,
14.9821855266378));
#84391=CARTESIAN_POINT('Ctrl Pts',(-6.63425889966502,-6.61792547708285,
14.9738164439272));
#84392=CARTESIAN_POINT('Ctrl Pts',(-6.69996976496323,-6.55139175010933,
14.9722434870024));
#84393=CARTESIAN_POINT('Ctrl Pts',(-6.81936111007782,-6.4268301034296,14.9693245847937));
#84394=CARTESIAN_POINT('Ctrl Pts',(-6.87332441821854,-6.36908490570559,
14.9679813228595));
#84395=CARTESIAN_POINT('Ctrl Pts',(-6.98842678446998,-6.24274917189362,
14.9650628025681));
#84396=CARTESIAN_POINT('Ctrl Pts',(-7.04930057660508,-6.17392804251074,
14.9634854599055));
#84397=CARTESIAN_POINT('Ctrl Pts',(-7.13641989890285,-6.07246639257281,
14.9611780634694));
#84398=CARTESIAN_POINT('Ctrl Pts',(-7.16347434761205,-6.04052748764616,
14.9604542740297));
#84399=CARTESIAN_POINT('Ctrl Pts',(-7.28159928472947,-5.89916636229705,
14.9572621998112));
#84400=CARTESIAN_POINT('Ctrl Pts',(-7.37038310319124,-5.78785838473884,
14.9547782515122));
#84401=CARTESIAN_POINT('Ctrl Pts',(-7.60020054385354,-5.48586977190057,
14.9481292821605));
#84402=CARTESIAN_POINT('Ctrl Pts',(-7.73658983258874,-5.29178543343197,
14.9439467207313));
#84403=CARTESIAN_POINT('Ctrl Pts',(-7.94339503146362,-4.97238547519062,
14.9372815294534));
#84404=CARTESIAN_POINT('Ctrl Pts',(-8.01854800132615,-4.85026082620992,
14.9347820783155));
#84405=CARTESIAN_POINT('Ctrl Pts',(-8.11753144594043,-4.68081854793995,
14.931401903969));
#84406=CARTESIAN_POINT('Ctrl Pts',(-8.14380709840801,-4.63495253645753,
14.9304955583149));
#84407=CARTESIAN_POINT('Ctrl Pts',(-8.18320258068852,-4.56481560820111,
14.9291240582881));
#84408=CARTESIAN_POINT('Ctrl Pts',(-8.19660558461286,-4.54070511126053,
14.9286551968177));
#84409=CARTESIAN_POINT('Ctrl Pts',(-8.22917363783605,-4.48150475451051,
14.9275103599715));
#84410=CARTESIAN_POINT('Ctrl Pts',(-8.24822091913862,-4.44635078496461,
14.9268359224103));
#84411=CARTESIAN_POINT('Ctrl Pts',(-8.31466112898951,-4.32183149433479,
14.9244641431966));
#84412=CARTESIAN_POINT('Ctrl Pts',(-8.36083148895304,-4.2318216004866,14.9227806193413));
#84413=CARTESIAN_POINT('Ctrl Pts',(-8.44303455798622,-4.06496644788605,
14.9197022744777));
#84414=CARTESIAN_POINT('Ctrl Pts',(-8.47949802155801,-3.98834528359802,
14.9183048100877));
#84415=CARTESIAN_POINT('Ctrl Pts',(-8.65205766662259,-3.61267642319097,
14.9115117630621));
#84416=CARTESIAN_POINT('Ctrl Pts',(-8.77340144976112,-3.30710748288676,
14.9061569370261));
#84417=CARTESIAN_POINT('Ctrl Pts',(-8.91942322996013,-2.87435253332653,
14.8985772359048));
#84418=CARTESIAN_POINT('Ctrl Pts',(-8.9579055098469,-2.75207957634599,14.8964372536469));
#84419=CARTESIAN_POINT('Ctrl Pts',(-9.0146059836085,-2.55811012854314,14.8930371648305));
#84420=CARTESIAN_POINT('Ctrl Pts',(-9.03450441893329,-2.48692145966704,
14.891788239452));
#84421=CARTESIAN_POINT('Ctrl Pts',(-9.0727718210926,-2.34349133834688,14.8892687212566));
#84422=CARTESIAN_POINT('Ctrl Pts',(-9.09112524341568,-2.27125118617137,
14.8879981241305));
#84423=CARTESIAN_POINT('Ctrl Pts',(-9.12776300880281,-2.11947780354789,
14.8853247988519));
#84424=CARTESIAN_POINT('Ctrl Pts',(-9.14587417724437,-2.03990911636392,
14.8839210752183));
#84425=CARTESIAN_POINT('Ctrl Pts',(-9.22487873389747,-1.67058659117372,
14.8773960535077));
#84426=CARTESIAN_POINT('Ctrl Pts',(-9.27305614763012,-1.37828720650158,
14.8721987555121));
#84427=CARTESIAN_POINT('Ctrl Pts',(-9.33415293420309,-0.853801898862271,
14.8629150560277));
#84428=CARTESIAN_POINT('Ctrl Pts',(-9.35242749034445,-0.622486220083037,
14.8588367076895));
#84429=CARTESIAN_POINT('Ctrl Pts',(-9.3647488749212,-0.327260078623795,
14.8537270545419));
#84430=CARTESIAN_POINT('Ctrl Pts',(-9.36675234064347,-0.263763654014486,
14.8526338499193));
#84431=CARTESIAN_POINT('Ctrl Pts',(-9.36884081189437,-0.166061462144396,
14.8509629765942));
#84432=CARTESIAN_POINT('Ctrl Pts',(-9.36938448135584,-0.131867431932818,
14.8503803333988));
#84433=CARTESIAN_POINT('Ctrl Pts',(-9.37008015239402,-0.0651306203950395,
14.8492477688838));
#84434=CARTESIAN_POINT('Ctrl Pts',(-9.37024983919293,-0.032588570022699,
14.8486975781768));
#84435=CARTESIAN_POINT('Ctrl Pts',(-9.37024999988576,-4.62699946108937E-5,
14.8481491766056));
#84436=CARTESIAN_POINT('Ctrl Pts',(-9.37024999988558,-4.63062477912489E-5,
14.8481491772165));
#84437=CARTESIAN_POINT('Ctrl Pts',(-9.37025016016673,0.032387210047458,
14.8476026088632));
#84438=CARTESIAN_POINT('Ctrl Pts',(-9.37008192584371,0.0648205413103381,
14.8470578249882));
#84439=CARTESIAN_POINT('Ctrl Pts',(-9.36929780245289,0.140366629717473,
14.8457924112172));
#84440=CARTESIAN_POINT('Ctrl Pts',(-9.36855272598917,0.183477326384378,
14.8450729797667));
#84441=CARTESIAN_POINT('Ctrl Pts',(-9.36256155825491,0.431169014311936,
14.8409515014231));
#84442=CARTESIAN_POINT('Ctrl Pts',(-9.35091197546653,0.63554016256853,14.8375966945186));
#84443=CARTESIAN_POINT('Ctrl Pts',(-9.31000650999248,1.09035195682257,14.8301116941649));
#84444=CARTESIAN_POINT('Ctrl Pts',(-9.2773173533605,1.34032498169207,14.825983467721));
#84445=CARTESIAN_POINT('Ctrl Pts',(-9.21854480882273,1.68195584608197,14.8202287393192));
#84446=CARTESIAN_POINT('Ctrl Pts',(-9.20108483103443,1.77498781506405,14.8186503810149));
#84447=CARTESIAN_POINT('Ctrl Pts',(-9.1673099459977,1.94103261517819,14.8158093206971));
#84448=CARTESIAN_POINT('Ctrl Pts',(-9.15152444755324,2.01414486010617,14.814549980076));
#84449=CARTESIAN_POINT('Ctrl Pts',(-9.11727783589863,2.16403904591509,14.8119494245596));
#84450=CARTESIAN_POINT('Ctrl Pts',(-9.09871801239683,2.24079241037001,14.8106076588955));
#84451=CARTESIAN_POINT('Ctrl Pts',(-9.05450247207541,2.4140289254047,14.8075552341209));
#84452=CARTESIAN_POINT('Ctrl Pts',(-9.02827049074515,2.51035506438266,14.8058409508684));
#84453=CARTESIAN_POINT('Ctrl Pts',(-8.91216590888784,2.91131522585685,14.798634094877));
#84454=CARTESIAN_POINT('Ctrl Pts',(-8.80837422098841,3.2116972951539,14.7930544204129));
#84455=CARTESIAN_POINT('Ctrl Pts',(-8.63030217313856,3.653015846571,14.7846881166589));
#84456=CARTESIAN_POINT('Ctrl Pts',(-8.56736252369659,3.79828117371726,14.7819073399662));
#84457=CARTESIAN_POINT('Ctrl Pts',(-8.47070038269466,4.00673563098657,14.7779035477802));
#84458=CARTESIAN_POINT('Ctrl Pts',(-8.4398861570895,4.07124269412026,14.7766627327093));
#84459=CARTESIAN_POINT('Ctrl Pts',(-8.38455397178697,4.18374757192508,14.7744990100095));
#84460=CARTESIAN_POINT('Ctrl Pts',(-8.36035443240386,4.23189825408347,14.7735730814653));
#84461=CARTESIAN_POINT('Ctrl Pts',(-8.3304346079049,4.29017240575354,14.7724537844061));
#84462=CARTESIAN_POINT('Ctrl Pts',(-8.32510914963593,4.30049737524762,14.7722555185418));
#84463=CARTESIAN_POINT('Ctrl Pts',(-8.30052497412412,4.34794424393631,14.7713446947745));
#84464=CARTESIAN_POINT('Ctrl Pts',(-8.28103712268044,4.38494676906722,14.7706353079543));
#84465=CARTESIAN_POINT('Ctrl Pts',(-8.23173478286286,4.47705855580376,14.7688709866335));
#84466=CARTESIAN_POINT('Ctrl Pts',(-8.2016140212376,4.53200157987228,14.7678198419312));
#84467=CARTESIAN_POINT('Ctrl Pts',(-8.0635371416166,4.77798096631243,14.7631110000088));
#84468=CARTESIAN_POINT('Ctrl Pts',(-7.94944151650463,4.96549227394637,14.7595120048732));
#84469=CARTESIAN_POINT('Ctrl Pts',(-7.70888392173955,5.33126381070386,14.7523355753741));
#84470=CARTESIAN_POINT('Ctrl Pts',(-7.58255894241874,5.50945232116996,14.7487601897487));
#84471=CARTESIAN_POINT('Ctrl Pts',(-7.38410509968045,5.76961229989866,14.7433485562269));
#84472=CARTESIAN_POINT('Ctrl Pts',(-7.3165821598779,5.85500295849619,14.7415400788273));
#84473=CARTESIAN_POINT('Ctrl Pts',(-7.19789848197688,5.99983233225335,14.7384101950405));
#84474=CARTESIAN_POINT('Ctrl Pts',(-7.1474511249961,6.05984100096852,14.7370942558684));
#84475=CARTESIAN_POINT('Ctrl Pts',(-7.04636934006488,6.17706240065272,14.734483773726));
#84476=CARTESIAN_POINT('Ctrl Pts',(-6.99577636210066,6.23430299546772,14.7331896416136));
#84477=CARTESIAN_POINT('Ctrl Pts',(-6.88501087086556,6.35657604047414,14.7303817997884));
#84478=CARTESIAN_POINT('Ctrl Pts',(-6.82460449781062,6.42138669226045,14.7288661594031));
#84479=CARTESIAN_POINT('Ctrl Pts',(-6.64233222177486,6.61147104829941,14.7243380358121));
#84480=CARTESIAN_POINT('Ctrl Pts',(-6.5178713035553,6.73420226328853,14.7213038271286));
#84481=CARTESIAN_POINT('Ctrl Pts',(-6.29190752288132,6.94488955315872,14.7159047195832));
#84482=CARTESIAN_POINT('Ctrl Pts',(-6.19180926871345,7.03427957149033,14.7135487994992));
#84483=CARTESIAN_POINT('Ctrl Pts',(-5.94579009655439,7.24465888683698,14.7078587022797));
#84484=CARTESIAN_POINT('Ctrl Pts',(-5.7980504584273,7.36343080644468,14.7045225426141));
#84485=CARTESIAN_POINT('Ctrl Pts',(-5.58429191104298,7.52485259018563,14.6998477731187));
#84486=CARTESIAN_POINT('Ctrl Pts',(-5.52118313442434,7.57127858974637,14.6984857403366));
#84487=CARTESIAN_POINT('Ctrl Pts',(-5.40659596619699,7.65338007166294,14.6960497051497));
#84488=CARTESIAN_POINT('Ctrl Pts',(-5.35532798436316,7.68934123764587,14.6949728205539));
#84489=CARTESIAN_POINT('Ctrl Pts',(-5.27209128272421,7.74649010615319,14.6932476986284));
#84490=CARTESIAN_POINT('Ctrl Pts',(-5.24034631436417,7.76800012730232,14.6925952067104));
#84491=CARTESIAN_POINT('Ctrl Pts',(-5.16446878294425,7.81873704859955,14.6910488448522));
#84492=CARTESIAN_POINT('Ctrl Pts',(-5.12021891757649,7.84778599976995,14.6901573638823));
#84493=CARTESIAN_POINT('Ctrl Pts',(-4.96712621598174,7.9464415680789,14.6871043888964));
#84494=CARTESIAN_POINT('Ctrl Pts',(-4.85709114600769,8.01417133611161,14.6849638226828));
#84495=CARTESIAN_POINT('Ctrl Pts',(-4.66310339031397,8.12811328731931,14.6812558365575));
#84496=CARTESIAN_POINT('Ctrl Pts',(-4.57977716083409,8.17535320487262,14.679683637225));
#84497=CARTESIAN_POINT('Ctrl Pts',(-4.29359779329665,8.3318475864602,14.6743350245929));
#84498=CARTESIAN_POINT('Ctrl Pts',(-4.08744615058297,8.43489478694661,14.670566181726));
#84499=CARTESIAN_POINT('Ctrl Pts',(-3.77623673975164,8.57636548957207,14.6649156068853));
#84500=CARTESIAN_POINT('Ctrl Pts',(-3.67395178675623,8.62067788066451,14.6630648746156));
#84501=CARTESIAN_POINT('Ctrl Pts',(-3.47962571686501,8.7007779294017,14.6595532010026));
#84502=CARTESIAN_POINT('Ctrl Pts',(-3.38776186047385,8.73695606154295,14.6578949802547));
#84503=CARTESIAN_POINT('Ctrl Pts',(-3.2215125181812,8.79941262404106,14.6548941671624));
#84504=CARTESIAN_POINT('Ctrl Pts',(-3.14733425013258,8.8262162061279,14.6535553079421));
#84505=CARTESIAN_POINT('Ctrl Pts',(-2.98139592767012,8.88381845089406,14.6505593833357));
#84506=CARTESIAN_POINT('Ctrl Pts',(-2.88947922730363,8.9141383027309,14.6488992679234));
#84507=CARTESIAN_POINT('Ctrl Pts',(-2.55683799549484,9.01817844156007,14.6428891652543));
#84508=CARTESIAN_POINT('Ctrl Pts',(-2.31363638457182,9.08361430133465,14.6384879564239));
#84509=CARTESIAN_POINT('Ctrl Pts',(-2.02586832571781,9.14873308876972,14.6333050892782));
#84510=CARTESIAN_POINT('Ctrl Pts',(-1.98357433715222,9.15799609361822,14.6325440689058));
#84511=CARTESIAN_POINT('Ctrl Pts',(-1.76436540003371,9.20441628115723,14.6286047910578));
#84512=CARTESIAN_POINT('Ctrl Pts',(-1.58646624535125,9.23674127075432,14.6254241521223));
#84513=CARTESIAN_POINT('Ctrl Pts',(-1.33208108117045,9.27539767696573,14.6209353588839));
#84514=CARTESIAN_POINT('Ctrl Pts',(-1.25628044552962,9.2859679920136,14.6196053665935));
#84515=CARTESIAN_POINT('Ctrl Pts',(-1.11925918377197,9.30336698687795,14.6172192598907));
#84516=CARTESIAN_POINT('Ctrl Pts',(-1.05808450070686,9.31052284392828,14.6161604317797));
#84517=CARTESIAN_POINT('Ctrl Pts',(-0.954866776683514,9.32156621647971,
14.6143872062694));
#84518=CARTESIAN_POINT('Ctrl Pts',(-0.912860102034708,9.32577362677442,
14.6136693731625));
#84519=CARTESIAN_POINT('Ctrl Pts',(-0.815681048787701,9.33484423928135,
14.6120176879915));
#84520=CARTESIAN_POINT('Ctrl Pts',(-0.760491246312097,9.33950242936874,
14.6110860649273));
#84521=CARTESIAN_POINT('Ctrl Pts',(-0.526056044526549,9.35719767436545,
14.6071502532815));
#84522=CARTESIAN_POINT('Ctrl Pts',(-0.346496114815447,9.36556587242737,
14.6041884291376));
#84523=CARTESIAN_POINT('Ctrl Pts',(0.0886052375417247,9.37331264770265,
14.5970431134733));
#84524=CARTESIAN_POINT('Ctrl Pts',(0.344095864972601,9.36741367288125,14.5928719316847));
#84525=CARTESIAN_POINT('Ctrl Pts',(0.715194620127776,9.34364127931472,14.586731659203));
#84526=CARTESIAN_POINT('Ctrl Pts',(0.831214765062937,9.33403544221045,14.5848008479602));
#84527=CARTESIAN_POINT('Ctrl Pts',(1.0481475003125,9.31199780124703,14.5811608818815));
#84528=CARTESIAN_POINT('Ctrl Pts',(1.14909538516653,9.30008042771529,14.5794549434649));
#84529=CARTESIAN_POINT('Ctrl Pts',(1.32809077750361,9.27599028476565,14.5764049540663));
#84530=CARTESIAN_POINT('Ctrl Pts',(1.40621595242587,9.26446855129081,14.5750652150476));
#84531=CARTESIAN_POINT('Ctrl Pts',(1.57734076495685,9.23701695855951,14.572110860953));
#84532=CARTESIAN_POINT('Ctrl Pts',(1.6702643192013,9.22066717917013,14.5704936753074));
#84533=CARTESIAN_POINT('Ctrl Pts',(2.18261586985526,9.12252032692422,14.5615050151998));
#84534=CARTESIAN_POINT('Ctrl Pts',(2.59631456429605,9.01350850611793,14.553952755));
#84535=CARTESIAN_POINT('Ctrl Pts',(3.1432999897111,8.82857721398656,14.5438341908778));
#84536=CARTESIAN_POINT('Ctrl Pts',(3.2843034278182,8.77709870381412,14.5412163785394));
#84537=CARTESIAN_POINT('Ctrl Pts',(3.47412330407415,8.70258299118752,14.5377037727648));
#84538=CARTESIAN_POINT('Ctrl Pts',(3.52406654396406,8.68247882011976,14.5367807183511));
#84539=CARTESIAN_POINT('Ctrl Pts',(3.61312345621974,8.64573481026152,14.5351385426375));
#84540=CARTESIAN_POINT('Ctrl Pts',(3.65230225720898,8.62925719524365,14.5344175898242));
#84541=CARTESIAN_POINT('Ctrl Pts',(3.74118399425694,8.59116202478304,14.532784688199));
#84542=CARTESIAN_POINT('Ctrl Pts',(3.79081419107952,8.56937864729061,14.5318746711408));
#84543=CARTESIAN_POINT('Ctrl Pts',(3.99240531836963,8.47880349360051,14.5281805499157));
#84544=CARTESIAN_POINT('Ctrl Pts',(4.14268294627997,8.40640056746697,14.5254314779371));
#84545=CARTESIAN_POINT('Ctrl Pts',(4.29092664592494,8.33003803003272,14.5226929117958));
#84546=CARTESIAN_POINT('Ctrl Pts',(4.29092662550047,8.33003804055367,14.3259466798393));
#84547=CARTESIAN_POINT('Ctrl Pts',(4.05084536093733,8.45370747464059,14.3303894881587));
#84548=CARTESIAN_POINT('Ctrl Pts',(3.80551611770131,8.56694707685406,14.3347937749374));
#84549=CARTESIAN_POINT('Ctrl Pts',(3.47798520775956,8.70127839277931,14.3406310429407));
#84550=CARTESIAN_POINT('Ctrl Pts',(3.39992225332927,8.73207623756258,14.342018827415));
#84551=CARTESIAN_POINT('Ctrl Pts',(3.26648413190112,8.78266034162208,14.3443885984858));
#84552=CARTESIAN_POINT('Ctrl Pts',(3.2113171583457,8.80298150385962,14.3453676102072));
#84553=CARTESIAN_POINT('Ctrl Pts',(3.06284214511523,8.85609191613734,14.3480020271751));
#84554=CARTESIAN_POINT('Ctrl Pts',(2.96920028501613,8.88792527187953,14.3496630885747));
#84555=CARTESIAN_POINT('Ctrl Pts',(2.80000432352773,8.94247067099421,14.3526667798033));
#84556=CARTESIAN_POINT('Ctrl Pts',(2.72463396102764,8.96572226082316,14.3540056420404));
#84557=CARTESIAN_POINT('Ctrl Pts',(2.55629726413946,9.01533501480509,14.3569987948649));
#84558=CARTESIAN_POINT('Ctrl Pts',(2.46319858758205,9.04121528277558,14.3586561043616));
#84559=CARTESIAN_POINT('Ctrl Pts',(2.01042058168902,9.15956922139413,14.3667257668998));
#84560=CARTESIAN_POINT('Ctrl Pts',(1.64586025526886,9.23204422622544,14.3732667824454));
#84561=CARTESIAN_POINT('Ctrl Pts',(1.08714467519491,9.30896366021473,14.3831732090329));
#84562=CARTESIAN_POINT('Ctrl Pts',(0.895558215445643,9.32934423204637,14.3865462398719));
#84563=CARTESIAN_POINT('Ctrl Pts',(0.647066226770523,9.3480527859424,14.390843468458));
#84564=CARTESIAN_POINT('Ctrl Pts',(0.590615274597854,9.35178909129636,14.391814441156));
#84565=CARTESIAN_POINT('Ctrl Pts',(0.491996767333084,9.35741981357484,14.3934996093404));
#84566=CARTESIAN_POINT('Ctrl Pts',(0.449844045780326,9.35954094634964,14.3942162129236));
#84567=CARTESIAN_POINT('Ctrl Pts',(0.346364072686315,9.36404739122861,14.3959667566645));
#84568=CARTESIAN_POINT('Ctrl Pts',(0.285025072492648,9.36611511507469,14.3969972269791));
#84569=CARTESIAN_POINT('Ctrl Pts',(-0.0965361060028026,9.3752256673999,
14.4033737098141));
#84570=CARTESIAN_POINT('Ctrl Pts',(-0.416925000390062,9.36644814392845,
14.4085882986319));
#84571=CARTESIAN_POINT('Ctrl Pts',(-0.899340459825774,9.32842647220958,
14.4165309663505));
#84572=CARTESIAN_POINT('Ctrl Pts',(-1.06208100147298,9.31130160122788,14.4192246645185));
#84573=CARTESIAN_POINT('Ctrl Pts',(-1.35010068027961,9.27334441438653,14.4240469960312));
#84574=CARTESIAN_POINT('Ctrl Pts',(-1.47556199507631,9.25421013125627,14.4261661615369));
#84575=CARTESIAN_POINT('Ctrl Pts',(-1.68129145381729,9.21854389970623,14.4296796424607));
#84576=CARTESIAN_POINT('Ctrl Pts',(-1.76180021195588,9.20349675718852,14.4310643121705));
#84577=CARTESIAN_POINT('Ctrl Pts',(-1.9148651920481,9.17280675706991,14.4337167960061));
#84578=CARTESIAN_POINT('Ctrl Pts',(-1.98745315663559,9.15735346202679,14.4349832800418));
#84579=CARTESIAN_POINT('Ctrl Pts',(-2.18706434551763,9.11237290345313,14.4384902996344));
#84580=CARTESIAN_POINT('Ctrl Pts',(-2.31366631626269,9.0810538165816,14.4407420411893));
#84581=CARTESIAN_POINT('Ctrl Pts',(-2.75620799057858,8.96172138813919,14.4487053985504));
#84582=CARTESIAN_POINT('Ctrl Pts',(-3.06814178782416,8.85977637288835,14.4544935594099));
#84583=CARTESIAN_POINT('Ctrl Pts',(-3.47976170918821,8.70090079202678,14.4622328724799));
#84584=CARTESIAN_POINT('Ctrl Pts',(-3.58468944130418,8.65819945654388,14.46421390005));
#84585=CARTESIAN_POINT('Ctrl Pts',(-3.76298356364481,8.58184416268024,14.4675817042819));
#84586=CARTESIAN_POINT('Ctrl Pts',(-3.83673670643166,8.54912545397693,14.4689752828404));
#84587=CARTESIAN_POINT('Ctrl Pts',(-3.95067431189847,8.49680852002755,14.4711240803083));
#84588=CARTESIAN_POINT('Ctrl Pts',(-3.99115657033654,8.47786835217413,14.4718867275096));
#84589=CARTESIAN_POINT('Ctrl Pts',(-4.07473980431761,8.43803145218863,14.4734585209734));
#84590=CARTESIAN_POINT('Ctrl Pts',(-4.11781914576937,8.41709241703564,14.4742671666284));
#84591=CARTESIAN_POINT('Ctrl Pts',(-4.25045517172635,8.3513617033913,14.4767550251326));
#84592=CARTESIAN_POINT('Ctrl Pts',(-4.3394559970726,8.30546405714749,14.4784218257828));
#84593=CARTESIAN_POINT('Ctrl Pts',(-4.76830583917766,8.07553113557125,14.486476355208));
#84594=CARTESIAN_POINT('Ctrl Pts',(-5.09728372106305,7.87201651796003,14.4927425875687));
#84595=CARTESIAN_POINT('Ctrl Pts',(-5.46846809484981,7.60934296379044,14.5002696190677));
#84596=CARTESIAN_POINT('Ctrl Pts',(-5.52374997446446,7.56930841279338,14.5014027449445));
#84597=CARTESIAN_POINT('Ctrl Pts',(-5.66625192062478,7.46371745369295,14.504357765077));
#84598=CARTESIAN_POINT('Ctrl Pts',(-5.75277301358116,7.39723540453827,14.5061858278198));
#84599=CARTESIAN_POINT('Ctrl Pts',(-5.90035128572482,7.27968207350246,14.5093679508152));
#84600=CARTESIAN_POINT('Ctrl Pts',(-5.96195525657858,7.22931572629689,14.510716202894));
#84601=CARTESIAN_POINT('Ctrl Pts',(-6.09176068910101,7.12040128765922,14.5136011405656));
#84602=CARTESIAN_POINT('Ctrl Pts',(-6.15977636972704,7.06164412982918,14.515139474987));
#84603=CARTESIAN_POINT('Ctrl Pts',(-6.3656906445377,6.87852072121091,14.5198799773297));
#84604=CARTESIAN_POINT('Ctrl Pts',(-6.50074610111098,6.75102691832861,14.5231073643514));
#84605=CARTESIAN_POINT('Ctrl Pts',(-6.82837374691557,6.42278958076299,14.531220486772));
#84606=CARTESIAN_POINT('Ctrl Pts',(-7.01596464021389,6.2173269044752,14.5361308942662));
#84607=CARTESIAN_POINT('Ctrl Pts',(-7.25364136442272,5.93252862694117,14.5426215921704));
#84608=CARTESIAN_POINT('Ctrl Pts',(-7.31207985259046,5.86034958288285,14.5442407057133));
#84609=CARTESIAN_POINT('Ctrl Pts',(-7.41300339468307,5.7318358025775,14.5470711140271));
#84610=CARTESIAN_POINT('Ctrl Pts',(-7.45594317718138,5.67586754348695,14.5482867726703));
#84611=CARTESIAN_POINT('Ctrl Pts',(-7.52411042032971,5.58490889441025,14.5502319188713));
#84612=CARTESIAN_POINT('Ctrl Pts',(-7.54973536840059,5.55021989351209,14.5509666680425));
#84613=CARTESIAN_POINT('Ctrl Pts',(-7.60525486849176,5.47396607638004,14.5525656420107));
#84614=CARTESIAN_POINT('Ctrl Pts',(-7.63505003540046,5.43233073298915,14.553428565614));
#84615=CARTESIAN_POINT('Ctrl Pts',(-7.72707723534672,5.30148038065266,14.5561123583616));
#84616=CARTESIAN_POINT('Ctrl Pts',(-7.78809810351027,5.21142445617067,14.5579190439355));
#84617=CARTESIAN_POINT('Ctrl Pts',(-7.9184003742091,5.01172001446904,14.5618583395755));
#84618=CARTESIAN_POINT('Ctrl Pts',(-7.98700127024777,4.90165408575369,14.5639864987368));
#84619=CARTESIAN_POINT('Ctrl Pts',(-8.06904069476718,4.76372920379202,14.5666175706578));
#84620=CARTESIAN_POINT('Ctrl Pts',(-8.08465512460191,4.73718114254341,14.567122384326));
#84621=CARTESIAN_POINT('Ctrl Pts',(-8.23598463194248,4.47695924952901,14.5720562953741));
#84622=CARTESIAN_POINT('Ctrl Pts',(-8.36166217790112,4.23759509557695,14.5764872566878));
#84623=CARTESIAN_POINT('Ctrl Pts',(-8.52439840272248,3.89213086903517,14.5828459701593));
#84624=CARTESIAN_POINT('Ctrl Pts',(-8.57016901720414,3.79028412666944,14.5847156788946));
#84625=CARTESIAN_POINT('Ctrl Pts',(-8.6455334452908,3.61423747804889,14.5879442155574));
#84626=CARTESIAN_POINT('Ctrl Pts',(-8.67601865115214,3.54043237918989,14.589296713674));
#84627=CARTESIAN_POINT('Ctrl Pts',(-8.73838622968068,3.38379480239614,14.5921661954579));
#84628=CARTESIAN_POINT('Ctrl Pts',(-8.77004261627735,3.30088073475064,14.5936845794317));
#84629=CARTESIAN_POINT('Ctrl Pts',(-8.86096118134483,3.05220227377164,14.5982374753096));
#84630=CARTESIAN_POINT('Ctrl Pts',(-8.91673504347879,2.88520495304862,14.6012941059062));
#84631=CARTESIAN_POINT('Ctrl Pts',(-8.98426472226402,2.66229383709832,14.6053650068161));
#84632=CARTESIAN_POINT('Ctrl Pts',(-9.00026166360764,2.60770225575625,14.6063611900446));
#84633=CARTESIAN_POINT('Ctrl Pts',(-9.0823796197847,2.31770422175702,14.6116466204395));
#84634=CARTESIAN_POINT('Ctrl Pts',(-9.13976442393024,2.07992274142518,14.6159607080618));
#84635=CARTESIAN_POINT('Ctrl Pts',(-9.20508217569917,1.75379776084045,14.6217760392419));
#84636=CARTESIAN_POINT('Ctrl Pts',(-9.22116237515398,1.6671859356969,14.6233105317947));
#84637=CARTESIAN_POINT('Ctrl Pts',(-9.24748800528196,1.51333238846675,14.6260123354634));
#84638=CARTESIAN_POINT('Ctrl Pts',(-9.25822705038691,1.44618160734907,14.6271834980128));
#84639=CARTESIAN_POINT('Ctrl Pts',(-9.27453246328535,1.33658684568228,14.6290787286666));
#84640=CARTESIAN_POINT('Ctrl Pts',(-9.28054062028352,1.29421119818023,14.6298075358139));
#84641=CARTESIAN_POINT('Ctrl Pts',(-9.29325418805039,1.19989750487372,14.6314200992881));
#84642=CARTESIAN_POINT('Ctrl Pts',(-9.29981492965487,1.14794151269805,14.6323022893931));
#84643=CARTESIAN_POINT('Ctrl Pts',(-9.32081629198952,0.969611833663032,
14.6353130541187));
#84644=CARTESIAN_POINT('Ctrl Pts',(-9.33311920349649,0.843000325885971,
14.6374212494292));
#84645=CARTESIAN_POINT('Ctrl Pts',(-9.36110118395367,0.477963431696432,
14.6434571253253));
#84646=CARTESIAN_POINT('Ctrl Pts',(-9.37024427109779,0.2391380051819,14.6473561618306));
#84647=CARTESIAN_POINT('Ctrl Pts',(-9.37025135436427,-0.05639555157854,
14.6522120430209));
#84648=CARTESIAN_POINT('Ctrl Pts',(-9.36973951704211,-0.113014508858485,
14.6531436177697));
#84649=CARTESIAN_POINT('Ctrl Pts',(-9.36581304919372,-0.329880466951533,
14.6567195284928));
#84650=CARTESIAN_POINT('Ctrl Pts',(-9.35880020392255,-0.490034425258301,
14.6593769645584));
#84651=CARTESIAN_POINT('Ctrl Pts',(-9.34118377445768,-0.743404788223204,
14.6636271706575));
#84652=CARTESIAN_POINT('Ctrl Pts',(-9.33328283111655,-0.836777466382237,
14.6652032868241));
#84653=CARTESIAN_POINT('Ctrl Pts',(-9.31614035832275,-1.00864134985332,
14.6681250429189));
#84654=CARTESIAN_POINT('Ctrl Pts',(-9.30730368775735,-1.08716446716224,
14.6694679598235));
#84655=CARTESIAN_POINT('Ctrl Pts',(-9.28472180551968,-1.26729534730405,
14.672567911156));
#84656=CARTESIAN_POINT('Ctrl Pts',(-9.27029994115426,-1.36880803354643,
14.674329105132));
#84657=CARTESIAN_POINT('Ctrl Pts',(-9.24447254778108,-1.53139439240809,
14.6771725761396));
#84658=CARTESIAN_POINT('Ctrl Pts',(-9.23412046928646,-1.59262695455721,
14.6782486446894));
#84659=CARTESIAN_POINT('Ctrl Pts',(-9.19254818345805,-1.82448025464363,
14.6823418897166));
#84660=CARTESIAN_POINT('Ctrl Pts',(-9.15720136853533,-1.99432524401874,
14.6853797638788));
#84661=CARTESIAN_POINT('Ctrl Pts',(-9.08915235353315,-2.28114346069903,
14.6905579095618));
#84662=CARTESIAN_POINT('Ctrl Pts',(-9.05885351970946,-2.39864105233331,
14.6926929153118));
#84663=CARTESIAN_POINT('Ctrl Pts',(-8.97895674897119,-2.68532992761396,
14.6979202285522));
#84664=CARTESIAN_POINT('Ctrl Pts',(-8.92684915818135,-2.85377390227389,
14.7010074689203));
#84665=CARTESIAN_POINT('Ctrl Pts',(-8.84961105654361,-3.08058074754514,
14.7051489325922));
#84666=CARTESIAN_POINT('Ctrl Pts',(-8.82859417818543,-3.14030547207364,
14.7062379365153));
#84667=CARTESIAN_POINT('Ctrl Pts',(-8.79251940762764,-3.23959551889592,
14.7080431842528));
#84668=CARTESIAN_POINT('Ctrl Pts',(-8.77779583854697,-3.27927993516069,
14.7087632130622));
#84669=CARTESIAN_POINT('Ctrl Pts',(-8.74327932431064,-3.37041397817867,
14.7104129896911));
#84670=CARTESIAN_POINT('Ctrl Pts',(-8.72330028836909,-3.42179131814794,
14.7113405703043));
#84671=CARTESIAN_POINT('Ctrl Pts',(-8.6410924679992,-3.6277936418695,14.715054989824));
#84672=CARTESIAN_POINT('Ctrl Pts',(-8.5751962791023,-3.78092248589737,14.7178055821021));
#84673=CARTESIAN_POINT('Ctrl Pts',(-8.36739408396648,-4.23039204866728,
14.7259425156153));
#84674=CARTESIAN_POINT('Ctrl Pts',(-8.21395248892635,-4.52111548752836,
14.7312964588699));
#84675=CARTESIAN_POINT('Ctrl Pts',(-7.97975984102508,-4.91339966486704,
14.7388783260067));
#84676=CARTESIAN_POINT('Ctrl Pts',(-7.91170073927985,-5.02225593489993,
14.7410215039779));
#84677=CARTESIAN_POINT('Ctrl Pts',(-7.80094838019064,-5.19155628873473,
14.7444252512929));
#84678=CARTESIAN_POINT('Ctrl Pts',(-7.75973896565726,-5.25295188319357,
14.7456745934583));
#84679=CARTESIAN_POINT('Ctrl Pts',(-7.67119566417211,-5.38155162198325,
14.7483245262173));
#84680=CARTESIAN_POINT('Ctrl Pts',(-7.62369540382396,-5.44863369385304,
14.7497263275338));
#84681=CARTESIAN_POINT('Ctrl Pts',(-7.49944580980689,-5.61929847813231,
14.753343977036));
#84682=CARTESIAN_POINT('Ctrl Pts',(-7.42143044993666,-5.72193785193335,
14.7555694055062));
#84683=CARTESIAN_POINT('Ctrl Pts',(-7.28638913881069,-5.89219252091804,
14.7593439547139));
#84684=CARTESIAN_POINT('Ctrl Pts',(-7.23047849674247,-5.96066943053437,
14.7608855831825));
#84685=CARTESIAN_POINT('Ctrl Pts',(-6.95176818780392,-6.2923290105902,14.768463030344));
#84686=CARTESIAN_POINT('Ctrl Pts',(-6.71552700823923,-6.54386595828249,
14.7745684557952));
#84687=CARTESIAN_POINT('Ctrl Pts',(-6.4027891990157,-6.84203872762999,14.7820815678534));
#84688=CARTESIAN_POINT('Ctrl Pts',(-6.33877828813087,-6.90138343751596,
14.7835911190928));
#84689=CARTESIAN_POINT('Ctrl Pts',(-6.23992586951538,-6.99049413546934,
14.7858739778964));
#84690=CARTESIAN_POINT('Ctrl Pts',(-6.20567974074907,-7.02091319451156,
14.786656213681));
#84691=CARTESIAN_POINT('Ctrl Pts',(-6.13623055794022,-7.08169617023907,
14.7882240397799));
#84692=CARTESIAN_POINT('Ctrl Pts',(-6.10102181769235,-7.11205166601367,
14.7890095096051));
#84693=CARTESIAN_POINT('Ctrl Pts',(-5.99597819946792,-7.20126176582358,
14.7913276799931));
#84694=CARTESIAN_POINT('Ctrl Pts',(-5.92550707995577,-7.25935889061715,
14.7928502637643));
#84695=CARTESIAN_POINT('Ctrl Pts',(-5.74690385742039,-7.40226745508306,
14.7966425463728));
#84696=CARTESIAN_POINT('Ctrl Pts',(-5.63773418436791,-7.48574784570016,
14.7989012243898));
#84697=CARTESIAN_POINT('Ctrl Pts',(-5.23094710274699,-7.78286402140929,
14.8071649672548));
#84698=CARTESIAN_POINT('Ctrl Pts',(-4.92271110412059,-7.98139680474615,
14.8131484634814));
#84699=CARTESIAN_POINT('Ctrl Pts',(-4.52056863147075,-8.20823624073675,
14.8208704554806));
#84700=CARTESIAN_POINT('Ctrl Pts',(-4.4367808478872,-8.25382690557972,14.8224740389974));
#84701=CARTESIAN_POINT('Ctrl Pts',(-4.28309913330269,-8.33443189851926,
14.8254084763126));
#84702=CARTESIAN_POINT('Ctrl Pts',(-4.21343511912902,-8.36986605155365,
14.8267361464593));
#84703=CARTESIAN_POINT('Ctrl Pts',(-4.05375281063335,-8.4485885708916,14.8297746572075));
#84704=CARTESIAN_POINT('Ctrl Pts',(-3.9634693143098,-8.49131742534833,14.8314892666445));
#84705=CARTESIAN_POINT('Ctrl Pts',(-3.62763479183893,-8.6437360045026,14.8378547593405));
#84706=CARTESIAN_POINT('Ctrl Pts',(-3.37807916548652,-8.74428307273401,
14.8425643928425));
#84707=CARTESIAN_POINT('Ctrl Pts',(-2.86323900478452,-8.92638063170287,
14.8521629574976));
#84708=CARTESIAN_POINT('Ctrl Pts',(-2.59795908274709,-9.00716480402229,
14.857048185045));
#84709=CARTESIAN_POINT('Ctrl Pts',(-2.27651965451766,-9.0896663267212,14.8627790601197));
#84710=CARTESIAN_POINT('Ctrl Pts',(-2.2234320178086,-9.10279768797023,14.8637193224976));
#84711=CARTESIAN_POINT('Ctrl Pts',(-2.12881805343246,-9.12532361765254,
14.8653822659638));
#84712=CARTESIAN_POINT('Ctrl Pts',(-2.08733696132503,-9.13490130550559,
14.8661069032441));
#84713=CARTESIAN_POINT('Ctrl Pts',(-1.99364354946407,-9.15586293153534,
14.8677331491781));
#84714=CARTESIAN_POINT('Ctrl Pts',(-1.94139632872598,-9.16708355670175,
14.8686329550725));
#84715=CARTESIAN_POINT('Ctrl Pts',(-1.74642443891925,-9.20721414667796,
14.8719689919735));
#84716=CARTESIAN_POINT('Ctrl Pts',(-1.60312755750746,-9.23324281741756,
14.8743777718265));
#84717=CARTESIAN_POINT('Ctrl Pts',(-1.10868226379325,-9.31119671788151,
14.8826162851932));
#84718=CARTESIAN_POINT('Ctrl Pts',(-0.755225319006357,-9.34650714695677,
14.8883906199345));
#84719=CARTESIAN_POINT('Ctrl Pts',(-0.272997798198905,-9.36714333229914,
14.8964014782491));
#84720=CARTESIAN_POINT('Ctrl Pts',(-0.145278763930164,-9.36999444847109,
14.8985343542295));
#84721=CARTESIAN_POINT('Ctrl Pts',(0.0563156259553912,-9.3703718460242,
14.9019263187443));
#84722=CARTESIAN_POINT('Ctrl Pts',(0.130171878215257,-9.36963687863521,
14.903174328213));
#84723=CARTESIAN_POINT('Ctrl Pts',(0.286281796148723,-9.36623720540823,
14.9058246348694));
#84724=CARTESIAN_POINT('Ctrl Pts',(0.368524675021764,-9.36336190588312,
14.9072281715753));
#84725=CARTESIAN_POINT('Ctrl Pts',(0.580136466425123,-9.35317136042498,
14.9108589869445));
#84726=CARTESIAN_POINT('Ctrl Pts',(0.709410561265598,-9.34425541896425,
14.9130959933781));
#84727=CARTESIAN_POINT('Ctrl Pts',(1.00699831646342,-9.31751976764447,14.9182863726715));
#84728=CARTESIAN_POINT('Ctrl Pts',(1.17509734816618,-9.29781513267433,14.9212487925555));
#84729=CARTESIAN_POINT('Ctrl Pts',(1.64518656150708,-9.22975852311878,14.9295905060204));
#84730=CARTESIAN_POINT('Ctrl Pts',(1.9454773503055,-9.17116128743463,14.9349906750936));
#84731=CARTESIAN_POINT('Ctrl Pts',(2.30373964137129,-9.08286102712808,14.9413683756027));
#84732=CARTESIAN_POINT('Ctrl Pts',(2.36496006767125,-9.06711335973801,14.942455604498));
#84733=CARTESIAN_POINT('Ctrl Pts',(2.46689317939797,-9.03979059796486,14.9442589502369));
#84734=CARTESIAN_POINT('Ctrl Pts',(2.50769509508009,-9.02855699103623,14.9449788315351));
#84735=CARTESIAN_POINT('Ctrl Pts',(2.60153369943944,-9.00203609771469,14.9466296350848));
#84736=CARTESIAN_POINT('Ctrl Pts',(2.65451409950806,-8.98655587020102,14.9475583751003));
#84737=CARTESIAN_POINT('Ctrl Pts',(2.86791102105804,-8.92215208268953,14.9512911744615));
#84738=CARTESIAN_POINT('Ctrl Pts',(3.02713800522539,-8.86939384821649,14.954058524797));
#84739=CARTESIAN_POINT('Ctrl Pts',(3.49397727825909,-8.70067466763205,14.9622148063664));
#84740=CARTESIAN_POINT('Ctrl Pts',(3.7969985637573,-8.57277194888512,14.9675719519537));
#84741=CARTESIAN_POINT('Ctrl Pts',(4.20749628118755,-8.37346123146881,14.975145721397));
#84742=CARTESIAN_POINT('Ctrl Pts',(4.32116943254741,-8.31536965892312,14.9772770574238));
#84743=CARTESIAN_POINT('Ctrl Pts',(4.4986757871922,-8.22003371662507,14.9806672610655));
#84744=CARTESIAN_POINT('Ctrl Pts',(4.56331609471864,-8.18432552708443,14.9819150716935));
#84745=CARTESIAN_POINT('Ctrl Pts',(4.69909484115661,-8.10721078688609,14.9845654388003));
#84746=CARTESIAN_POINT('Ctrl Pts',(4.77012345888892,-8.06562342401307,14.985969239139));
#84747=CARTESIAN_POINT('Ctrl Pts',(4.95162020213482,-7.9561206670151,14.9896020532128));
#84748=CARTESIAN_POINT('Ctrl Pts',(5.06124288631309,-7.88683834003664,14.9918408171678));
#84749=CARTESIAN_POINT('Ctrl Pts',(5.31070775317086,-7.72183109226504,14.9970367141201));
#84750=CARTESIAN_POINT('Ctrl Pts',(5.449461815304,-7.62454313184033,15.0000029260064));
#84751=CARTESIAN_POINT('Ctrl Pts',(5.838435773624,-7.33576782638403,15.0085108856225));
#84752=CARTESIAN_POINT('Ctrl Pts',(6.0817399418717,-7.13535293226558,15.014075560044));
#84753=CARTESIAN_POINT('Ctrl Pts',(6.35368277420726,-6.8873154888373,15.0204277575143));
#84754=CARTESIAN_POINT('Ctrl Pts',(6.39257420994285,-6.85123305869351,15.0213393608049));
#84755=CARTESIAN_POINT('Ctrl Pts',(6.46196353379338,-6.78575025795265,15.0229699066767));
#84756=CARTESIAN_POINT('Ctrl Pts',(6.4925723971653,-6.75646971134094,15.0236905291332));
#84757=CARTESIAN_POINT('Ctrl Pts',(6.56236296419189,-6.68879559419791,15.0253364167723));
#84758=CARTESIAN_POINT('Ctrl Pts',(6.60140808083821,-6.65026356948071,15.0262595722346));
#84759=CARTESIAN_POINT('Ctrl Pts',(6.75503020580465,-6.49597406578625,15.0299062021755));
#84760=CARTESIAN_POINT('Ctrl Pts',(6.86691937385006,-6.37758032174672,15.0325951067752));
#84761=CARTESIAN_POINT('Ctrl Pts',(7.19447386980348,-6.01236451097467,15.0406585865365));
#84762=CARTESIAN_POINT('Ctrl Pts',(7.40033223573199,-5.75708817217689,15.0459985038913));
#84763=CARTESIAN_POINT('Ctrl Pts',(7.66926069909016,-5.38527884090373,15.0536098250143));
#84764=CARTESIAN_POINT('Ctrl Pts',(7.74388835269695,-5.2774028570135,15.0557986345105));
#84765=CARTESIAN_POINT('Ctrl Pts',(7.85721281820569,-5.10600765984033,15.0592546247565));
#84766=CARTESIAN_POINT('Ctrl Pts',(7.89745994506394,-5.04353386837535,15.0605099136011));
#84767=CARTESIAN_POINT('Ctrl Pts',(7.98043747169921,-4.91130263900006,15.0631587853762));
#84768=CARTESIAN_POINT('Ctrl Pts',(8.02300615893516,-4.84145102089897,15.0645534564323));
#84769=CARTESIAN_POINT('Ctrl Pts',(8.12890958111824,-4.66243920237817,15.0681167863805));
#84770=CARTESIAN_POINT('Ctrl Pts',(8.1909635842154,-4.55254057947949,15.0702944241105));
#84771=CARTESIAN_POINT('Ctrl Pts',(8.29128752695059,-4.36616995769018,15.0739690672849));
#84772=CARTESIAN_POINT('Ctrl Pts',(8.33076473325884,-4.29036687031483,15.0754586663927));
#84773=CARTESIAN_POINT('Ctrl Pts',(8.51144201287931,-3.93153634955085,15.0824819419));
#84774=CARTESIAN_POINT('Ctrl Pts',(8.63928969651244,-3.64201814470987,15.0880748743119));
#84775=CARTESIAN_POINT('Ctrl Pts',(8.79080935000653,-3.24575277713097,15.0954807079435));
#84776=CARTESIAN_POINT('Ctrl Pts',(8.82762133949223,-3.14425534954562,15.0973555561701));
#84777=CARTESIAN_POINT('Ctrl Pts',(8.87924706107478,-2.99385426826711,15.1000911703786));
#84778=CARTESIAN_POINT('Ctrl Pts',(8.89542788383968,-2.94542943050717,15.1009655164933));
#84779=CARTESIAN_POINT('Ctrl Pts',(8.92455936139365,-2.85581672614698,15.102570148329));
#84780=CARTESIAN_POINT('Ctrl Pts',(8.93762263297203,-2.81466705601372,15.1033016505745));
#84781=CARTESIAN_POINT('Ctrl Pts',(8.97137908065879,-2.70572833975215,15.105225441598));
#84782=CARTESIAN_POINT('Ctrl Pts',(8.99158834455321,-2.63779217062365,15.1064122900545));
#84783=CARTESIAN_POINT('Ctrl Pts',(9.03666732100547,-2.47971210454445,15.1091505006019));
#84784=CARTESIAN_POINT('Ctrl Pts',(9.06096232529297,-2.38941210034794,15.1106971262895));
#84785=CARTESIAN_POINT('Ctrl Pts',(9.15333455809474,-2.02438965171595,15.1169016304677));
#84786=CARTESIAN_POINT('Ctrl Pts',(9.21030078596373,-1.74701081497711,15.1215132882247));
#84787=CARTESIAN_POINT('Ctrl Pts',(9.2830167155094,-1.28842956847979,15.1291646404631));
#84788=CARTESIAN_POINT('Ctrl Pts',(9.30620598902747,-1.10859365665703,15.1321707160256));
#84789=CARTESIAN_POINT('Ctrl Pts',(9.33301699705726,-0.839265364406819,
15.1367073458948));
#84790=CARTESIAN_POINT('Ctrl Pts',(9.3405972919208,-0.750209838905443,15.138212871676));
#84791=CARTESIAN_POINT('Ctrl Pts',(9.35252421224344,-0.581571865928536,
15.14107622203));
#84792=CARTESIAN_POINT('Ctrl Pts',(9.35713178070997,-0.502015716461471,
15.1424322438239));
#84793=CARTESIAN_POINT('Ctrl Pts',(9.36569166262584,-0.31232660322585,15.1456787454651));
#84794=CARTESIAN_POINT('Ctrl Pts',(9.36871698526925,-0.202163767082633,
15.1475748789663));
#84795=CARTESIAN_POINT('Ctrl Pts',(9.37108834110714,0.0394182011394155,
15.1517556994895));
#84796=CARTESIAN_POINT('Ctrl Pts',(9.36961419443536,0.17082218711811,15.1540445620345));
#84797=CARTESIAN_POINT('Ctrl Pts',(9.35368840482981,0.664452319270811,15.1626855823257));
#84798=CARTESIAN_POINT('Ctrl Pts',(9.32098606602358,1.02576885517853,15.1691088980123));
#84799=CARTESIAN_POINT('Ctrl Pts',(9.25646844379374,1.45769945460381,15.1766807073362));
#84800=CARTESIAN_POINT('Ctrl Pts',(9.24462963869411,1.53098616402235,15.1779611413842));
#84801=CARTESIAN_POINT('Ctrl Pts',(9.22517811390165,1.64293192510444,15.179906716406));
#84802=CARTESIAN_POINT('Ctrl Pts',(9.21819036109052,1.68169647223961,15.1805785220759));
#84803=CARTESIAN_POINT('Ctrl Pts',(9.20221454731507,1.76722960168414,15.1820558052592));
#84804=CARTESIAN_POINT('Ctrl Pts',(9.1931139443524,1.81397603595547,15.1828599392524));
#84805=CARTESIAN_POINT('Ctrl Pts',(9.16412567605563,1.95705408039645,15.1853138312532));
#84806=CARTESIAN_POINT('Ctrl Pts',(9.14307721210707,2.05314374972946,15.1869516544349));
#84807=CARTESIAN_POINT('Ctrl Pts',(9.08491392674533,2.30000645015942,15.1911510365151));
#84808=CARTESIAN_POINT('Ctrl Pts',(9.04555749451854,2.4502204985434,15.1936985187694));
#84809=CARTESIAN_POINT('Ctrl Pts',(8.91263752020387,2.91056371866555,15.2015535554786));
#84810=CARTESIAN_POINT('Ctrl Pts',(8.8067145978278,3.21687211462933,15.2068555368832));
#84811=CARTESIAN_POINT('Ctrl Pts',(8.64749778597169,3.61004532016563,15.213939327009));
#84812=CARTESIAN_POINT('Ctrl Pts',(8.60836043250434,3.70240135207181,15.2156233076951));
#84813=CARTESIAN_POINT('Ctrl Pts',(8.53579668638417,3.86626262981798,15.2186504463519));
#84814=CARTESIAN_POINT('Ctrl Pts',(8.50293526566627,3.93800757088068,15.219989558651));
#84815=CARTESIAN_POINT('Ctrl Pts',(8.42834993689971,4.09555911756303,15.2229617375705));
#84816=CARTESIAN_POINT('Ctrl Pts',(8.38621375928479,4.18116082799509,15.2245975843047));
#84817=CARTESIAN_POINT('Ctrl Pts',(8.22535744100787,4.49573087222814,15.2306874684807));
#84818=CARTESIAN_POINT('Ctrl Pts',(8.09850717779906,4.72041117744608,15.2351963973872));
#84819=CARTESIAN_POINT('Ctrl Pts',(7.80041307499569,5.20093660647382,15.2451304074111));
#84820=CARTESIAN_POINT('Ctrl Pts',(7.62550443927557,5.45416062726863,15.2505603927787));
#84821=CARTESIAN_POINT('Ctrl Pts',(7.40687826366323,5.73955020121121,15.2567619833702));
#84822=CARTESIAN_POINT('Ctrl Pts',(7.37495389243577,5.78051357793326,15.2576540100204));
#84823=CARTESIAN_POINT('Ctrl Pts',(7.31644424456274,5.85431580783031,15.2592630236567));
#84824=CARTESIAN_POINT('Ctrl Pts',(7.28997432245437,5.88724420715825,15.2599814985525));
#84825=CARTESIAN_POINT('Ctrl Pts',(7.22792538535899,5.96337250412848,15.2616437270448));
#84826=CARTESIAN_POINT('Ctrl Pts',(7.19218032034089,6.0064348209689,15.2625851349745));
#84827=CARTESIAN_POINT('Ctrl Pts',(7.03967501287623,6.18684553104261,15.2665398802811));
#84828=CARTESIAN_POINT('Ctrl Pts',(6.91934942525058,6.32113010747913,15.2695106592199));
#84829=CARTESIAN_POINT('Ctrl Pts',(6.52518241178908,6.73627449098843,15.2789100080205));
#84830=CARTESIAN_POINT('Ctrl Pts',(6.2375507427531,7.00345344388833,15.2853040262032));
#84831=CARTESIAN_POINT('Ctrl Pts',(5.86107149062879,7.31151913900467,15.2934429722194));
#84832=CARTESIAN_POINT('Ctrl Pts',(5.78722061869043,7.37011184409929,15.2950283112351));
#84833=CARTESIAN_POINT('Ctrl Pts',(5.64989843130722,7.47572534876947,15.2979584827));
#84834=CARTESIAN_POINT('Ctrl Pts',(5.58669241970508,7.52307713294167,15.2993004766885));
#84835=CARTESIAN_POINT('Ctrl Pts',(5.44069856637601,7.62959613208488,15.3023860041862));
#84836=CARTESIAN_POINT('Ctrl Pts',(5.3575304237325,7.68822513442907,15.3041335477523));
#84837=CARTESIAN_POINT('Ctrl Pts',(5.07333675975128,7.88171503962326,15.3100707132721));
#84838=CARTESIAN_POINT('Ctrl Pts',(4.86804651796867,8.01013734082422,15.3143049608386));
#84839=CARTESIAN_POINT('Ctrl Pts',(4.53713320989625,8.19972048212067,15.3210050454066));
#84840=CARTESIAN_POINT('Ctrl Pts',(4.4147394240174,8.26626022482994,15.3234567955017));
#84841=CARTESIAN_POINT('Ctrl Pts',(4.29092660882816,8.33003804914182,15.3259008099036));
#84842=CARTESIAN_POINT('Origin',(0.,0.,2.15141010809499));
#84843=CARTESIAN_POINT('',(4.29092663733565,8.33003803445719,16.522914704178));
#84844=CARTESIAN_POINT('',(4.29092662815671,8.3300380391854,16.3257048922231));
#84845=CARTESIAN_POINT('',(4.29092662815669,8.33003803918541,2.15141010809499));
#84846=CARTESIAN_POINT('Ctrl Pts',(4.29092663733565,8.33003803445719,16.522914704178));
#84847=CARTESIAN_POINT('Ctrl Pts',(4.34419074622071,8.30260089879425,16.5218617865547));
#84848=CARTESIAN_POINT('Ctrl Pts',(4.3971956545877,8.27465085053372,16.5208081053267));
#84849=CARTESIAN_POINT('Ctrl Pts',(4.59003078621386,8.17059025536445,16.5169558422932));
#84850=CARTESIAN_POINT('Ctrl Pts',(4.72817847057187,8.09143103549738,16.5141589721163));
#84851=CARTESIAN_POINT('Ctrl Pts',(4.92552548441208,7.97156978210543,16.5101354584452));
#84852=CARTESIAN_POINT('Ctrl Pts',(4.98637943026975,7.93364646900825,16.5088908545452));
#84853=CARTESIAN_POINT('Ctrl Pts',(5.09633041068881,7.86336176326533,16.5066386623559));
#84854=CARTESIAN_POINT('Ctrl Pts',(5.14556957709859,7.83122950910619,16.505628791034));
#84855=CARTESIAN_POINT('Ctrl Pts',(5.22614112555678,7.77756253902676,16.5039762412962));
#84856=CARTESIAN_POINT('Ctrl Pts',(5.25765053963257,7.75629685644575,16.5033300466127));
#84857=CARTESIAN_POINT('Ctrl Pts',(5.33419320423295,7.70395751391395,16.5017605373996));
#84858=CARTESIAN_POINT('Ctrl Pts',(5.37908530880289,7.67268009076504,16.5008399863193));
#84859=CARTESIAN_POINT('Ctrl Pts',(5.5585497033799,7.54529365225603,16.4971546337167));
#84860=CARTESIAN_POINT('Ctrl Pts',(5.6908414002494,7.44602280243445,16.4944254486344));
#84861=CARTESIAN_POINT('Ctrl Pts',(6.02926471379512,7.17778226458798,16.4873290361088));
#84862=CARTESIAN_POINT('Ctrl Pts',(6.23093677260032,7.00342903492275,16.4829811501577));
#84863=CARTESIAN_POINT('Ctrl Pts',(6.5110773636398,6.73954535803286,16.4766287048069));
#84864=CARTESIAN_POINT('Ctrl Pts',(6.59570502211195,6.65674659631357,16.4746658724048));
#84865=CARTESIAN_POINT('Ctrl Pts',(6.75084345273616,6.49909723971123,16.4709747903405));
#84866=CARTESIAN_POINT('Ctrl Pts',(6.8217352395538,6.42464633324573,16.4692499634749));
#84867=CARTESIAN_POINT('Ctrl Pts',(6.9449375509302,6.2909199257943,16.4661800470896));
#84868=CARTESIAN_POINT('Ctrl Pts',(6.99774996248071,6.23212054825388,16.4648394988121));
#84869=CARTESIAN_POINT('Ctrl Pts',(7.11141179672457,6.10230705578462,16.4618989025599));
#84870=CARTESIAN_POINT('Ctrl Pts',(7.17195477191904,6.03103588450162,16.4602964511755));
#84871=CARTESIAN_POINT('Ctrl Pts',(7.48995401030316,5.64512613113075,16.451682696129));
#84872=CARTESIAN_POINT('Ctrl Pts',(7.72779409538944,5.31488992298295,16.4445098461343));
#84873=CARTESIAN_POINT('Ctrl Pts',(8.03349204271351,4.82632549789793,16.434397206636));
#84874=CARTESIAN_POINT('Ctrl Pts',(8.11962294895016,4.67997175777033,16.4314300300769));
#84875=CARTESIAN_POINT('Ctrl Pts',(8.22848817208142,4.48292640430834,16.4275498898206));
#84876=CARTESIAN_POINT('Ctrl Pts',(8.25481691869994,4.43425804416627,16.4266006426443));
#84877=CARTESIAN_POINT('Ctrl Pts',(8.30051226322842,4.34797320098906,16.4249355519017));
#84878=CARTESIAN_POINT('Ctrl Pts',(8.32005794672287,4.31045363676942,16.4242175600519));
#84879=CARTESIAN_POINT('Ctrl Pts',(8.3633132423917,4.22603106398965,16.4226149843629));
#84880=CARTESIAN_POINT('Ctrl Pts',(8.38688364109877,4.17905847656221,16.4217320512057));
#84881=CARTESIAN_POINT('Ctrl Pts',(8.54377464018161,3.85972220707158,16.4157808671813));
#84882=CARTESIAN_POINT('Ctrl Pts',(8.66420144452708,3.58122262967216,16.4108360116664));
#84883=CARTESIAN_POINT('Ctrl Pts',(8.86254100790409,3.0536455925217,16.4015919269044));
#84884=CARTESIAN_POINT('Ctrl Pts',(8.94397019457801,2.80620404010665,16.3973051509225));
#84885=CARTESIAN_POINT('Ctrl Pts',(9.04103727051634,2.46380836098728,16.3913532155405));
#84886=CARTESIAN_POINT('Ctrl Pts',(9.0656798728991,2.37153008674136,16.3897476093256));
#84887=CARTESIAN_POINT('Ctrl Pts',(9.10809759128846,2.20235540923167,16.3867984793622));
#84888=CARTESIAN_POINT('Ctrl Pts',(9.12632017262488,2.12558019234843,16.3854580454985));
#84889=CARTESIAN_POINT('Ctrl Pts',(9.16547215295705,1.95083076080501,16.3824014523416));
#84890=CARTESIAN_POINT('Ctrl Pts',(9.18580437482541,1.85273267483054,16.3806815859644));
#84891=CARTESIAN_POINT('Ctrl Pts',(9.2655241613127,1.43446101329832,16.3733317109346));
#84892=CARTESIAN_POINT('Ctrl Pts',(9.30977347201924,1.11163507932695,16.3676091066765));
#84893=CARTESIAN_POINT('Ctrl Pts',(9.35537412618965,0.570732537952196,16.358066770792));
#84894=CARTESIAN_POINT('Ctrl Pts',(9.3660896407541,0.35373137883533,16.3542532180947));
#84895=CARTESIAN_POINT('Ctrl Pts',(9.37015353226316,0.0748995286265283,
16.3494356565903));
#84896=CARTESIAN_POINT('Ctrl Pts',(9.37044353016443,0.0132374696732548,
16.3483755858442));
#84897=CARTESIAN_POINT('Ctrl Pts',(9.36990669744964,-0.0906426147310336,
16.3466010558192));
#84898=CARTESIAN_POINT('Ctrl Pts',(9.36940317148674,-0.13286017860814,16.3458831464376));
#84899=CARTESIAN_POINT('Ctrl Pts',(9.36758052959633,-0.230394450235545,
16.344232283201));
#84900=CARTESIAN_POINT('Ctrl Pts',(9.36605674187886,-0.285705631614874,
16.3433015471269));
#84901=CARTESIAN_POINT('Ctrl Pts',(9.35759441368305,-0.518085611577563,
16.3394086400234));
#84902=CARTESIAN_POINT('Ctrl Pts',(9.34612360690806,-0.694953100015896,
16.3364875781861));
#84903=CARTESIAN_POINT('Ctrl Pts',(9.32574054154149,-0.913187127621161,
16.3328882216055));
#84904=CARTESIAN_POINT('Ctrl Pts',(9.32155575686584,-0.95495845525837,16.3321995426532));
#84905=CARTESIAN_POINT('Ctrl Pts',(9.29268786405095,-1.2248136761063,16.3277493466816));
#84906=CARTESIAN_POINT('Ctrl Pts',(9.25991608958468,-1.45195391693056,16.3239962271645));
#84907=CARTESIAN_POINT('Ctrl Pts',(9.19892194793587,-1.78712002499303,16.318364985256));
#84908=CARTESIAN_POINT('Ctrl Pts',(9.17705466648271,-1.89621479923809,16.3165175938012));
#84909=CARTESIAN_POINT('Ctrl Pts',(9.13215258815439,-2.10121313163741,16.3130112856188));
#84910=CARTESIAN_POINT('Ctrl Pts',(9.10953623704109,-2.1971929825401,16.3113550694203));
#84911=CARTESIAN_POINT('Ctrl Pts',(9.06611131269506,-2.36926799417323,16.3083562797361));
#84912=CARTESIAN_POINT('Ctrl Pts',(9.04584861607053,-2.4454913502132,16.3070174150153));
#84913=CARTESIAN_POINT('Ctrl Pts',(8.99855204910986,-2.61477247145234,16.3040194966337));
#84914=CARTESIAN_POINT('Ctrl Pts',(8.97103204148134,-2.70768500896524,16.3023573706975));
#84915=CARTESIAN_POINT('Ctrl Pts',(8.86763496968194,-3.03787560972726,16.2963907004436));
#84916=CARTESIAN_POINT('Ctrl Pts',(8.78374417735473,-3.27253351165463,16.2920362852277));
#84917=CARTESIAN_POINT('Ctrl Pts',(8.57638338538348,-3.78689208258241,16.2822948866805));
#84918=CARTESIAN_POINT('Ctrl Pts',(8.44837630966893,-4.06446080939157,16.2769011145216));
#84919=CARTESIAN_POINT('Ctrl Pts',(8.27909160684131,-4.38883544321028,16.2705827134957));
#84920=CARTESIAN_POINT('Ctrl Pts',(8.25062494498381,-4.44211913651728,16.2695445616066));
#84921=CARTESIAN_POINT('Ctrl Pts',(8.20141655799285,-4.53212197000876,16.2677928406647));
#84922=CARTESIAN_POINT('Ctrl Pts',(8.18093866352746,-4.56898300552095,16.2670760757343));
#84923=CARTESIAN_POINT('Ctrl Pts',(8.13252582853682,-4.65475902563531,16.2654097281733));
#84924=CARTESIAN_POINT('Ctrl Pts',(8.10439730127077,-4.70356272855464,16.2644625700254));
#84925=CARTESIAN_POINT('Ctrl Pts',(7.98427441283909,-4.90770196235974,16.2604988675927));
#84926=CARTESIAN_POINT('Ctrl Pts',(7.88824070472727,-5.06061611109365,16.257524516251));
#84927=CARTESIAN_POINT('Ctrl Pts',(7.64694809538953,-5.42125185958143,16.2504008340038));
#84928=CARTESIAN_POINT('Ctrl Pts',(7.49756290821882,-5.62604099934838,16.2462628871382));
#84929=CARTESIAN_POINT('Ctrl Pts',(7.26794283967614,-5.9154081121667,16.2401627114989));
#84930=CARTESIAN_POINT('Ctrl Pts',(7.19414196812091,-6.00494525522994,16.2382381314519));
#84931=CARTESIAN_POINT('Ctrl Pts',(7.05275037422716,-6.17013635214738,16.234608125144));
#84932=CARTESIAN_POINT('Ctrl Pts',(6.98555675143945,-6.24610816840465,16.2329058756864));
#84933=CARTESIAN_POINT('Ctrl Pts',(6.86388115370386,-6.37925972460924,16.229859750427));
#84934=CARTESIAN_POINT('Ctrl Pts',(6.80988454728909,-6.43686970080591,16.2285201418467));
#84935=CARTESIAN_POINT('Ctrl Pts',(6.68966418889043,-6.5619289479247,16.2255629386361));
#84936=CARTESIAN_POINT('Ctrl Pts',(6.62313490120561,-6.62907252195861,16.2239427394424));
#84937=CARTESIAN_POINT('Ctrl Pts',(6.25090007311462,-6.99354615576505,16.2149657535695));
#84938=CARTESIAN_POINT('Ctrl Pts',(5.92618796862801,-7.27074490740096,16.2074292034106));
#84939=CARTESIAN_POINT('Ctrl Pts',(5.46297211156788,-7.61446869719605,16.1973207054333));
#84940=CARTESIAN_POINT('Ctrl Pts',(5.34007191773079,-7.70115770261324,16.1946977411072));
#84941=CARTESIAN_POINT('Ctrl Pts',(5.17038991504525,-7.8148291275132,16.1911796533957));
#84942=CARTESIAN_POINT('Ctrl Pts',(5.12538346545211,-7.84442034286915,16.1902561574537));
#84943=CARTESIAN_POINT('Ctrl Pts',(5.04441390457464,-7.89666255626724,16.1886136088818));
#84944=CARTESIAN_POINT('Ctrl Pts',(5.00854723078353,-7.91945994406787,16.1878927193168));
#84945=CARTESIAN_POINT('Ctrl Pts',(4.92661405052329,-7.97075864390634,16.1862603800322));
#84946=CARTESIAN_POINT('Ctrl Pts',(4.88045300067559,-7.99910606801568,16.1853508569566));
#84947=CARTESIAN_POINT('Ctrl Pts',(4.57086839635086,-8.18554401717489,16.1793101140676));
#84948=CARTESIAN_POINT('Ctrl Pts',(4.30005163390314,-8.33099791695939,16.1743028689377));
#84949=CARTESIAN_POINT('Ctrl Pts',(3.86709982593019,-8.53678859425633,16.1664389556998));
#84950=CARTESIAN_POINT('Ctrl Pts',(3.70961335697883,-8.6063923424553,16.1636075506105));
#84951=CARTESIAN_POINT('Ctrl Pts',(3.49310126985347,-8.69503585929266,16.1597267852866));
#84952=CARTESIAN_POINT('Ctrl Pts',(3.43567295285092,-8.71788715365546,16.1586986310291));
#84953=CARTESIAN_POINT('Ctrl Pts',(3.28268972839102,-8.77701425376229,16.1559611555106));
#84954=CARTESIAN_POINT('Ctrl Pts',(3.18676035955294,-8.81229762359147,16.1542460009714));
#84955=CARTESIAN_POINT('Ctrl Pts',(3.01569577931341,-8.87205751639885,16.1511863175207));
#84956=CARTESIAN_POINT('Ctrl Pts',(2.94079200790026,-8.89716628709695,16.1498462123963));
#84957=CARTESIAN_POINT('Ctrl Pts',(2.77615015947903,-8.9500501764275,16.1468987401513));
#84958=CARTESIAN_POINT('Ctrl Pts',(2.68629379737132,-8.97742911121932,16.1452888854231));
#84959=CARTESIAN_POINT('Ctrl Pts',(2.39755486011037,-9.06068363760305,16.1401117634759));
#84960=CARTESIAN_POINT('Ctrl Pts',(2.19723094552465,-9.11133541096132,16.1365125147237));
#84961=CARTESIAN_POINT('Ctrl Pts',(1.74989549431628,-9.2088319102773,16.1284872782335));
#84962=CARTESIAN_POINT('Ctrl Pts',(1.50234069437424,-9.25244247241578,16.1240532110747));
#84963=CARTESIAN_POINT('Ctrl Pts',(1.16502267084434,-9.29797010508297,16.1181009250778));
#84964=CARTESIAN_POINT('Ctrl Pts',(1.07654636089967,-9.30862900100692,16.1165482987409));
#84965=CARTESIAN_POINT('Ctrl Pts',(0.919762059057807,-9.32525185256086,
16.1138188382958));
#84966=CARTESIAN_POINT('Ctrl Pts',(0.851515331387109,-9.33173113801424,
16.1126380449183));
#84967=CARTESIAN_POINT('Ctrl Pts',(0.740487244954019,-9.3410439043735,16.1107320679288));
#84968=CARTESIAN_POINT('Ctrl Pts',(0.69774679075457,-9.34433368525447,16.1100020326202));
#84969=CARTESIAN_POINT('Ctrl Pts',(0.603014675231229,-9.35097174350932,
16.1083927425419));
#84970=CARTESIAN_POINT('Ctrl Pts',(0.551014728230223,-9.35417992300858,
16.1075149935758));
#84971=CARTESIAN_POINT('Ctrl Pts',(0.373433854733403,-9.36365001289734,
16.1045328374649));
#84972=CARTESIAN_POINT('Ctrl Pts',(0.247754654171279,-9.36781789927196,
16.1024483570671));
#84973=CARTESIAN_POINT('Ctrl Pts',(-0.178748909620081,-9.37337275888033,
16.0954148305606));
#84974=CARTESIAN_POINT('Ctrl Pts',(-0.479541597051895,-9.36280451559987,
16.0905171298384));
#84975=CARTESIAN_POINT('Ctrl Pts',(-0.862682952782038,-9.33082866763476,
16.0841771922614));
#84976=CARTESIAN_POINT('Ctrl Pts',(-0.945964686502081,-9.32275368585295,
16.0827934093149));
#84977=CARTESIAN_POINT('Ctrl Pts',(-1.08744835825269,-9.30712007235797,
16.0804295026583));
#84978=CARTESIAN_POINT('Ctrl Pts',(-1.14570784493946,-9.30012803652572,
16.0794523338354));
#84979=CARTESIAN_POINT('Ctrl Pts',(-1.3018530011159,-9.27989871202747,16.0768217956801));
#84980=CARTESIAN_POINT('Ctrl Pts',(-1.39960128038713,-9.26566012414879,
16.0751627770707));
#84981=CARTESIAN_POINT('Ctrl Pts',(-1.57496288897138,-9.23727759940475,
16.0721611575476));
#84982=CARTESIAN_POINT('Ctrl Pts',(-1.65265746572546,-9.22369388138638,
16.0708222994514));
#84983=CARTESIAN_POINT('Ctrl Pts',(-1.82524531056657,-9.19126883326174,
16.0678271622371));
#84984=CARTESIAN_POINT('Ctrl Pts',(-1.92003696256901,-9.17193552151032,
16.0661678418955));
#84985=CARTESIAN_POINT('Ctrl Pts',(-2.25233651167558,-9.09878380443507,
16.0603005317881));
#84986=CARTESIAN_POINT('Ctrl Pts',(-2.48802880309683,-9.03717867421254,
16.0560453134387));
#84987=CARTESIAN_POINT('Ctrl Pts',(-2.89213241007543,-8.91454536325154,
16.0486288738686));
#84988=CARTESIAN_POINT('Ctrl Pts',(-3.06169156952756,-8.85774201750675,
16.0454798163883));
#84989=CARTESIAN_POINT('Ctrl Pts',(-3.36870308004292,-8.74502186423979,
16.0397492884474));
#84990=CARTESIAN_POINT('Ctrl Pts',(-3.50665246994715,-8.69062463295451,
16.037163689291));
#84991=CARTESIAN_POINT('Ctrl Pts',(-3.69270650274365,-8.61210688181122,
16.033685403748));
#84992=CARTESIAN_POINT('Ctrl Pts',(-3.74197970608444,-8.59081219419687,
16.032765149478));
#84993=CARTESIAN_POINT('Ctrl Pts',(-3.82996034720434,-8.55188853669681,
16.0311253268392));
#84994=CARTESIAN_POINT('Ctrl Pts',(-3.86873572972371,-8.53441724190768,
16.0304039613926));
#84995=CARTESIAN_POINT('Ctrl Pts',(-3.9568277213642,-8.49400128814837,16.0287674492606));
#84996=CARTESIAN_POINT('Ctrl Pts',(-4.00606618446022,-8.47088999116988,
16.0278542670405));
#84997=CARTESIAN_POINT('Ctrl Pts',(-4.31011536622006,-8.32493299142422,
16.0222172156383));
#84998=CARTESIAN_POINT('Ctrl Pts',(-4.55945676453774,-8.19102918162043,
16.0175981848308));
#84999=CARTESIAN_POINT('Ctrl Pts',(-4.81644832639015,-8.03764143406757,
16.0126912699411));
#85000=CARTESIAN_POINT('Ctrl Pts',(-4.83051592478062,-8.02919486647417,
16.0124222065597));
#85001=CARTESIAN_POINT('Ctrl Pts',(-4.99534124367152,-7.92963931384419,
16.0092640065528));
#85002=CARTESIAN_POINT('Ctrl Pts',(-5.14352296018176,-7.8343337423779,16.006368115123));
#85003=CARTESIAN_POINT('Ctrl Pts',(-5.39852713277017,-7.65996849923668,
16.0012455081852));
#85004=CARTESIAN_POINT('Ctrl Pts',(-5.50651907508048,-7.58270796968518,
15.9990303970227));
#85005=CARTESIAN_POINT('Ctrl Pts',(-5.67910349282999,-7.45360436703456,
15.9954058084714));
#85006=CARTESIAN_POINT('Ctrl Pts',(-5.74471459781343,-7.40315396936248,
15.994007355565));
#85007=CARTESIAN_POINT('Ctrl Pts',(-5.87497382561442,-7.30021916203003,
15.991187934991));
#85008=CARTESIAN_POINT('Ctrl Pts',(-5.93960795857675,-7.2477289218264,15.9897670075863));
#85009=CARTESIAN_POINT('Ctrl Pts',(-6.10805686349279,-7.10716252253127,
15.9860046570422));
#85010=CARTESIAN_POINT('Ctrl Pts',(-6.21066640580657,-7.01767343262509,
15.9836519935949));
#85011=CARTESIAN_POINT('Ctrl Pts',(-6.55220899096653,-6.70644326921703,
15.9756163210451));
#85012=CARTESIAN_POINT('Ctrl Pts',(-6.78150918809198,-6.4744849912915,15.9698612963954));
#85013=CARTESIAN_POINT('Ctrl Pts',(-7.10246121855436,-6.11401557726361,
15.9613991920208));
#85014=CARTESIAN_POINT('Ctrl Pts',(-7.20371591262726,-5.99438229713728,
15.9586640429115));
#85015=CARTESIAN_POINT('Ctrl Pts',(-7.33600669269451,-5.82988411490018,
15.9550270576576));
#85016=CARTESIAN_POINT('Ctrl Pts',(-7.36972092689752,-5.78720627472664,
15.9540943694905));
#85017=CARTESIAN_POINT('Ctrl Pts',(-7.42906577083377,-5.71072378941442,
15.9524439484673));
#85018=CARTESIAN_POINT('Ctrl Pts',(-7.45484186933651,-5.67703418440411,
15.9517242662979));
#85019=CARTESIAN_POINT('Ctrl Pts',(-7.51918623003714,-5.59174156425845,
15.94991981167));
#85020=CARTESIAN_POINT('Ctrl Pts',(-7.55745273731492,-5.53991366672258,
15.9488391351669));
#85021=CARTESIAN_POINT('Ctrl Pts',(-7.70643218282382,-5.33372036898968,
15.9445935478327));
#85022=CARTESIAN_POINT('Ctrl Pts',(-7.81297495879755,-5.17639765267232,
15.9414709713661));
#85023=CARTESIAN_POINT('Ctrl Pts',(-8.04118813872398,-4.81629996874281,
15.934478420199));
#85024=CARTESIAN_POINT('Ctrl Pts',(-8.1601147017571,-4.61193885824473,15.9306136914542));
#85025=CARTESIAN_POINT('Ctrl Pts',(-8.30616009651294,-4.33760629751067,
15.9254780298822));
#85026=CARTESIAN_POINT('Ctrl Pts',(-8.34034956838809,-4.27149774643698,
15.9242445278765));
#85027=CARTESIAN_POINT('Ctrl Pts',(-8.42556261749079,-4.10180584325191,
15.9210853616981));
#85028=CARTESIAN_POINT('Ctrl Pts',(-8.47546570838047,-3.99767401489658,
15.9191532724041));
#85029=CARTESIAN_POINT('Ctrl Pts',(-8.55679664914613,-3.81958986170785,
15.9158543845303));
#85030=CARTESIAN_POINT('Ctrl Pts',(-8.58922099584045,-3.74610708015055,
15.9144947122147));
#85031=CARTESIAN_POINT('Ctrl Pts',(-8.65491605529649,-3.59188492248353,
15.9116430500496));
#85032=CARTESIAN_POINT('Ctrl Pts',(-8.68801092646013,-3.51107893916356,
15.9101499901404));
#85033=CARTESIAN_POINT('Ctrl Pts',(-8.78027370323774,-3.27651029281188,
15.9058184116452));
#85034=CARTESIAN_POINT('Ctrl Pts',(-8.83652197419855,-3.12163500985146,
15.9029611601497));
#85035=CARTESIAN_POINT('Ctrl Pts',(-8.93509828852161,-2.82615259307612,
15.8975234305245));
#85036=CARTESIAN_POINT('Ctrl Pts',(-8.97826216947224,-2.68587568938342,
15.8949476755025));
#85037=CARTESIAN_POINT('Ctrl Pts',(-9.07003165260838,-2.36064832172299,
15.8890077995921));
#85038=CARTESIAN_POINT('Ctrl Pts',(-9.11630640308529,-2.17510743230606,
15.8856420940714));
#85039=CARTESIAN_POINT('Ctrl Pts',(-9.17356775207786,-1.91139477540088,
15.8809321505888));
#85040=CARTESIAN_POINT('Ctrl Pts',(-9.18929349213915,-1.83430107689474,
15.8795641882862));
#85041=CARTESIAN_POINT('Ctrl Pts',(-9.21582413948716,-1.69532170627578,
15.8771189323152));
#85042=CARTESIAN_POINT('Ctrl Pts',(-9.22698118336977,-1.63350804274296,
15.8760387248672));
#85043=CARTESIAN_POINT('Ctrl Pts',(-9.24454578964052,-1.53026631886198,
15.8742493150969));
#85044=CARTESIAN_POINT('Ctrl Pts',(-9.25129834930941,-1.48889916765478,
15.8735363683235));
#85045=CARTESIAN_POINT('Ctrl Pts',(-9.26615189226422,-1.39389959494387,
15.8719086043672));
#85046=CARTESIAN_POINT('Ctrl Pts',(-9.27406519000285,-1.34023947143676,
15.8709958434625));
#85047=CARTESIAN_POINT('Ctrl Pts',(-9.30307803061953,-1.13092723939612,
15.8674565590222));
#85048=CARTESIAN_POINT('Ctrl Pts',(-9.32072841432442,-0.974822735321517,
15.8648620125391));
#85049=CARTESIAN_POINT('Ctrl Pts',(-9.35829827594381,-0.546284030860297,
15.8577888096516));
#85050=CARTESIAN_POINT('Ctrl Pts',(-9.37024418740387,-0.27330729227416,
15.8533345246508));
#85051=CARTESIAN_POINT('Ctrl Pts',(-9.37025356323642,0.167381950165816,
15.8460620169799));
#85052=CARTESIAN_POINT('Ctrl Pts',(-9.36576149366356,0.334932770290093,
15.8432789744368));
#85053=CARTESIAN_POINT('Ctrl Pts',(-9.35207842141409,0.589833238234219,
15.8389972685167));
#85054=CARTESIAN_POINT('Ctrl Pts',(-9.34614929998464,0.67732360578869,15.8375191778604));
#85055=CARTESIAN_POINT('Ctrl Pts',(-9.33244939828673,0.844631469072172,
15.8346744278891));
#85056=CARTESIAN_POINT('Ctrl Pts',(-9.32488025672346,0.924457815456634,
15.8333091841404));
#85057=CARTESIAN_POINT('Ctrl Pts',(-9.304027518363,1.11791982015351,15.8299803229));
#85058=CARTESIAN_POINT('Ctrl Pts',(-9.28968552131401,1.23142827823779,15.828010210307));
#85059=CARTESIAN_POINT('Ctrl Pts',(-9.26273907565275,1.41726287271645,15.8247576515957));
#85060=CARTESIAN_POINT('Ctrl Pts',(-9.25135676604782,1.48975407358555,15.8234821009583));
#85061=CARTESIAN_POINT('Ctrl Pts',(-9.2007427136253,1.78911283046138,15.8181886459976));
#85062=CARTESIAN_POINT('Ctrl Pts',(-9.15400777384044,2.01462961897199,15.8141369440333));
#85063=CARTESIAN_POINT('Ctrl Pts',(-9.09234931818992,2.26529194695014,15.8096000269021));
#85064=CARTESIAN_POINT('Ctrl Pts',(-9.08556296639746,2.29235889705144,15.80910971416));
#85065=CARTESIAN_POINT('Ctrl Pts',(-9.03194861919503,2.50221800996891,15.8053056703467));
#85066=CARTESIAN_POINT('Ctrl Pts',(-8.97972952517669,2.68358879427491,15.8020024326592));
#85067=CARTESIAN_POINT('Ctrl Pts',(-8.90499334285409,2.91647076131029,15.797784950666));
#85068=CARTESIAN_POINT('Ctrl Pts',(-8.88744105032833,2.96952853735195,15.7968257856545));
#85069=CARTESIAN_POINT('Ctrl Pts',(-8.85580758261927,3.06235805249446,15.7951525281267));
#85070=CARTESIAN_POINT('Ctrl Pts',(-8.84193055550554,3.10219742113524,15.7944361673277));
#85071=CARTESIAN_POINT('Ctrl Pts',(-8.80734745982603,3.19936412141319,15.7926928924964));
#85072=CARTESIAN_POINT('Ctrl Pts',(-8.78635021194856,3.25658564094406,15.7916693615523));
#85073=CARTESIAN_POINT('Ctrl Pts',(-8.68355102012543,3.52849969874744,15.7868120236144));
#85074=CARTESIAN_POINT('Ctrl Pts',(-8.59442944174783,3.74034112336728,15.7830451638138));
#85075=CARTESIAN_POINT('Ctrl Pts',(-8.36675180305747,4.23030483455728,15.7741890389838));
#85076=CARTESIAN_POINT('Ctrl Pts',(-8.22197364695728,4.50523734701086,15.7691021879588));
#85077=CARTESIAN_POINT('Ctrl Pts',(-8.01255894856545,4.85907514277056,15.7622386246166));
#85078=CARTESIAN_POINT('Ctrl Pts',(-7.95991245021477,4.94484639474211,15.7605497449081));
#85079=CARTESIAN_POINT('Ctrl Pts',(-7.86348522324334,5.09641318705451,15.7575165383232));
#85080=CARTESIAN_POINT('Ctrl Pts',(-7.8202343906044,5.16253438455124,15.756176304074));
#85081=CARTESIAN_POINT('Ctrl Pts',(-7.72381733034893,5.30594282880879,15.7532309689126));
#85082=CARTESIAN_POINT('Ctrl Pts',(-7.67031626384744,5.38299468810639,15.7516234064154));
#85083=CARTESIAN_POINT('Ctrl Pts',(-7.4822445113779,5.64535620915769,15.7460622480555));
#85084=CARTESIAN_POINT('Ctrl Pts',(-7.34204351717437,5.82652778161682,15.7420670764762));
#85085=CARTESIAN_POINT('Ctrl Pts',(-7.04082143476646,6.18761743948393,15.733816031374));
#85086=CARTESIAN_POINT('Ctrl Pts',(-6.87920049817855,6.36681839973998,15.7295605562487));
#85087=CARTESIAN_POINT('Ctrl Pts',(-6.631600299452,6.620902905275,15.7233628608246));
#85088=CARTESIAN_POINT('Ctrl Pts',(-6.55088357298351,6.70077624879833,15.7213894181907));
#85089=CARTESIAN_POINT('Ctrl Pts',(-6.43114263043601,6.81503407580786,15.7185408880979));
#85090=CARTESIAN_POINT('Ctrl Pts',(-6.39325238808896,6.85059186536449,15.7176506872935));
#85091=CARTESIAN_POINT('Ctrl Pts',(-6.32354089130607,6.91492995526093,15.7160347061809));
#85092=CARTESIAN_POINT('Ctrl Pts',(-6.29181407858179,6.94381028604951,15.7153075049748));
#85093=CARTESIAN_POINT('Ctrl Pts',(-6.20866679389262,7.01845997636821,15.7134219517893));
#85094=CARTESIAN_POINT('Ctrl Pts',(-6.15693826418206,7.06388243403045,15.7122686115244));
#85095=CARTESIAN_POINT('Ctrl Pts',(-6.03670209454123,7.16713678806433,15.7096270636883));
#85096=CARTESIAN_POINT('Ctrl Pts',(-5.9678555492318,7.22456380063715,15.7081431401988));
#85097=CARTESIAN_POINT('Ctrl Pts',(-5.70013244705699,7.44144121742001,15.7024619433389));
#85098=CARTESIAN_POINT('Ctrl Pts',(-5.49560484848972,7.59373985443148,15.6983046173089));
#85099=CARTESIAN_POINT('Ctrl Pts',(-5.11764353183826,7.85190714034292,15.6907783993391));
#85100=CARTESIAN_POINT('Ctrl Pts',(-4.94649463491711,7.96083610739333,15.6874246305098));
#85101=CARTESIAN_POINT('Ctrl Pts',(-4.69137527066045,8.1118030086513,15.6824637778958));
#85102=CARTESIAN_POINT('Ctrl Pts',(-4.6100941510685,8.15827076323484,15.6808889699364));
#85103=CARTESIAN_POINT('Ctrl Pts',(-4.45894775038666,8.24169973553113,15.6779684005877));
#85104=CARTESIAN_POINT('Ctrl Pts',(-4.38928480825566,8.27901011048647,15.6766253458315));
#85105=CARTESIAN_POINT('Ctrl Pts',(-4.22807452093195,8.36274508994909,15.6735232980258));
#85106=CARTESIAN_POINT('Ctrl Pts',(-4.13621966528828,8.40855554793786,15.6717601236956));
#85107=CARTESIAN_POINT('Ctrl Pts',(-3.8189423435365,8.56033308520592,15.665685025036));
#85108=CARTESIAN_POINT('Ctrl Pts',(-3.59005814216845,8.65881659981613,15.6613255098028));
#85109=CARTESIAN_POINT('Ctrl Pts',(-3.08997590857638,8.85074912450476,15.651912879018));
#85110=CARTESIAN_POINT('Ctrl Pts',(-2.81785793593207,8.94110665445982,15.6468581113258));
#85111=CARTESIAN_POINT('Ctrl Pts',(-2.48235116529867,9.03567163966352,15.6408354451146));
#85112=CARTESIAN_POINT('Ctrl Pts',(-2.42250893029571,9.05189923693731,15.6397694073616));
#85113=CARTESIAN_POINT('Ctrl Pts',(-2.32163553941544,9.07818140482797,15.6379885954601));
#85114=CARTESIAN_POINT('Ctrl Pts',(-2.28068961480581,9.08855456564394,15.6372703021023));
#85115=CARTESIAN_POINT('Ctrl Pts',(-2.18522188514386,9.11205438695823,15.6356063438053));
#85116=CARTESIAN_POINT('Ctrl Pts',(-2.13064971155267,9.1249691322488,15.6346630487893));
#85117=CARTESIAN_POINT('Ctrl Pts',(-1.89810781504891,9.17780135525472,15.6306710703351));
#85118=CARTESIAN_POINT('Ctrl Pts',(-1.71910832552624,9.21300808442412,15.6276659755268));
#85119=CARTESIAN_POINT('Ctrl Pts',(-1.15510815692486,9.30692881872542,15.6182790533383));
#85120=CARTESIAN_POINT('Ctrl Pts',(-0.767408870734917,9.34688623888578,
15.6119296456137));
#85121=CARTESIAN_POINT('Ctrl Pts',(-0.284024001470532,9.36642020355662,
15.6038358871157));
#85122=CARTESIAN_POINT('Ctrl Pts',(-0.189645543171991,9.36880630477435,
15.6022483038232));
#85123=CARTESIAN_POINT('Ctrl Pts',(-0.016288041175524,9.37056855125156,
15.5993160680699));
#85124=CARTESIAN_POINT('Ctrl Pts',(0.0626781072318076,9.37037308196079,
15.5979742820961));
#85125=CARTESIAN_POINT('Ctrl Pts',(0.243186585160061,9.36764436726062,15.5948921573239));
#85126=CARTESIAN_POINT('Ctrl Pts',(0.344709074986845,9.36445814185987,15.5931478437941));
#85127=CARTESIAN_POINT('Ctrl Pts',(0.761531885481913,9.34458880828794,15.5859419970708));
#85128=CARTESIAN_POINT('Ctrl Pts',(1.07594183185033,9.31362541768284,15.5803951409329));
#85129=CARTESIAN_POINT('Ctrl Pts',(1.60482165262962,9.23439855919564,15.5709935129916));
#85130=CARTESIAN_POINT('Ctrl Pts',(1.82025330259932,9.19435955158589,15.5671457668868));
#85131=CARTESIAN_POINT('Ctrl Pts',(2.0963290126656,9.13296533618817,15.5622565085354));
#85132=CARTESIAN_POINT('Ctrl Pts',(2.15843161451212,9.11848804101339,15.561159569068));
#85133=CARTESIAN_POINT('Ctrl Pts',(2.26153797896965,9.09333963077009,15.5593457944175));
#85134=CARTESIAN_POINT('Ctrl Pts',(2.30262571044512,9.08302232331562,15.5586250823846));
#85135=CARTESIAN_POINT('Ctrl Pts',(2.39671545272811,9.05871651133231,15.5569797715574));
#85136=CARTESIAN_POINT('Ctrl Pts',(2.44966739368923,9.04454086578479,15.5560572739475));
#85137=CARTESIAN_POINT('Ctrl Pts',(2.65892101363595,8.98654958981423,15.5524204011845));
#85138=CARTESIAN_POINT('Ctrl Pts',(2.81419763513012,8.93914014082858,15.5497403583112));
#85139=CARTESIAN_POINT('Ctrl Pts',(3.27887686829661,8.7839547558277,15.5416877245926));
#85140=CARTESIAN_POINT('Ctrl Pts',(3.58393364941571,8.66396643681611,15.5363501164303));
#85141=CARTESIAN_POINT('Ctrl Pts',(4.00183291132801,8.47373771938385,15.5287346085468));
#85142=CARTESIAN_POINT('Ctrl Pts',(4.12042486130357,8.41670935804079,15.5265389735733));
#85143=CARTESIAN_POINT('Ctrl Pts',(4.25552198162736,8.34820421466785,15.5239913328453));
#85144=CARTESIAN_POINT('Ctrl Pts',(4.27323885690915,8.33914927352573,15.5236563045117));
#85145=CARTESIAN_POINT('Ctrl Pts',(4.29092662820214,8.330038039162,15.5233208859591));
#85146=CARTESIAN_POINT('',(-9.37024999994221,-3.29085560364655E-5,15.651410108095));
#85147=CARTESIAN_POINT('Ctrl Pts',(4.29092660882816,8.33003804914182,15.3259008099036));
#85148=CARTESIAN_POINT('Ctrl Pts',(4.14338165943684,8.40604064908272,15.3288132869415));
#85149=CARTESIAN_POINT('Ctrl Pts',(3.99382155619009,8.47812106179566,15.3317149276861));
#85150=CARTESIAN_POINT('Ctrl Pts',(3.79486872530126,8.56757098912454,15.3354781348473));
#85151=CARTESIAN_POINT('Ctrl Pts',(3.74715706517178,8.58854558352599,15.3363733892997));
#85152=CARTESIAN_POINT('Ctrl Pts',(3.66044193914147,8.6258064036087,15.337985915101));
#85153=CARTESIAN_POINT('Ctrl Pts',(3.62149862581783,8.64222882253731,15.3387047062237));
#85154=CARTESIAN_POINT('Ctrl Pts',(3.53091024838905,8.67971015704992,15.3403640552681));
#85155=CARTESIAN_POINT('Ctrl Pts',(3.47918572957726,8.7005725254746,15.3413023080991));
#85156=CARTESIAN_POINT('Ctrl Pts',(3.26264434492313,8.78567170098749,15.3451975990018));
#85157=CARTESIAN_POINT('Ctrl Pts',(3.09621109067015,8.84569684167798,15.3481136942107));
#85158=CARTESIAN_POINT('Ctrl Pts',(2.55131166892319,9.02495391183104,15.3575338867737));
#85159=CARTESIAN_POINT('Ctrl Pts',(2.16695257128601,9.12487264814757,15.3639998561766));
#85160=CARTESIAN_POINT('Ctrl Pts',(1.68509077809691,9.2179659879519,15.372211626545));
#85161=CARTESIAN_POINT('Ctrl Pts',(1.59249864456165,9.23441259087598,15.373793214));
#85162=CARTESIAN_POINT('Ctrl Pts',(1.4217037147495,9.26210467021329,15.3767199451349));
#85163=CARTESIAN_POINT('Ctrl Pts',(1.34357599216646,9.2737601809637,15.3780622972214));
#85164=CARTESIAN_POINT('Ctrl Pts',(1.16418493369478,9.29820814942461,15.3811535897687));
#85165=CARTESIAN_POINT('Ctrl Pts',(1.06284128407922,9.31033671164013,15.3829066001443));
#85166=CARTESIAN_POINT('Ctrl Pts',(0.899972766852598,9.32713447904183,15.385734302485));
#85167=CARTESIAN_POINT('Ctrl Pts',(0.838564682809169,9.33285582392137,15.3868028154152));
#85168=CARTESIAN_POINT('Ctrl Pts',(0.60613591919492,9.35219851453027,15.3908551729958));
#85169=CARTESIAN_POINT('Ctrl Pts',(0.434809019184202,9.36172840385953,15.3938593229248));
#85170=CARTESIAN_POINT('Ctrl Pts',(-0.0462849266090543,9.37525318514394,
15.4023127357885));
#85171=CARTESIAN_POINT('Ctrl Pts',(-0.356128831416666,9.36860113135022,
15.4077823653244));
#85172=CARTESIAN_POINT('Ctrl Pts',(-0.718523987558737,9.34281434062199,
15.4140537628747));
#85173=CARTESIAN_POINT('Ctrl Pts',(-0.771941332846491,9.33855251734523,
15.4149747451152));
#85174=CARTESIAN_POINT('Ctrl Pts',(-0.867576173558023,9.33009626181011,
15.4166157884542));
#85175=CARTESIAN_POINT('Ctrl Pts',(-0.909807239364471,9.32607288610909,
15.4173376204022));
#85176=CARTESIAN_POINT('Ctrl Pts',(-1.00609510332455,9.31623923279315,15.4189765648432));
#85177=CARTESIAN_POINT('Ctrl Pts',(-1.06013145991945,9.3102450078071,15.4198916726837));
#85178=CARTESIAN_POINT('Ctrl Pts',(-1.26945444804055,9.28517891965654,15.4234233371553));
#85179=CARTESIAN_POINT('Ctrl Pts',(-1.42430646756362,9.26268932466101,15.4260080656733));
#85180=CARTESIAN_POINT('Ctrl Pts',(-1.89972177579867,9.18143911745269,15.4339391924436));
#85181=CARTESIAN_POINT('Ctrl Pts',(-2.21783816644118,9.10982772513381,15.4392471254171));
#85182=CARTESIAN_POINT('Ctrl Pts',(-2.66285879524998,8.98495187757467,15.4469071235945));
#85183=CARTESIAN_POINT('Ctrl Pts',(-2.7933210807633,8.94525205912265,15.4491807988518));
#85184=CARTESIAN_POINT('Ctrl Pts',(-3.00200667067457,8.87673806215471,15.452873345799));
#85185=CARTESIAN_POINT('Ctrl Pts',(-3.08079304782268,8.84970264091211,15.4542803202716));
#85186=CARTESIAN_POINT('Ctrl Pts',(-3.23709628302548,8.7937271551059,15.4570989883812));
#85187=CARTESIAN_POINT('Ctrl Pts',(-3.31461123286781,8.7648035893701,15.4585104620641));
#85188=CARTESIAN_POINT('Ctrl Pts',(-3.5153101038635,8.68687249918063,15.4622013399725));
#85189=CARTESIAN_POINT('Ctrl Pts',(-3.63785482021707,8.63627067103908,15.4644911536243));
#85190=CARTESIAN_POINT('Ctrl Pts',(-3.92022880447052,8.51259439739314,15.4698489950298));
#85191=CARTESIAN_POINT('Ctrl Pts',(-4.07915837899617,8.43758993700404,15.47292706393));
#85192=CARTESIAN_POINT('Ctrl Pts',(-4.50612693615062,8.22120389245774,15.4813364207233));
#85193=CARTESIAN_POINT('Ctrl Pts',(-4.76956812564212,8.07122008554411,15.4866842231501));
#85194=CARTESIAN_POINT('Ctrl Pts',(-5.07018872589917,7.88020319686578,15.4928315089698));
#85195=CARTESIAN_POINT('Ctrl Pts',(-5.11485377660323,7.85128569091352,15.4937458660693));
#85196=CARTESIAN_POINT('Ctrl Pts',(-5.19464443469504,7.79865693552052,15.4953794827591));
#85197=CARTESIAN_POINT('Ctrl Pts',(-5.22986001849909,7.77508488734085,15.4961004489973));
#85198=CARTESIAN_POINT('Ctrl Pts',(-5.31017132640637,7.72053486786514,15.4977442422347));
#85199=CARTESIAN_POINT('Ctrl Pts',(-5.35515797613774,7.68939927632527,15.4986649908635));
#85200=CARTESIAN_POINT('Ctrl Pts',(-5.53135626676057,7.56515486078743,15.5022761904285));
#85201=CARTESIAN_POINT('Ctrl Pts',(-5.66043376802533,7.46906688071462,15.5049329300348));
#85202=CARTESIAN_POINT('Ctrl Pts',(-6.04432512846104,7.16762066575808,15.5129566813675));
#85203=CARTESIAN_POINT('Ctrl Pts',(-6.29091476325641,6.95219705395721,15.5182878564457));
#85204=CARTESIAN_POINT('Ctrl Pts',(-6.62095580651084,6.63190301697132,15.5259143344115));
#85205=CARTESIAN_POINT('Ctrl Pts',(-6.7142079554203,6.53747694566034,15.5281282640163));
#85206=CARTESIAN_POINT('Ctrl Pts',(-6.85664729006891,6.38698098219872,15.5316130428055));
#85207=CARTESIAN_POINT('Ctrl Pts',(-6.9072240032617,6.33225036368195,15.5328716280295));
#85208=CARTESIAN_POINT('Ctrl Pts',(-7.00726979730507,6.22136276646034,15.5354054517924));
#85209=CARTESIAN_POINT('Ctrl Pts',(-7.05672975127081,6.16520477137091,15.5366806469937));
#85210=CARTESIAN_POINT('Ctrl Pts',(-7.1581946305707,6.04717832442305,15.5393446860341));
#85211=CARTESIAN_POINT('Ctrl Pts',(-7.21008251642192,5.98521729999843,15.5407343566862));
#85212=CARTESIAN_POINT('Ctrl Pts',(-7.33508712685367,5.83196030945969,15.5441498466552));
#85213=CARTESIAN_POINT('Ctrl Pts',(-7.40730842900602,5.73995173823779,15.5461819925114));
#85214=CARTESIAN_POINT('Ctrl Pts',(-7.63353648519067,5.44035891165868,15.552734583431));
#85215=CARTESIAN_POINT('Ctrl Pts',(-7.7806841981848,5.22774686800166,15.5572911315491));
#85216=CARTESIAN_POINT('Ctrl Pts',(-8.01155606378281,4.86277943992659,15.5648713679657));
#85217=CARTESIAN_POINT('Ctrl Pts',(-8.10017274757297,4.71368817210393,15.5679036604525));
#85218=CARTESIAN_POINT('Ctrl Pts',(-8.2117572333541,4.51350629059428,15.5718560814117));
#85219=CARTESIAN_POINT('Ctrl Pts',(-8.23847763144406,4.46454725925851,15.5728135061304));
#85220=CARTESIAN_POINT('Ctrl Pts',(-8.28339881190472,4.38046275075152,15.5744403123562));
#85221=CARTESIAN_POINT('Ctrl Pts',(-8.30181710245382,4.3454553953276,15.5751123616867));
#85222=CARTESIAN_POINT('Ctrl Pts',(-8.33637823538616,4.27874381368598,15.5763832283343));
#85223=CARTESIAN_POINT('Ctrl Pts',(-8.3525631985838,4.24706236419942,15.5769826868324));
#85224=CARTESIAN_POINT('Ctrl Pts',(-8.41750174756852,4.11814058462066,15.5794070040464));
#85225=CARTESIAN_POINT('Ctrl Pts',(-8.4647408767115,4.02014670667257,15.581215203477));
#85226=CARTESIAN_POINT('Ctrl Pts',(-8.5877689860493,3.75314658120452,15.586074671246));
#85227=CARTESIAN_POINT('Ctrl Pts',(-8.66027093213542,3.58267958439453,15.5891062476071));
#85228=CARTESIAN_POINT('Ctrl Pts',(-8.76065627671584,3.32576308295427,15.5936276220563));
#85229=CARTESIAN_POINT('Ctrl Pts',(-8.79241269015809,3.24087604777668,15.5951137916613));
#85230=CARTESIAN_POINT('Ctrl Pts',(-8.89243744406557,2.96120563484695,15.5999964691581));
#85231=CARTESIAN_POINT('Ctrl Pts',(-8.95550230967423,2.76462665102001,15.6034081676231));
#85232=CARTESIAN_POINT('Ctrl Pts',(-9.03775390475236,2.47576583469663,15.6084337563054));
#85233=CARTESIAN_POINT('Ctrl Pts',(-9.06212307647707,2.3850235646686,15.6100139733665));
#85234=CARTESIAN_POINT('Ctrl Pts',(-9.10446240417055,2.21733842881238,15.6129394536193));
#85235=CARTESIAN_POINT('Ctrl Pts',(-9.12283196555392,2.14050514396401,15.6142819423674));
#85236=CARTESIAN_POINT('Ctrl Pts',(-9.15708425758601,1.98878161322273,15.6169377682931));
#85237=CARTESIAN_POINT('Ctrl Pts',(-9.17302514074449,1.91391069353834,15.6182506169118));
#85238=CARTESIAN_POINT('Ctrl Pts',(-9.20810113699684,1.73864932055023,15.6213291301637));
#85239=CARTESIAN_POINT('Ctrl Pts',(-9.22651484183486,1.63812448195104,15.6230989791019));
#85240=CARTESIAN_POINT('Ctrl Pts',(-9.28250340262572,1.30148774251282,15.6290362989418));
#85241=CARTESIAN_POINT('Ctrl Pts',(-9.31268635841509,1.06424248018041,15.6332399503902));
#85242=CARTESIAN_POINT('Ctrl Pts',(-9.35140417596125,0.626787906599619,
15.6409604976902));
#85243=CARTESIAN_POINT('Ctrl Pts',(-9.36265617330869,0.426957596360454,
15.6444750097962));
#85244=CARTESIAN_POINT('Ctrl Pts',(-9.36854682124597,0.183785776007762,
15.6486908625793));
#85245=CARTESIAN_POINT('Ctrl Pts',(-9.36929377931046,0.140644366409776,
15.6494364201494));
#85246=CARTESIAN_POINT('Ctrl Pts',(-9.37008099742837,0.0649922206876054,
15.6507388237825));
#85247=CARTESIAN_POINT('Ctrl Pts',(-9.37025008779887,0.0324835742681818,
15.651296864785));
#85248=CARTESIAN_POINT('Ctrl Pts',(-9.3702499999658,-2.53166982348E-5,15.65185308165));
#85249=CARTESIAN_POINT('Ctrl Pts',(-9.37024999994221,-3.29085560364655E-5,
15.651410108095));
#85250=CARTESIAN_POINT('Ctrl Pts',(-9.37024988706599,-0.0321728302279683,
15.6519561937273));
#85251=CARTESIAN_POINT('Ctrl Pts',(-9.37008441347547,-0.0643126166714824,
15.6525022793597));
#85252=CARTESIAN_POINT('Ctrl Pts',(-9.36975358934515,-0.0964506996016772,
15.653048364992));
#85253=CARTESIAN_POINT('Ctrl Pts',(-9.36734961314108,-0.32998622355172,
15.6570165666596));
#85254=CARTESIAN_POINT('Ctrl Pts',(-9.35620981951031,-0.563468090583012,
15.6609847683271));
#85255=CARTESIAN_POINT('Ctrl Pts',(-9.33635895696654,-0.796232685319189,
15.6649529699946));
#85256=CARTESIAN_POINT('Ctrl Pts',(-9.31651157239417,-1.02895649852255,
15.6689204764132));
#85257=CARTESIAN_POINT('Ctrl Pts',(-9.28795618961534,-1.26096300696166,
15.6728879828317));
#85258=CARTESIAN_POINT('Ctrl Pts',(-9.25076952484415,-1.49159252502647,
15.6768554892503));
#85259=CARTESIAN_POINT('Ctrl Pts',(-9.21358691453216,-1.7221968975726,15.6808225630919));
#85260=CARTESIAN_POINT('Ctrl Pts',(-9.16777494645078,-1.95142429874742,
15.6847896369335));
#85261=CARTESIAN_POINT('Ctrl Pts',(-9.11346183096947,-2.17862307845176,
15.6887567107752));
#85262=CARTESIAN_POINT('Ctrl Pts',(-9.05914448620663,-2.40583954978719,
15.6927240935269));
#85263=CARTESIAN_POINT('Ctrl Pts',(-8.99632473461012,-2.63102680662034,
15.6966914762787));
#85264=CARTESIAN_POINT('Ctrl Pts',(-8.92518154797546,-2.85354505802489,
15.7006588590305));
#85265=CARTESIAN_POINT('Ctrl Pts',(-8.85403911498194,-3.07606095222681,
15.7046261997546));
#85266=CARTESIAN_POINT('Ctrl Pts',(-8.77457351207394,-3.2959076272409,15.7085935404787));
#85267=CARTESIAN_POINT('Ctrl Pts',(-8.68701328200696,-3.5124614304978,15.7125608812028));
#85268=CARTESIAN_POINT('Ctrl Pts',(-8.59943420184895,-3.72906185376586,
15.7165290760216));
#85269=CARTESIAN_POINT('Ctrl Pts',(-8.50375711873428,-3.94236772478265,
15.7204972708405));
#85270=CARTESIAN_POINT('Ctrl Pts',(-8.4002588336377,-4.1517751131765,15.7244654656593));
#85271=CARTESIAN_POINT('Ctrl Pts',(-8.33662135806883,-4.28053239210552,
15.7269053698626));
#85272=CARTESIAN_POINT('Ctrl Pts',(-8.27002794412772,-4.40781622564588,
15.7293452740658));
#85273=CARTESIAN_POINT('Ctrl Pts',(-8.20055166581281,-4.5334906461616,15.7317851782691));
#85274=CARTESIAN_POINT('Ctrl Pts',(-8.08755711336536,-4.73788450899779,
15.7357533799366));
#85275=CARTESIAN_POINT('Ctrl Pts',(-7.96689962036225,-4.93808352651896,
15.7397215816041));
#85276=CARTESIAN_POINT('Ctrl Pts',(-7.83891604164744,-5.13351539926613,
15.7436897832716));
#85277=CARTESIAN_POINT('Ctrl Pts',(-7.71095488630218,-5.32891303136188,
15.7476572896901));
#85278=CARTESIAN_POINT('Ctrl Pts',(-7.57567036319796,-5.51954494802817,
15.7516247961087));
#85279=CARTESIAN_POINT('Ctrl Pts',(-7.43344319830096,-5.70486698180888,
15.7555923025272));
#85280=CARTESIAN_POINT('Ctrl Pts',(-7.2912315404208,-5.89016880994251,15.7595593763688));
#85281=CARTESIAN_POINT('Ctrl Pts',(-7.14207892523925,-6.07016168550439,
15.7635264502104));
#85282=CARTESIAN_POINT('Ctrl Pts',(-6.98640758373676,-6.24433296168658,
15.767493524052));
#85283=CARTESIAN_POINT('Ctrl Pts',(-6.83072412033846,-6.41851780032698,
15.7714609068038));
#85284=CARTESIAN_POINT('Ctrl Pts',(-6.66852110374997,-6.5868799197005,15.7754282895555));
#85285=CARTESIAN_POINT('Ctrl Pts',(-6.50025980967756,-6.74894121097455,
15.7793956723073));
#85286=CARTESIAN_POINT('Ctrl Pts',(-6.33200029804755,-6.9110007854847,15.7833630130314));
#85287=CARTESIAN_POINT('Ctrl Pts',(-6.15768284375902,-7.06675946964164,
15.7873303537554));
#85288=CARTESIAN_POINT('Ctrl Pts',(-5.97780468782581,-7.21577689349579,
15.7912976944795));
#85289=CARTESIAN_POINT('Ctrl Pts',(-5.79788780746694,-7.36482639803323,
15.7952658892984));
#85290=CARTESIAN_POINT('Ctrl Pts',(-5.61240805228575,-7.50713156048764,
15.7992340841172));
#85291=CARTESIAN_POINT('Ctrl Pts',(-5.42189577170874,-7.64229228067253,
15.803202278936));
#85292=CARTESIAN_POINT('Ctrl Pts',(-5.30475643370081,-7.72539788016028,
15.8056421831394));
#85293=CARTESIAN_POINT('Ctrl Pts',(-5.18571513404556,-7.80580326579222,
15.8080820873427));
#85294=CARTESIAN_POINT('Ctrl Pts',(-5.06490074054801,-7.88342346641966,
15.810521991546));
#85295=CARTESIAN_POINT('Ctrl Pts',(-4.86841110907637,-8.00966309875578,
15.8144901932135));
#85296=CARTESIAN_POINT('Ctrl Pts',(-4.66716894661539,-8.12857259914405,
15.8184583948811));
#85297=CARTESIAN_POINT('Ctrl Pts',(-4.46174243832586,-8.23980821843215,
15.8224265965486));
#85298=CARTESIAN_POINT('Ctrl Pts',(-4.25635192179843,-8.35102434867778,
15.8263941029671));
#85299=CARTESIAN_POINT('Ctrl Pts',(-4.04677877289066,-8.45456914623218,
15.8303616093857));
#85300=CARTESIAN_POINT('Ctrl Pts',(-3.83361643124384,-8.55014445027669,
15.8343291158042));
#85301=CARTESIAN_POINT('Ctrl Pts',(-3.62047733067052,-8.64570933375325,
15.8382961896458));
#85302=CARTESIAN_POINT('Ctrl Pts',(-3.4037500781858,-8.73330634226022,15.8422632634875));
#85303=CARTESIAN_POINT('Ctrl Pts',(-3.18404967662088,-8.81268476227934,
15.8462303373291));
#85304=CARTESIAN_POINT('Ctrl Pts',(-2.96433216731255,-8.89206936337792,
15.8501977200809));
#85305=CARTESIAN_POINT('Ctrl Pts',(-2.74164131289812,-8.96323399778914,
15.8541651028326));
#85306=CARTESIAN_POINT('Ctrl Pts',(-2.51661008151512,-9.02597688674841,
15.8581324855844));
#85307=CARTESIAN_POINT('Ctrl Pts',(-2.29158123395598,-9.08871911105329,
15.8620998263085));
#85308=CARTESIAN_POINT('Ctrl Pts',(-2.06421233366606,-9.14303969408616,
15.8660671670326));
#85309=CARTESIAN_POINT('Ctrl Pts',(-1.83515008414716,-9.18878714690653,
15.8700345077567));
#85310=CARTESIAN_POINT('Ctrl Pts',(-1.6060385217808,-9.23454444830373,15.8740027025755));
#85311=CARTESIAN_POINT('Ctrl Pts',(-1.37523316074441,-9.27172487541669,
15.8779708973944));
#85312=CARTESIAN_POINT('Ctrl Pts',(-1.14339072392327,-9.3002281001568,15.8819390922132));
#85313=CARTESIAN_POINT('Ctrl Pts',(-1.00083891839998,-9.317753736126,15.8843789964165));
#85314=CARTESIAN_POINT('Ctrl Pts',(-0.85789520831772,-9.33199988680165,
15.8868189006197));
#85315=CARTESIAN_POINT('Ctrl Pts',(-0.714713353468726,-9.34295295315531,
15.889258804823));
#85316=CARTESIAN_POINT('Ctrl Pts',(-0.481845819402004,-9.36076675752972,
15.8932270064905));
#85317=CARTESIAN_POINT('Ctrl Pts',(-0.248275795756671,-9.36987287027141,
15.8971952081581));
#85318=CARTESIAN_POINT('Ctrl Pts',(-0.0146665502080458,-9.37023852176694,
15.9011634098256));
#85319=CARTESIAN_POINT('Ctrl Pts',(0.218901765820847,-9.37060410919847,
15.9051309162442));
#85320=CARTESIAN_POINT('Ctrl Pts',(0.452509005685188,-9.36223229176214,
15.9090984226627));
#85321=CARTESIAN_POINT('Ctrl Pts',(0.685491319762012,-9.34514241266718,
15.9130659290813));
#85322=CARTESIAN_POINT('Ctrl Pts',(0.918448231795425,-9.32805439688039,
15.917033002923));
#85323=CARTESIAN_POINT('Ctrl Pts',(1.15078007046233,-9.30225023808432,15.9210000767646));
#85324=CARTESIAN_POINT('Ctrl Pts',(1.38182653551341,-9.26780127582864,15.9249671506063));
#85325=CARTESIAN_POINT('Ctrl Pts',(1.61289099180863,-9.23334963108358,15.928934533358));
#85326=CARTESIAN_POINT('Ctrl Pts',(1.84266959266458,-9.19025187685204,15.9329019161098));
#85327=CARTESIAN_POINT('Ctrl Pts',(2.0705094599306,-9.13863094992012,15.9368692988616));
#85328=CARTESIAN_POINT('Ctrl Pts',(2.29834691362034,-9.08701056982421,15.9408366395857));
#85329=CARTESIAN_POINT('Ctrl Pts',(2.52424539782052,-9.02686726265966,15.9448039803098));
#85330=CARTESIAN_POINT('Ctrl Pts',(2.74756382262737,-8.95837474674336,15.9487713210339));
#85331=CARTESIAN_POINT('Ctrl Pts',(2.97093032374271,-8.88986748566072,15.9527395158528));
#85332=CARTESIAN_POINT('Ctrl Pts',(3.19171538339562,-8.81300750727174,15.9567077106716));
#85333=CARTESIAN_POINT('Ctrl Pts',(3.40929338392328,-8.72801831373176,15.9606759054905));
#85334=CARTESIAN_POINT('Ctrl Pts',(3.54307448647365,-8.67576143119276,15.9631158096937));
#85335=CARTESIAN_POINT('Ctrl Pts',(3.6756434598503,-8.62043219518479,15.9655557138968));
#85336=CARTESIAN_POINT('Ctrl Pts',(3.80685852306037,-8.56209163977486,15.9679956181));
#85337=CARTESIAN_POINT('Ctrl Pts',(4.02026355427017,-8.46720795993301,15.9719638197674));
#85338=CARTESIAN_POINT('Ctrl Pts',(4.23015258035528,-8.36432708726278,15.9759320214349));
#85339=CARTESIAN_POINT('Ctrl Pts',(4.43592629921327,-8.2537350896699,15.9799002231023));
#85340=CARTESIAN_POINT('Ctrl Pts',(4.64166396547619,-8.14316246835367,15.9838677295208));
#85341=CARTESIAN_POINT('Ctrl Pts',(4.84328751329962,-8.02488155355912,15.9878352359392));
#85342=CARTESIAN_POINT('Ctrl Pts',(5.0402218707143,-7.89922455412386,15.9918027423577));
#85343=CARTESIAN_POINT('Ctrl Pts',(5.23713475639108,-7.77358125506161,15.9957698161992));
#85344=CARTESIAN_POINT('Ctrl Pts',(5.42935923271748,-7.64056363003513,15.9997368900408));
#85345=CARTESIAN_POINT('Ctrl Pts',(5.61634803854036,-7.50054796481456,16.0037039638823));
#85346=CARTESIAN_POINT('Ctrl Pts',(5.80335140490346,-7.36052139678237,16.007671346634));
#85347=CARTESIAN_POINT('Ctrl Pts',(5.98511805662897,-7.21349586788017,16.0116387293857));
#85348=CARTESIAN_POINT('Ctrl Pts',(6.16113176228737,-7.05988955085232,16.0156061121374));
#85349=CARTESIAN_POINT('Ctrl Pts',(6.33714360337977,-6.90628486102227,16.0195734528614));
#85350=CARTESIAN_POINT('Ctrl Pts',(6.50740240741105,-6.74609971124894,16.0235407935854));
#85351=CARTESIAN_POINT('Ctrl Pts',(6.67142642805035,-6.5797913703712,16.0275081343094));
#85352=CARTESIAN_POINT('Ctrl Pts',(6.83548576001426,-6.41344722639715,16.0314763291281));
#85353=CARTESIAN_POINT('Ctrl Pts',(6.99330742641979,-6.24097745961411,16.0354445239469));
#85354=CARTESIAN_POINT('Ctrl Pts',(7.14444693463981,-6.06287580778428,16.0394127187657));
#85355=CARTESIAN_POINT('Ctrl Pts',(7.23737733203747,-5.9533673313002,16.0418526229694));
#85356=CARTESIAN_POINT('Ctrl Pts',(7.32778222870503,-5.84173036731443,16.0442925271732));
#85357=CARTESIAN_POINT('Ctrl Pts',(7.41556582078254,-5.72808594734242,16.0467324313769));
#85358=CARTESIAN_POINT('Ctrl Pts',(7.55833494915475,-5.54325738884095,16.0507006330447));
#85359=CARTESIAN_POINT('Ctrl Pts',(7.69421269716705,-5.35305982094031,16.0546688347124));
#85360=CARTESIAN_POINT('Ctrl Pts',(7.82280743777052,-5.15802955149176,16.0586370363801));
#85361=CARTESIAN_POINT('Ctrl Pts',(7.95137964792578,-4.9630334523317,16.0626045427989));
#85362=CARTESIAN_POINT('Ctrl Pts',(8.0726712412503,-4.76320657916864,16.0665720492176));
#85363=CARTESIAN_POINT('Ctrl Pts',(8.18633382265112,-4.55911434454307,16.0705395556364));
#85364=CARTESIAN_POINT('Ctrl Pts',(8.29998401142945,-4.35504436207808,16.0745066294782));
#85365=CARTESIAN_POINT('Ctrl Pts',(8.40600671068612,-4.14671019513277,16.07847370332));
#85366=CARTESIAN_POINT('Ctrl Pts',(8.50409892869981,-3.93470284435645,16.0824407771619));
#85367=CARTESIAN_POINT('Ctrl Pts',(8.60219878500862,-3.72267898488307,16.0864081599139));
#85368=CARTESIAN_POINT('Ctrl Pts',(8.69236680400761,-3.50698162702699,16.0903755426658));
#85369=CARTESIAN_POINT('Ctrl Pts',(8.77434719056013,-3.28822390387419,16.0943429254178));
#85370=CARTESIAN_POINT('Ctrl Pts',(8.85632670866975,-3.06946849808776,16.0983102661421));
#85371=CARTESIAN_POINT('Ctrl Pts',(8.93011867006442,-2.84765305904123,16.1022776068664));
#85372=CARTESIAN_POINT('Ctrl Pts',(8.99551619221329,-2.62340875544175,16.1062449475907));
#85373=CARTESIAN_POINT('Ctrl Pts',(9.06092779323377,-2.39911617620958,16.1102131424097));
#85374=CARTESIAN_POINT('Ctrl Pts',(9.11794126387308,-2.1723939606798,16.1141813372288));
#85375=CARTESIAN_POINT('Ctrl Pts',(9.16639982352533,-1.94388768651246,16.1181495320479));
#85376=CARTESIAN_POINT('Ctrl Pts',(9.19619529696115,-1.80338717079906,16.1205894362499));
#85377=CARTESIAN_POINT('Ctrl Pts',(9.22275749985951,-1.66221243362113,16.1230293404519));
#85378=CARTESIAN_POINT('Ctrl Pts',(9.24605957875349,-1.52051548122368,16.1254692446539));
#85379=CARTESIAN_POINT('Ctrl Pts',(9.28395752090944,-1.29006295679158,16.129437446321));
#85380=CARTESIAN_POINT('Ctrl Pts',(9.31324122410686,-1.0581570665037,16.1334056479881));
#85381=CARTESIAN_POINT('Ctrl Pts',(9.33382064644945,-0.825455754364823,
16.1373738496552));
#85382=CARTESIAN_POINT('Ctrl Pts',(9.35439646317327,-0.592795212671557,
16.1413413560733));
#85383=CARTESIAN_POINT('Ctrl Pts',(9.36627101816281,-0.359339810557692,
16.1453088624915));
#85384=CARTESIAN_POINT('Ctrl Pts',(9.36940613650569,-0.125752581323693,
16.1492763689096));
#85385=CARTESIAN_POINT('Ctrl Pts',(9.37254091302685,0.107809179912775,16.1532434427508));
#85386=CARTESIAN_POINT('Ctrl Pts',(9.36693815158309,0.341502455215567,16.157210516592));
#85387=CARTESIAN_POINT('Ctrl Pts',(9.35261178570038,0.574663247892473,16.1611775904332));
#85388=CARTESIAN_POINT('Ctrl Pts',(9.33828430424486,0.807842196453683,16.1651449731845));
#85389=CARTESIAN_POINT('Ctrl Pts',(9.31523187552841,1.04048829538867,16.1691123559359));
#85390=CARTESIAN_POINT('Ctrl Pts',(9.28352047903083,1.27194047734756,16.1730797386872));
#85391=CARTESIAN_POINT('Ctrl Pts',(9.25180941846159,1.50339020746409,16.1770470794109));
#85392=CARTESIAN_POINT('Ctrl Pts',(9.2114396144082,1.73364576433429,16.1810144201346));
#85393=CARTESIAN_POINT('Ctrl Pts',(9.16252865747875,1.96205343030729,16.1849817608583));
#85394=CARTESIAN_POINT('Ctrl Pts',(9.1136071709288,2.19051026820809,16.1889499556767));
#85395=CARTESIAN_POINT('Ctrl Pts',(9.05614091651315,2.41711814193612,16.1929181504951));
#85396=CARTESIAN_POINT('Ctrl Pts',(8.99029842080894,2.64123444004886,16.1968863453136));
#85397=CARTESIAN_POINT('Ctrl Pts',(8.94981417304946,2.77903571326451,16.1993262495193));
#85398=CARTESIAN_POINT('Ctrl Pts',(8.90616420613945,2.91589526715953,16.2017661537251));
#85399=CARTESIAN_POINT('Ctrl Pts',(8.85939705632466,3.05166657105358,16.2042060579309));
#85400=CARTESIAN_POINT('Ctrl Pts',(8.78333608578722,3.27248176261888,16.2081742595991));
#85401=CARTESIAN_POINT('Ctrl Pts',(8.69900366671695,3.4904861670358,16.2121424612672));
#85402=CARTESIAN_POINT('Ctrl Pts',(8.60663293394173,3.70505797564485,16.2161106629354));
#85403=CARTESIAN_POINT('Ctrl Pts',(8.51427838498551,3.91959219018913,16.2200781693545));
#85404=CARTESIAN_POINT('Ctrl Pts',(8.41388844601816,4.13069474823769,16.2240456757737));
#85405=CARTESIAN_POINT('Ctrl Pts',(8.30574431645046,4.33776398761515,16.2280131821929));
#85406=CARTESIAN_POINT('Ctrl Pts',(8.19761197782881,4.54481065024951,16.2319802560351));
#85407=CARTESIAN_POINT('Ctrl Pts',(8.08172726827439,4.747824620156,16.2359473298774));
#85408=CARTESIAN_POINT('Ctrl Pts',(7.95841770537457,4.94622812750085,16.2399144037196));
#85409=CARTESIAN_POINT('Ctrl Pts',(7.83509854054274,5.14464708423132,16.243881786472));
#85410=CARTESIAN_POINT('Ctrl Pts',(7.70435351479008,5.33845461785254,16.2478491692244));
#85411=CARTESIAN_POINT('Ctrl Pts',(7.56655456068198,5.52710024721125,16.2518165519768));
#85412=CARTESIAN_POINT('Ctrl Pts',(7.42875706631973,5.71574387818997,16.2557838927015));
#85413=CARTESIAN_POINT('Ctrl Pts',(7.28390596267929,5.89922548585459,16.2597512334262));
#85414=CARTESIAN_POINT('Ctrl Pts',(7.13241511590066,6.077025561652,16.2637185741509));
#85415=CARTESIAN_POINT('Ctrl Pts',(6.98089165595732,6.25486391450231,16.2676867689704));
#85416=CARTESIAN_POINT('Ctrl Pts',(6.82272578088743,6.42701807455547,16.2716549637898));
#85417=CARTESIAN_POINT('Ctrl Pts',(6.65837091266764,6.59300249141781,16.2756231586093));
#85418=CARTESIAN_POINT('Ctrl Pts',(6.55731485281472,6.69506050373457,16.2780630628088));
#85419=CARTESIAN_POINT('Ctrl Pts',(6.45391974796182,6.79478667527731,16.2805029670084));
#85420=CARTESIAN_POINT('Ctrl Pts',(6.34829788533103,6.89207508821557,16.2829428712079));
#85421=CARTESIAN_POINT('Ctrl Pts',(6.1765156888821,7.05030385683692,16.286911103656));
#85422=CARTESIAN_POINT('Ctrl Pts',(5.99878819175189,7.20213159787593,16.2908793361041));
#85423=CARTESIAN_POINT('Ctrl Pts',(5.81561581276912,7.34712173444607,16.2948475685522));
#85424=CARTESIAN_POINT('Ctrl Pts',(5.63247800506067,7.49208450611647,16.2988150520508));
#85425=CARTESIAN_POINT('Ctrl Pts',(5.44389759010635,7.63021207327026,16.3027825355495));
#85426=CARTESIAN_POINT('Ctrl Pts',(5.25040770241951,7.76110842733651,16.3067500190481));
#85427=CARTESIAN_POINT('Ctrl Pts',(5.05692965561876,7.8919967710161,16.310717259751));
#85428=CARTESIAN_POINT('Ctrl Pts',(4.85854297054156,8.01565462433856,16.3146845004539));
#85429=CARTESIAN_POINT('Ctrl Pts',(4.65581028347088,8.13172894695997,16.3186517411569));
#85430=CARTESIAN_POINT('Ctrl Pts',(4.53566764739617,8.20051644887604,16.3210027915123));
#85431=CARTESIAN_POINT('Ctrl Pts',(4.41399926836326,8.26664148966478,16.3233538418677));
#85432=CARTESIAN_POINT('Ctrl Pts',(4.29092662815671,8.3300380391854,16.3257048922231));
#85433=CARTESIAN_POINT('Origin',(0.,0.,2.15141010809499));
#85434=CARTESIAN_POINT('',(4.29125029737385,8.33066558789108,17.5228836507406));
#85435=CARTESIAN_POINT('',(4.29092662815677,8.33003803918537,17.3256735943175));
#85436=CARTESIAN_POINT('',(4.29092662815669,8.33003803918541,2.15141010809499));
#85437=CARTESIAN_POINT('',(-9.36966006811048,0.00015743873267679,16.848589891905));
#85438=CARTESIAN_POINT('Ctrl Pts',(-9.36966006811048,0.00015743873267679,
16.848589891905));
#85439=CARTESIAN_POINT('Ctrl Pts',(-9.36907237380321,-0.963482148612044,
16.8649547993108));
#85440=CARTESIAN_POINT('Ctrl Pts',(-8.98390107505351,-3.47304054260515,
16.9075653111423));
#85441=CARTESIAN_POINT('Ctrl Pts',(-6.7782850671257,-7.0238660837389,16.9764214273993));
#85442=CARTESIAN_POINT('Ctrl Pts',(-2.630771112749,-9.39994023956942,17.0551582406763));
#85443=CARTESIAN_POINT('Ctrl Pts',(2.14758775784479,-9.52195992174593,17.1338950539533));
#85444=CARTESIAN_POINT('Ctrl Pts',(6.41096663338061,-7.36066081768614,17.2126318672303));
#85445=CARTESIAN_POINT('Ctrl Pts',(9.13702913819428,-3.43432004152829,17.2913686805072));
#85446=CARTESIAN_POINT('Ctrl Pts',(9.67208108851768,1.31556407398382,17.3701054937842));
#85447=CARTESIAN_POINT('Ctrl Pts',(7.92328567786768,5.66181210550089,17.4472771505287));
#85448=CARTESIAN_POINT('Ctrl Pts',(5.58235227426782,7.66474807205545,17.4982032028475));
#85449=CARTESIAN_POINT('Ctrl Pts',(4.29125029737042,8.33066558789285,17.5228836507406));
#85450=CARTESIAN_POINT('Ctrl Pts',(-9.3702499985761,0.0001633542619707,
16.8489304074991));
#85451=CARTESIAN_POINT('Ctrl Pts',(-9.37024181960975,0.469321358043213,
16.8407937247888));
#85452=CARTESIAN_POINT('Ctrl Pts',(-9.33499852673591,0.937813119156036,
16.8324468196874));
#85453=CARTESIAN_POINT('Ctrl Pts',(-9.25639715191407,1.45734889239428,16.8233336223895));
#85454=CARTESIAN_POINT('Ctrl Pts',(-9.24747481473559,1.5129321186541,16.8223610407942));
#85455=CARTESIAN_POINT('Ctrl Pts',(-9.23124416801755,1.60853052280593,16.8206942247754));
#85456=CARTESIAN_POINT('Ctrl Pts',(-9.22417518117763,1.64858471639062,16.819997660776));
#85457=CARTESIAN_POINT('Ctrl Pts',(-9.20921162645301,1.73026033840815,16.8185818235094));
#85458=CARTESIAN_POINT('Ctrl Pts',(-9.20129518058143,1.77187658187216,16.8178629924835));
#85459=CARTESIAN_POINT('Ctrl Pts',(-9.18075773030714,1.87598975018297,16.8160704694915));
#85460=CARTESIAN_POINT('Ctrl Pts',(-9.16778057927006,1.93841412578864,16.815000738157));
#85461=CARTESIAN_POINT('Ctrl Pts',(-9.11491148928658,2.18031555355801,16.8108672694784));
#85462=CARTESIAN_POINT('Ctrl Pts',(-9.07037770777503,2.3587360981436,16.8078432520672));
#85463=CARTESIAN_POINT('Ctrl Pts',(-8.95533634872791,2.76798486425719,16.8008689808035));
#85464=CARTESIAN_POINT('Ctrl Pts',(-8.88110353182279,2.99763061625038,16.7969256611321));
#85465=CARTESIAN_POINT('Ctrl Pts',(-8.75897437016394,3.33089735251735,16.7910615635904));
#85466=CARTESIAN_POINT('Ctrl Pts',(-8.7179181160513,3.43691909083854,16.789174844691));
#85467=CARTESIAN_POINT('Ctrl Pts',(-8.63795502644643,3.6327526524998,16.7856421045001));
#85468=CARTESIAN_POINT('Ctrl Pts',(-8.59955054522782,3.72275291062085,16.7839994136168));
#85469=CARTESIAN_POINT('Ctrl Pts',(-8.53210853098703,3.87418677894387,16.7811998233642));
#85470=CARTESIAN_POINT('Ctrl Pts',(-8.50379950769038,3.93593611410202,16.7800480700436));
#85471=CARTESIAN_POINT('Ctrl Pts',(-8.43654087258266,4.07853102900152,16.7773638869738));
#85472=CARTESIAN_POINT('Ctrl Pts',(-8.39709634887749,4.15913574051146,16.7758280646212));
#85473=CARTESIAN_POINT('Ctrl Pts',(-8.27955578858586,4.39083905292596,16.7713587749051));
#85474=CARTESIAN_POINT('Ctrl Pts',(-8.19849619758667,4.54039331501592,16.7684054560219));
#85475=CARTESIAN_POINT('Ctrl Pts',(-7.96784682624004,4.93960188790244,16.7603485331533));
#85476=CARTESIAN_POINT('Ctrl Pts',(-7.81062614248576,5.18462810757901,16.7552092857057));
#85477=CARTESIAN_POINT('Ctrl Pts',(-7.58757638156798,5.49901818483393,16.7484626723151));
#85478=CARTESIAN_POINT('Ctrl Pts',(-7.53172932983633,5.57526409224734,16.7468144912902));
#85479=CARTESIAN_POINT('Ctrl Pts',(-7.44238859463641,5.69344489683138,16.7442477448354));
#85480=CARTESIAN_POINT('Ctrl Pts',(-7.40967183700969,5.7359590366,16.7433218916292));
#85481=CARTESIAN_POINT('Ctrl Pts',(-7.35000236941168,5.81213467445593,16.741660079054));
#85482=CARTESIAN_POINT('Ctrl Pts',(-7.32317894333512,5.84589552402361,16.7409225255032));
#85483=CARTESIAN_POINT('Ctrl Pts',(-7.2691603902236,5.91292980191826,16.7394569802778));
#85484=CARTESIAN_POINT('Ctrl Pts',(-7.24196755441882,5.94620362577631,16.7387291305881));
#85485=CARTESIAN_POINT('Ctrl Pts',(-7.16830705656106,6.0350815989535,16.7367824920474));
#85486=CARTESIAN_POINT('Ctrl Pts',(-7.12142160299381,6.0903358161585,16.735569547554));
#85487=CARTESIAN_POINT('Ctrl Pts',(-6.83447510730782,6.42065596860322,16.7282841803512));
#85488=CARTESIAN_POINT('Ctrl Pts',(-6.57914634471105,6.68204374545883,16.7223612608149));
#85489=CARTESIAN_POINT('Ctrl Pts',(-6.21187474633604,7.01651851507457,16.7141799772493));
#85490=CARTESIAN_POINT('Ctrl Pts',(-6.11267336090889,7.10310806739002,16.712002314275));
#85491=CARTESIAN_POINT('Ctrl Pts',(-5.92704092455368,7.25837077997098,16.707971414249));
#85492=CARTESIAN_POINT('Ctrl Pts',(-5.8411576163619,7.32766252761595,16.7061231084371));
#85493=CARTESIAN_POINT('Ctrl Pts',(-5.69116614514037,7.44436467587544,16.7029184915326));
#85494=CARTESIAN_POINT('Ctrl Pts',(-5.62763971293949,7.49250350322979,16.7015682412572));
#85495=CARTESIAN_POINT('Ctrl Pts',(-5.49164506799169,7.59285159623958,16.6986912276238));
#85496=CARTESIAN_POINT('Ctrl Pts',(-5.41902888138777,7.64484707824218,16.6971629394608));
#85497=CARTESIAN_POINT('Ctrl Pts',(-5.20275508520661,7.79507592725685,16.6926338884447));
#85498=CARTESIAN_POINT('Ctrl Pts',(-5.05709197096571,7.89035421744078,16.689611842163));
#85499=CARTESIAN_POINT('Ctrl Pts',(-4.66266365935591,8.13293877463738,16.6815185091125));
#85500=CARTESIAN_POINT('Ctrl Pts',(-4.40959309941721,8.27288424482264,16.6764136668451));
#85501=CARTESIAN_POINT('Ctrl Pts',(-4.0296580003687,8.46059079840007,16.6689970363393));
#85502=CARTESIAN_POINT('Ctrl Pts',(-3.90758202608788,8.51766066103064,16.6666507852358));
#85503=CARTESIAN_POINT('Ctrl Pts',(-3.73641490031448,8.59322585855475,16.6634299495345));
#85504=CARTESIAN_POINT('Ctrl Pts',(-3.6883356067873,8.61397164098076,16.662532701195));
#85505=CARTESIAN_POINT('Ctrl Pts',(-3.60064640445006,8.65093997035938,16.6609113803635));
#85506=CARTESIAN_POINT('Ctrl Pts',(-3.56109454869803,8.66729614783114,16.6601857975763));
#85507=CARTESIAN_POINT('Ctrl Pts',(-3.45840695827095,8.7089397624329,16.6583156574734));
#85508=CARTESIAN_POINT('Ctrl Pts',(-3.39510543856361,8.73381185783161,16.6571759389361));
#85509=CARTESIAN_POINT('Ctrl Pts',(-3.1479506207643,8.82782950165556,16.65276749471));
#85510=CARTESIAN_POINT('Ctrl Pts',(-2.96221150961838,8.89187664179254,16.6495421735003));
#85511=CARTESIAN_POINT('Ctrl Pts',(-2.74130839687928,8.96035869497896,16.6457500761035));
#85512=CARTESIAN_POINT('Ctrl Pts',(-2.70796277882292,8.97049258726913,16.6451788475486));
#85513=CARTESIAN_POINT('Ctrl Pts',(-2.47711860808384,9.03924277036251,16.6412309906005));
#85514=CARTESIAN_POINT('Ctrl Pts',(-2.27779045042254,9.09151785806547,16.637854163583));
#85515=CARTESIAN_POINT('Ctrl Pts',(-2.00968994884745,9.15245771518472,16.6333040229718));
#85516=CARTESIAN_POINT('Ctrl Pts',(-1.9423114697882,9.16699307603529,16.6321599504571));
#85517=CARTESIAN_POINT('Ctrl Pts',(-1.76718873247439,9.2027543367994,16.6291824767245));
#85518=CARTESIAN_POINT('Ctrl Pts',(-1.65922095241976,9.22283194841569,16.6273428758723));
#85519=CARTESIAN_POINT('Ctrl Pts',(-1.47237979820681,9.2541896451788,16.6241479508398));
#85520=CARTESIAN_POINT('Ctrl Pts',(-1.39366937541875,9.26637004963315,16.6227985786645));
#85521=CARTESIAN_POINT('Ctrl Pts',(-1.22615237168245,9.29011055235098,16.6199182666768));
#85522=CARTESIAN_POINT('Ctrl Pts',(-1.13731597222442,9.30140398241826,16.6183857495498));
#85523=CARTESIAN_POINT('Ctrl Pts',(-0.866688774887697,9.33187269145,16.6137013502423));
#85524=CARTESIAN_POINT('Ctrl Pts',(-0.684487092087161,9.34700349990969,
16.6105251989289));
#85525=CARTESIAN_POINT('Ctrl Pts',(-0.377921660298956,9.36344969135507,
16.605155853724));
#85526=CARTESIAN_POINT('Ctrl Pts',(-0.253763164707002,9.36763679412889,
16.6029745812385));
#85527=CARTESIAN_POINT('Ctrl Pts',(0.058856776555768,9.37195966630942,16.597478690213));
#85528=CARTESIAN_POINT('Ctrl Pts',(0.247307739141228,9.36888099461859,16.5941618313608));
#85529=CARTESIAN_POINT('Ctrl Pts',(0.489174449052452,9.35762665287357,16.5899363554316));
#85530=CARTESIAN_POINT('Ctrl Pts',(0.542789030154573,9.35466986567322,16.5890017629769));
#85531=CARTESIAN_POINT('Ctrl Pts',(0.671531270746277,9.34645934096579,16.5867645333661));
#85532=CARTESIAN_POINT('Ctrl Pts',(0.746626902874601,9.34076039567737,16.5854652468591));
#85533=CARTESIAN_POINT('Ctrl Pts',(0.865303772421255,9.33031377999916,16.5834249399983));
#85534=CARTESIAN_POINT('Ctrl Pts',(0.908934374176971,9.32616449451436,16.5826776572712));
#85535=CARTESIAN_POINT('Ctrl Pts',(1.00170076526,9.3166852050695,16.5810957754857));
#85536=CARTESIAN_POINT('Ctrl Pts',(1.05082667328386,9.31127225197728,16.5802620590381));
#85537=CARTESIAN_POINT('Ctrl Pts',(1.20971099260783,9.29249211075097,16.5775754900517));
#85538=CARTESIAN_POINT('Ctrl Pts',(1.31927641995736,9.2775708110679,16.5757380271228));
#85539=CARTESIAN_POINT('Ctrl Pts',(1.66864671608303,9.22367715549834,16.5698962231511));
#85540=CARTESIAN_POINT('Ctrl Pts',(1.90721034479679,9.17731721296951,16.5659312652029));
#85541=CARTESIAN_POINT('Ctrl Pts',(2.3733181609767,9.06777708273342,16.5580711277267));
#85542=CARTESIAN_POINT('Ctrl Pts',(2.60081384248497,9.00516447289314,16.5541800554601));
#85543=CARTESIAN_POINT('Ctrl Pts',(2.91556770618963,8.90561246782929,16.54865674158));
#85544=CARTESIAN_POINT('Ctrl Pts',(3.00499773611537,8.87583556788492,16.5470716332787));
#85545=CARTESIAN_POINT('Ctrl Pts',(3.16850746490285,8.81863834914141,16.5441416784427));
#85546=CARTESIAN_POINT('Ctrl Pts',(3.2427190138618,8.79162074088098,16.5427996675298));
#85547=CARTESIAN_POINT('Ctrl Pts',(3.41014346238886,8.72825953560375,16.5397433138038));
#85548=CARTESIAN_POINT('Ctrl Pts',(3.50313365119126,8.6913547568976,16.5380253068828));
#85549=CARTESIAN_POINT('Ctrl Pts',(3.83165148774084,8.5548477509526,16.5318830065843));
#85550=CARTESIAN_POINT('Ctrl Pts',(4.0636487589826,8.44711225407878,16.527407502209));
#85551=CARTESIAN_POINT('Ctrl Pts',(4.29092663733566,8.33003803445718,16.522914704178));
#85552=CARTESIAN_POINT('',(-9.37024999773577,-0.000205992430197824,16.651410108095));
#85553=CARTESIAN_POINT('Ctrl Pts',(4.29092662815671,8.3300380391854,16.3257048922231));
#85554=CARTESIAN_POINT('Ctrl Pts',(4.08324528991728,8.43701778888531,16.3296722182125));
#85555=CARTESIAN_POINT('Ctrl Pts',(3.87156411057383,8.53622542790688,16.333639544202));
#85556=CARTESIAN_POINT('Ctrl Pts',(3.65648539798877,8.62738080745222,16.3376068701914));
#85557=CARTESIAN_POINT('Ctrl Pts',(3.43897743753376,8.71956575895721,16.341619005907));
#85558=CARTESIAN_POINT('Ctrl Pts',(3.21799499775753,8.8035153233757,16.3456311416225));
#85559=CARTESIAN_POINT('Ctrl Pts',(2.99418171318639,8.87898985982754,16.3496432773381));
#85560=CARTESIAN_POINT('Ctrl Pts',(2.77036842861529,8.95446439627936,16.3536554130537));
#85561=CARTESIAN_POINT('Ctrl Pts',(2.54372458648862,9.02146381586769,16.3576675487692));
#85562=CARTESIAN_POINT('Ctrl Pts',(2.31491039177459,9.07980037999482,16.3616796844848));
#85563=CARTESIAN_POINT('Ctrl Pts',(2.08860177878142,9.13749814184432,16.365647886152));
#85564=CARTESIAN_POINT('Ctrl Pts',(1.86009982710217,9.18673974318476,16.3696160878191));
#85565=CARTESIAN_POINT('Ctrl Pts',(1.63005222104112,9.22737854534965,16.3735842894863));
#85566=CARTESIAN_POINT('Ctrl Pts',(1.40004492048336,9.268010227391,16.3775517959044));
#85567=CARTESIAN_POINT('Ctrl Pts',(1.1684927861248,9.30004206946954,16.3815193023226));
#85568=CARTESIAN_POINT('Ctrl Pts',(0.936053060732539,9.32337866494723,16.3854868087407));
#85569=CARTESIAN_POINT('Ctrl Pts',(0.703638678226125,9.34671271603767,16.389453882582));
#85570=CARTESIAN_POINT('Ctrl Pts',(0.470337180866043,9.3613533849971,16.3934209564232));
#85571=CARTESIAN_POINT('Ctrl Pts',(0.236811280348955,9.36725709479565,16.3973880302644));
#85572=CARTESIAN_POINT('Ctrl Pts',(0.00326719551702451,9.37316126430731,
16.4013554130158));
#85573=CARTESIAN_POINT('Ctrl Pts',(-0.230501043047988,9.37032710511516,
16.4053227957672));
#85574=CARTESIAN_POINT('Ctrl Pts',(-0.463829138258932,9.35876314440119,
16.4092901785186));
#85575=CARTESIAN_POINT('Ctrl Pts',(-0.697154761755315,9.34719930618771,
16.4132575192423));
#85576=CARTESIAN_POINT('Ctrl Pts',(-0.930039967179378,9.32690586773196,
16.417224859966));
#85577=CARTESIAN_POINT('Ctrl Pts',(-1.16182331345612,9.29794340974443,16.4211922006897));
#85578=CARTESIAN_POINT('Ctrl Pts',(-1.39365655838131,9.26897471667775,16.4251603955081));
#85579=CARTESIAN_POINT('Ctrl Pts',(-1.6243871877291,9.23133330977507,16.4291285903266));
#85580=CARTESIAN_POINT('Ctrl Pts',(-1.85336041727917,9.18513147571458,16.4330967851451));
#85581=CARTESIAN_POINT('Ctrl Pts',(-1.99414804775193,9.15672358386778,16.4355366893506));
#85582=CARTESIAN_POINT('Ctrl Pts',(-2.13427143373024,9.12508035706661,16.4379765935562));
#85583=CARTESIAN_POINT('Ctrl Pts',(-2.27358039414982,9.09023746960648,16.4404164977618));
#85584=CARTESIAN_POINT('Ctrl Pts',(-2.50014914560209,9.03356983326021,16.4443846994328));
#85585=CARTESIAN_POINT('Ctrl Pts',(-2.72463341497766,8.96841854676107,16.4483529011038));
#85586=CARTESIAN_POINT('Ctrl Pts',(-2.94639355199476,8.89496206283443,16.4523211027748));
#85587=CARTESIAN_POINT('Ctrl Pts',(-3.1681148355162,8.82151844885465,16.4562886091968));
#85588=CARTESIAN_POINT('Ctrl Pts',(-3.38711266946891,8.73977263145653,16.4602561156189));
#85589=CARTESIAN_POINT('Ctrl Pts',(-3.6027633152631,8.64995269100904,16.4642236220409));
#85590=CARTESIAN_POINT('Ctrl Pts',(-3.81839044868502,8.5601425436223,16.468190695886));
#85591=CARTESIAN_POINT('Ctrl Pts',(-4.03067086008051,8.46226014019331,16.4721577697311));
#85592=CARTESIAN_POINT('Ctrl Pts',(-4.2390006054817,8.35658177302333,16.4761248435763));
#85593=CARTESIAN_POINT('Ctrl Pts',(-4.44734657320953,8.25089517683648,16.4800922263315));
#85594=CARTESIAN_POINT('Ctrl Pts',(-4.65174100518809,8.13741152999273,16.4840596090868));
#85595=CARTESIAN_POINT('Ctrl Pts',(-4.85160330036171,8.01645373456489,16.488026991842));
#85596=CARTESIAN_POINT('Ctrl Pts',(-5.0514634783335,7.89549722047962,16.4919943325696));
#85597=CARTESIAN_POINT('Ctrl Pts',(-5.24679137328432,7.76706686538866,16.4959616732972));
#85598=CARTESIAN_POINT('Ctrl Pts',(-5.43703361189728,7.6315300278253,16.4999290140247));
#85599=CARTESIAN_POINT('Ctrl Pts',(-5.62731680612774,7.49596401170036,16.503897208847));
#85600=CARTESIAN_POINT('Ctrl Pts',(-5.81251192428975,7.35328862087679,16.5078654036693));
#85601=CARTESIAN_POINT('Ctrl Pts',(-5.99209600092064,7.20391355988194,16.5118335984915));
#85602=CARTESIAN_POINT('Ctrl Pts',(-6.10251596750279,7.11206806025471,16.514273502674));
#85603=CARTESIAN_POINT('Ctrl Pts',(-6.21081524723272,7.01769050615019,16.5167134068564));
#85604=CARTESIAN_POINT('Ctrl Pts',(-6.3168786029285,6.92088359809382,16.5191533110388));
#85605=CARTESIAN_POINT('Ctrl Pts',(-6.48937750139262,6.76343916411478,16.5231215126959));
#85606=CARTESIAN_POINT('Ctrl Pts',(-6.65601394485932,6.59951792492163,16.5270897143529));
#85607=CARTESIAN_POINT('Ctrl Pts',(-6.81630970183415,6.42958063260596,16.53105791601));
#85608=CARTESIAN_POINT('Ctrl Pts',(-6.97657737418056,6.25967311416452,16.535025422418));
#85609=CARTESIAN_POINT('Ctrl Pts',(-7.13050638246639,6.0837518534588,16.538992928826));
#85610=CARTESIAN_POINT('Ctrl Pts',(-7.27765606150406,5.9023137253922,16.542960435234));
#85611=CARTESIAN_POINT('Ctrl Pts',(-7.42478969682335,5.720895379511,16.5469275090651));
#85612=CARTESIAN_POINT('Ctrl Pts',(-7.56514529956278,5.53396158811509,16.5508945828962));
#85613=CARTESIAN_POINT('Ctrl Pts',(-7.6983225160623,5.34204225939745,16.5548616567274));
#85614=CARTESIAN_POINT('Ctrl Pts',(-7.83151010287551,5.15010798620438,16.5588290394686));
#85615=CARTESIAN_POINT('Ctrl Pts',(-7.95751802192521,4.95318763203713,16.5627964222099));
#85616=CARTESIAN_POINT('Ctrl Pts',(-8.0759885932591,4.75184104364287,16.5667638049512));
#85617=CARTESIAN_POINT('Ctrl Pts',(-8.19445790960027,4.55049658817071,16.5707311456649));
#85618=CARTESIAN_POINT('Ctrl Pts',(-8.3053898955734,4.34472623859289,16.5746984863786));
#85619=CARTESIAN_POINT('Ctrl Pts',(-8.40847194162357,4.1351160406244,16.5786658270923));
#85620=CARTESIAN_POINT('Ctrl Pts',(-8.51157617932724,3.92546071746618,16.5826340219009));
#85621=CARTESIAN_POINT('Ctrl Pts',(-8.6068269743147,3.71196414930906,16.5866022167094));
#85622=CARTESIAN_POINT('Ctrl Pts',(-8.6939585842418,3.49523521354261,16.590570411518));
#85623=CARTESIAN_POINT('Ctrl Pts',(-8.74753276520119,3.36197616744439,16.5930103157839));
#85624=CARTESIAN_POINT('Ctrl Pts',(-8.79803834624232,3.22749552049675,16.5954502200498));
#85625=CARTESIAN_POINT('Ctrl Pts',(-8.84542266732393,3.0919383724279,16.5978901243158));
#85626=CARTESIAN_POINT('Ctrl Pts',(-8.922438993179,2.87160993362477,16.6018558340212));
#85627=CARTESIAN_POINT('Ctrl Pts',(-8.99123166558292,2.64836642609172,16.6058215437266));
#85628=CARTESIAN_POINT('Ctrl Pts',(-9.05159840689145,2.42283952065755,16.6097872534321));
#85629=CARTESIAN_POINT('Ctrl Pts',(-9.1119560688391,2.1973465352283,16.6137523666814));
#85630=CARTESIAN_POINT('Ctrl Pts',(-9.16389025429189,1.96957111243754,16.6177174799308));
#85631=CARTESIAN_POINT('Ctrl Pts',(-9.20724887214798,1.74015897803329,16.6216825931802));
#85632=CARTESIAN_POINT('Ctrl Pts',(-9.2506016704499,1.51077763511656,16.6256471742356));
#85633=CARTESIAN_POINT('Ctrl Pts',(-9.28538114690515,1.27976029945655,16.6296117552911));
#85634=CARTESIAN_POINT('Ctrl Pts',(-9.31148637694957,1.04776262310823,16.6335763363466));
#85635=CARTESIAN_POINT('Ctrl Pts',(-9.33759198184268,0.815761615472395,
16.63754097433));
#85636=CARTESIAN_POINT('Ctrl Pts',(-9.35502305804944,0.582780522227092,
16.6415056123135));
#85637=CARTESIAN_POINT('Ctrl Pts',(-9.36373045858973,0.349480988580246,
16.645470250297));
#85638=CARTESIAN_POINT('Ctrl Pts',(-9.36807896163217,0.232970472362477,
16.6474502028963));
#85639=CARTESIAN_POINT('Ctrl Pts',(-9.37025256073633,0.116380602494191,
16.6494301554957));
#85640=CARTESIAN_POINT('Ctrl Pts',(-9.37024999773577,-0.000205992430197824,
16.651410108095));
#85641=CARTESIAN_POINT('Ctrl Pts',(4.29092662815677,8.33003803918537,17.3256735943175));
#85642=CARTESIAN_POINT('Ctrl Pts',(4.29097821771431,8.33001146463611,17.3256726426547));
#85643=CARTESIAN_POINT('Ctrl Pts',(4.29102980690335,8.32998488935409,17.3256716911546));
#85644=CARTESIAN_POINT('Ctrl Pts',(4.55103047200112,8.19604856257909,17.3208754687787));
#85645=CARTESIAN_POINT('Ctrl Pts',(4.80456773014874,8.05004459447934,17.3161045805035));
#85646=CARTESIAN_POINT('Ctrl Pts',(5.09711683934695,7.86282397573055,17.310300584825));
#85647=CARTESIAN_POINT('Ctrl Pts',(5.14311149972626,7.83281590687947,17.3093787568522));
#85648=CARTESIAN_POINT('Ctrl Pts',(5.22431663423013,7.77881199345624,17.3077323279032));
#85649=CARTESIAN_POINT('Ctrl Pts',(5.25963223861385,7.75497704956278,17.3070097806095));
#85650=CARTESIAN_POINT('Ctrl Pts',(5.33872017865953,7.70081085156908,17.3053761130227));
#85651=CARTESIAN_POINT('Ctrl Pts',(5.38239884798838,7.67034572503948,17.3044632873311));
#85652=CARTESIAN_POINT('Ctrl Pts',(5.54292574620206,7.55633457580999,17.301072589534));
#85653=CARTESIAN_POINT('Ctrl Pts',(5.6581078311972,7.47047746970393,17.2985688759324));
#85654=CARTESIAN_POINT('Ctrl Pts',(6.04020614479632,7.17175211095036,17.2900737525178));
#85655=CARTESIAN_POINT('Ctrl Pts',(6.29745265428763,6.94695689234439,17.2840411098817));
#85656=CARTESIAN_POINT('Ctrl Pts',(6.63951357058691,6.61339924804405,17.2757321501428));
#85657=CARTESIAN_POINT('Ctrl Pts',(6.73507844538356,6.51605007359311,17.2733748032426));
#85658=CARTESIAN_POINT('Ctrl Pts',(6.88552669058092,6.35594572163212,17.269607123924));
#85659=CARTESIAN_POINT('Ctrl Pts',(6.94175720427595,6.29448415514974,17.268185488443));
#85660=CARTESIAN_POINT('Ctrl Pts',(7.05218246569183,6.17050654252348,17.2653659519672));
#85661=CARTESIAN_POINT('Ctrl Pts',(7.10638371389131,6.10800614519696,17.2639680783824));
#85662=CARTESIAN_POINT('Ctrl Pts',(7.24524107305612,5.94353674131959,17.2603481490724));
#85663=CARTESIAN_POINT('Ctrl Pts',(7.3285741974771,5.84047494373094,17.2581370587214));
#85664=CARTESIAN_POINT('Ctrl Pts',(7.51718633223192,5.59681454889321,17.2530272833262));
#85665=CARTESIAN_POINT('Ctrl Pts',(7.62075432577292,5.45495436401649,17.2501401062778));
#85666=CARTESIAN_POINT('Ctrl Pts',(7.89369928815981,5.05813630903082,17.2422406223595));
#85667=CARTESIAN_POINT('Ctrl Pts',(8.05466766021304,4.79766178725524,17.2372513318832));
#85668=CARTESIAN_POINT('Ctrl Pts',(8.22776116285262,4.48422122416561,17.2312609920759));
#85669=CARTESIAN_POINT('Ctrl Pts',(8.25254077159945,4.4384529442126,17.2303864332977));
#85670=CARTESIAN_POINT('Ctrl Pts',(8.29674693255514,4.35515339897856,17.2287929971384));
#85671=CARTESIAN_POINT('Ctrl Pts',(8.31630327395232,4.31769274533853,17.2280756817685));
#85672=CARTESIAN_POINT('Ctrl Pts',(8.36111570018489,4.23041940344972,17.2264023488769));
#85673=CARTESIAN_POINT('Ctrl Pts',(8.38618106739974,4.18051087384237,17.2254440747611));
#85674=CARTESIAN_POINT('Ctrl Pts',(8.48935096073708,3.97042344232227,17.221409115352));
#85675=CARTESIAN_POINT('Ctrl Pts',(8.56332389732108,3.80825755096658,17.2182924292607));
#85676=CARTESIAN_POINT('Ctrl Pts',(8.78425592282335,3.28488183961869,17.2083197981168));
#85677=CARTESIAN_POINT('Ctrl Pts',(8.91331857529786,2.91656577402384,17.2014450133711));
#85678=CARTESIAN_POINT('Ctrl Pts',(9.04504406615057,2.44906947532125,17.1930721413029));
#85679=CARTESIAN_POINT('Ctrl Pts',(9.06961110394666,2.35646301386921,17.1914292588907));
#85680=CARTESIAN_POINT('Ctrl Pts',(9.10990494028154,2.194597504292,17.1885848480121));
#85681=CARTESIAN_POINT('Ctrl Pts',(9.12627248775778,2.12550622923451,17.1873792455703));
#85682=CARTESIAN_POINT('Ctrl Pts',(9.16281199939242,1.96305458056824,17.1845637172916));
#85683=CARTESIAN_POINT('Ctrl Pts',(9.18234491090999,1.8695585082897,17.1829580670465));
#85684=CARTESIAN_POINT('Ctrl Pts',(9.24980199262434,1.52005848018524,17.1770051044867));
#85685=CARTESIAN_POINT('Ctrl Pts',(9.28847604180394,1.26238982578057,17.1727173771272));
#85686=CARTESIAN_POINT('Ctrl Pts',(9.34883473311864,0.701996810682248,17.1634732001829));
#85687=CARTESIAN_POINT('Ctrl Pts',(9.36665291698789,0.399151532677687,17.1585291761472));
#85688=CARTESIAN_POINT('Ctrl Pts',(9.37029669010384,0.043432259178177,17.152578941747));
#85689=CARTESIAN_POINT('Ctrl Pts',(9.37039290977881,-0.00911714825853897,
17.1516960927985));
#85690=CARTESIAN_POINT('Ctrl Pts',(9.36976869162356,-0.103968379140538,
17.150093607563));
#85691=CARTESIAN_POINT('Ctrl Pts',(9.36920380497295,-0.146269669516118,
17.1493756210499));
#85692=CARTESIAN_POINT('Ctrl Pts',(9.3672388513215,-0.243892738731495,17.1477104414955));
#85693=CARTESIAN_POINT('Ctrl Pts',(9.36563513975845,-0.299208582180905,
17.1467610990478));
#85694=CARTESIAN_POINT('Ctrl Pts',(9.35711484212669,-0.524254037369697,
17.1428794367222));
#85695=CARTESIAN_POINT('Ctrl Pts',(9.3460734591053,-0.693794700578072,17.1399107978014));
#85696=CARTESIAN_POINT('Ctrl Pts',(9.29300097226347,-1.26763373188855,17.129798698072));
#85697=CARTESIAN_POINT('Ctrl Pts',(9.22928214763292,-1.66946608927697,17.1226279385625));
#85698=CARTESIAN_POINT('Ctrl Pts',(9.11905861058671,-2.1571046249412,17.1140160470477));
#85699=CARTESIAN_POINT('Ctrl Pts',(9.0970764569506,-2.24800584913341,17.1124134811086));
#85700=CARTESIAN_POINT('Ctrl Pts',(9.05401323509711,-2.41509323408203,17.1094727773957));
#85701=CARTESIAN_POINT('Ctrl Pts',(9.03332172287519,-2.49137104329371,17.1081322349168));
#85702=CARTESIAN_POINT('Ctrl Pts',(8.98350471923446,-2.66623203914725,17.1050624741105));
#85703=CARTESIAN_POINT('Ctrl Pts',(8.95371701658031,-2.76461606426321,17.103337795225));
#85704=CARTESIAN_POINT('Ctrl Pts',(8.84740733806106,-3.09598090465691,17.0975303391178));
#85705=CARTESIAN_POINT('Ctrl Pts',(8.76336132044562,-3.32644152001317,17.0934961308356));
#85706=CARTESIAN_POINT('Ctrl Pts',(8.55898765480028,-3.82512611068331,17.0846580178484));
#85707=CARTESIAN_POINT('Ctrl Pts',(8.4348854419078,-4.09152363095245,17.0798659581457));
#85708=CARTESIAN_POINT('Ctrl Pts',(8.27317273202257,-4.3999053278032,17.0740462335787));
#85709=CARTESIAN_POINT('Ctrl Pts',(8.24744774601936,-4.44793880431639,17.0731314747842));
#85710=CARTESIAN_POINT('Ctrl Pts',(8.20089362376026,-4.53307166772422,17.0714931584655));
#85711=CARTESIAN_POINT('Ctrl Pts',(8.18022800721909,-4.57025871508599,17.0707715816735));
#85712=CARTESIAN_POINT('Ctrl Pts',(8.13295565134325,-4.65397574624297,17.0691329026291));
#85713=CARTESIAN_POINT('Ctrl Pts',(8.10620156262185,-4.70042062819725,17.0682140202201));
#85714=CARTESIAN_POINT('Ctrl Pts',(8.00438795634122,-4.87371340453068,17.0647522984064));
#85715=CARTESIAN_POINT('Ctrl Pts',(7.9267375773768,-4.99901391063899,17.0621822223329));
#85716=CARTESIAN_POINT('Ctrl Pts',(7.73945763839032,-5.28587563644333,17.0561799381729));
#85717=CARTESIAN_POINT('Ctrl Pts',(7.62766990621187,-5.44594689668563,17.0527404654126));
#85718=CARTESIAN_POINT('Ctrl Pts',(7.48937676635854,-5.63135191587965,17.0486805955986));
#85719=CARTESIAN_POINT('Ctrl Pts',(7.46762176250229,-5.66016907543471,17.0480472924013));
#85720=CARTESIAN_POINT('Ctrl Pts',(7.32256166434807,-5.85002681877477,17.0438604933698));
#85721=CARTESIAN_POINT('Ctrl Pts',(7.19422191126563,-6.00715362435688,17.0403280457051));
#85722=CARTESIAN_POINT('Ctrl Pts',(6.99963023851738,-6.23020412000172,17.0352297521916));
#85723=CARTESIAN_POINT('Ctrl Pts',(6.9373324142933,-6.29949885950972,17.0336331785939));
#85724=CARTESIAN_POINT('Ctrl Pts',(6.82028156666327,-6.42585366950758,17.0306979786604));
#85725=CARTESIAN_POINT('Ctrl Pts',(6.76581973634784,-6.48317201371972,17.0293570161597));
#85726=CARTESIAN_POINT('Ctrl Pts',(6.63855381292601,-6.61376261403732,17.026278612557));
#85727=CARTESIAN_POINT('Ctrl Pts',(6.56525050549346,-6.68653411803638,17.02454580959));
#85728=CARTESIAN_POINT('Ctrl Pts',(6.30733281678178,-6.93424971425095,17.0185787986013));
#85729=CARTESIAN_POINT('Ctrl Pts',(6.11680993016669,-7.10287991658575,17.0143976462547));
#85730=CARTESIAN_POINT('Ctrl Pts',(5.6998908030982,-7.44266153172543,17.0055794290911));
#85731=CARTESIAN_POINT('Ctrl Pts',(5.47210311943554,-7.61170493555478,17.0009502407934));
#85732=CARTESIAN_POINT('Ctrl Pts',(5.19187925310141,-7.80057280477059,16.9953021767148));
#85733=CARTESIAN_POINT('Ctrl Pts',(5.14649072274355,-7.83059253727644,16.994388579299));
#85734=CARTESIAN_POINT('Ctrl Pts',(5.06516458721259,-7.88336868523873,16.9927515899709));
#85735=CARTESIAN_POINT('Ctrl Pts',(5.02932867364814,-7.90627897403325,16.9920301667832));
#85736=CARTESIAN_POINT('Ctrl Pts',(4.94793455871087,-7.9575377917346,16.9903906365047));
#85737=CARTESIAN_POINT('Ctrl Pts',(4.90228648256506,-7.98574049975846,16.9894707367409));
#85738=CARTESIAN_POINT('Ctrl Pts',(4.72979449247776,-8.0902746872298,16.9859967598212));
#85739=CARTESIAN_POINT('Ctrl Pts',(4.6013900103263,-8.16398862205698,16.9834152011726));
#85740=CARTESIAN_POINT('Ctrl Pts',(4.3147640646925,-8.31962267731639,16.9777004811355));
#85741=CARTESIAN_POINT('Ctrl Pts',(4.15584300709399,-8.40013567278593,16.9745632525693));
#85742=CARTESIAN_POINT('Ctrl Pts',(3.77372685231633,-8.58022486177475,16.9671443789502));
#85743=CARTESIAN_POINT('Ctrl Pts',(3.54874009158387,-8.67569695014541,16.9628750328181));
#85744=CARTESIAN_POINT('Ctrl Pts',(3.22976906664956,-8.79656439964517,16.956993016288));
#85745=CARTESIAN_POINT('Ctrl Pts',(3.13873266361254,-8.8294569928234,16.9553327575967));
#85746=CARTESIAN_POINT('Ctrl Pts',(2.97262061413491,-8.88658157534683,16.9523366876462));
#85747=CARTESIAN_POINT('Ctrl Pts',(2.89771739835293,-8.91128718669281,16.9509978248047));
#85748=CARTESIAN_POINT('Ctrl Pts',(2.72837950968133,-8.96477971128716,16.9479971442045));
#85749=CARTESIAN_POINT('Ctrl Pts',(2.63378374427351,-8.99302581285969,16.9463390579085));
#85750=CARTESIAN_POINT('Ctrl Pts',(2.21933037904024,-9.10968034689929,16.9391455563678));
#85751=CARTESIAN_POINT('Ctrl Pts',(1.89535036876822,-9.18255688027763,16.9337147862008));
#85752=CARTESIAN_POINT('Ctrl Pts',(1.43833131696962,-9.26013698830243,16.926114906563));
#85753=CARTESIAN_POINT('Ctrl Pts',(1.30802335832507,-9.27944011414782,16.9239534697342));
#85754=CARTESIAN_POINT('Ctrl Pts',(1.0700269771862,-9.30958273908951,16.9199899821528));
#85755=CARTESIAN_POINT('Ctrl Pts',(0.962474731967153,-9.3213159368621,16.9181929602705));
#85756=CARTESIAN_POINT('Ctrl Pts',(0.803861869723648,-9.3358449991477,16.9155206818583));
#85757=CARTESIAN_POINT('Ctrl Pts',(0.752942768047164,-9.34008955665099,
16.9146594449482));
#85758=CARTESIAN_POINT('Ctrl Pts',(0.658952691285274,-9.34715086080005,
16.9130615829383));
#85759=CARTESIAN_POINT('Ctrl Pts',(0.615892158792157,-9.35008688138868,
16.9123262354685));
#85760=CARTESIAN_POINT('Ctrl Pts',(0.502162628556854,-9.35705231095244,
16.9103762954763));
#85761=CARTESIAN_POINT('Ctrl Pts',(0.431465648488899,-9.36057864739199,
16.9091563911607));
#85762=CARTESIAN_POINT('Ctrl Pts',(0.267477455635561,-9.36689654443972,
16.9063135991086));
#85763=CARTESIAN_POINT('Ctrl Pts',(0.174170907549871,-9.3690959813016,16.9046862966759));
#85764=CARTESIAN_POINT('Ctrl Pts',(-0.200775427095719,-9.37233116890465,
16.8981248857096));
#85765=CARTESIAN_POINT('Ctrl Pts',(-0.482364603050553,-9.36206318588132,
16.893151395504));
#85766=CARTESIAN_POINT('Ctrl Pts',(-0.944970258845761,-9.32426551511288,
16.885033961657));
#85767=CARTESIAN_POINT('Ctrl Pts',(-1.12640475273726,-9.30409097512259,
16.881862691635));
#85768=CARTESIAN_POINT('Ctrl Pts',(-1.39577434323878,-9.26614331836725,
16.8771836418002));
#85769=CARTESIAN_POINT('Ctrl Pts',(-1.48423081080008,-9.25238655497331,
16.8756516825369));
#85770=CARTESIAN_POINT('Ctrl Pts',(-1.65099896652092,-9.22399760919633,
16.8727718018418));
#85771=CARTESIAN_POINT('Ctrl Pts',(-1.72934770077451,-9.20963007107948,
16.8714223100646));
#85772=CARTESIAN_POINT('Ctrl Pts',(-1.91532078282375,-9.1730695582339,16.8682260960225));
#85773=CARTESIAN_POINT('Ctrl Pts',(-2.02275672949112,-9.1499789134594,16.8663853401387));
#85774=CARTESIAN_POINT('Ctrl Pts',(-2.25716806895841,-9.09526766875971,
16.8623755330154));
#85775=CARTESIAN_POINT('Ctrl Pts',(-2.38393767917349,-9.062866152648,16.8602113121964));
#85776=CARTESIAN_POINT('Ctrl Pts',(-2.85397349386821,-8.93218301487741,
16.8521754033214));
#85777=CARTESIAN_POINT('Ctrl Pts',(-3.19221074927094,-8.81696357961916,
16.8463806051515));
#85778=CARTESIAN_POINT('Ctrl Pts',(-3.59539403557866,-8.65337060819131,
16.8391462493862));
#85779=CARTESIAN_POINT('Ctrl Pts',(-3.66737286305208,-8.62311181598989,
16.8378410518825));
#85780=CARTESIAN_POINT('Ctrl Pts',(-3.77559264859349,-8.57601777422294,
16.8358525056425));
#85781=CARTESIAN_POINT('Ctrl Pts',(-3.81211802075441,-8.55984444381708,
16.8351767846005));
#85782=CARTESIAN_POINT('Ctrl Pts',(-3.89099827972331,-8.52431147259437,
16.8337064842666));
#85783=CARTESIAN_POINT('Ctrl Pts',(-3.93331450613576,-8.50486864555631,
16.8329108260949));
#85784=CARTESIAN_POINT('Ctrl Pts',(-4.05862720630252,-8.44615655348398,
16.8305359431349));
#85785=CARTESIAN_POINT('Ctrl Pts',(-4.14119324005963,-8.40598202507336,
16.8289467109252));
#85786=CARTESIAN_POINT('Ctrl Pts',(-4.46040163015587,-8.24481873040064,
16.822723960162));
#85787=CARTESIAN_POINT('Ctrl Pts',(-4.69244432369842,-8.11499752280547,
16.8180335125414));
#85788=CARTESIAN_POINT('Ctrl Pts',(-5.11923355461663,-7.8517875083662,16.8092306299026));
#85789=CARTESIAN_POINT('Ctrl Pts',(-5.31507562599017,-7.72056287171288,
16.805115527491));
#85790=CARTESIAN_POINT('Ctrl Pts',(-5.58335485243704,-7.52575104827351,
16.7993998525602));
#85791=CARTESIAN_POINT('Ctrl Pts',(-5.66007773063634,-7.46821935879904,
16.7977554267389));
#85792=CARTESIAN_POINT('Ctrl Pts',(-5.79204618653272,-7.36605911080785,
16.7949095095351));
#85793=CARTESIAN_POINT('Ctrl Pts',(-5.84769251055562,-7.32196136136638,
16.7937039271404));
#85794=CARTESIAN_POINT('Ctrl Pts',(-5.91590658827746,-7.26663042287683,
16.7922187216342));
#85795=CARTESIAN_POINT('Ctrl Pts',(-5.92895222260626,-7.2559902154205,16.7919343449152));
#85796=CARTESIAN_POINT('Ctrl Pts',(-5.95218554088438,-7.23693629417004,
16.7914272749044));
#85797=CARTESIAN_POINT('Ctrl Pts',(-5.96238423530891,-7.22853608067931,
16.7912044740943));
#85798=CARTESIAN_POINT('Ctrl Pts',(-5.98343058941076,-7.21112628423795,
16.790744246759));
#85799=CARTESIAN_POINT('Ctrl Pts',(-5.99427574802073,-7.2021137287882,16.7905068447255));
#85800=CARTESIAN_POINT('Ctrl Pts',(-6.01541970319076,-7.18446181415948,
16.790043507225));
#85801=CARTESIAN_POINT('Ctrl Pts',(-6.02572033476423,-7.17582470605425,
16.7898175546311));
#85802=CARTESIAN_POINT('Ctrl Pts',(-6.04688035580724,-7.15800428075745,
16.7893529095406));
#85803=CARTESIAN_POINT('Ctrl Pts',(-6.05773749657959,-7.14881834595813,
16.7891142383724));
#85804=CARTESIAN_POINT('Ctrl Pts',(-6.14037392405159,-7.07857845767196,
16.7872955984859));
#85805=CARTESIAN_POINT('Ctrl Pts',(-6.21124954062057,-7.0164694897886,16.7857240069436));
#85806=CARTESIAN_POINT('Ctrl Pts',(-6.40076432343102,-6.84527373599244,
16.7814837297196));
#85807=CARTESIAN_POINT('Ctrl Pts',(-6.51754560203392,-6.73417819148485,
16.7788296313941));
#85808=CARTESIAN_POINT('Ctrl Pts',(-6.80295871702365,-6.44827886962707,
16.7721977297799));
#85809=CARTESIAN_POINT('Ctrl Pts',(-6.96776867662509,-6.26982830417255,
16.7682346350307));
#85810=CARTESIAN_POINT('Ctrl Pts',(-7.19756409823333,-6.00074857568759,
16.7623874816041));
#85811=CARTESIAN_POINT('Ctrl Pts',(-7.26816125172843,-5.9150438985552,16.7605424983826));
#85812=CARTESIAN_POINT('Ctrl Pts',(-7.36799788332486,-5.78935584816625,
16.7578472238621));
#85813=CARTESIAN_POINT('Ctrl Pts',(-7.39846979736714,-5.7503633440447,16.7570124599158));
#85814=CARTESIAN_POINT('Ctrl Pts',(-7.44107685636038,-5.69494312784722,
16.7558266185048));
#85815=CARTESIAN_POINT('Ctrl Pts',(-7.45346938164514,-5.67871430752099,
16.7554794203767));
#85816=CARTESIAN_POINT('Ctrl Pts',(-7.49562042445197,-5.62313908894502,
16.7542907047262));
#85817=CARTESIAN_POINT('Ctrl Pts',(-7.52512117603729,-5.58359830514575,
16.7534454519072));
#85818=CARTESIAN_POINT('Ctrl Pts',(-7.58976103262434,-5.4955166515773,16.7515653023237));
#85819=CARTESIAN_POINT('Ctrl Pts',(-7.62474953930849,-5.44686792969848,
16.750528693163));
#85820=CARTESIAN_POINT('Ctrl Pts',(-7.72537132473201,-5.3040918188752,16.7474953048833));
#85821=CARTESIAN_POINT('Ctrl Pts',(-7.78974512303527,-5.20909041676758,
16.7454881327025));
#85822=CARTESIAN_POINT('Ctrl Pts',(-8.06892284822416,-4.78033371981941,
16.7365123809888));
#85823=CARTESIAN_POINT('Ctrl Pts',(-8.26413935400905,-4.43431058576743,
16.729507295104));
#85824=CARTESIAN_POINT('Ctrl Pts',(-8.47955789367914,-3.98852462923679,
16.7209659679655));
#85825=CARTESIAN_POINT('Ctrl Pts',(-8.52089692251835,-3.89942899530525,
16.7192806679644));
#85826=CARTESIAN_POINT('Ctrl Pts',(-8.5917745123903,-3.74015901009377,16.7163063871222));
#85827=CARTESIAN_POINT('Ctrl Pts',(-8.62187280820106,-3.67024358891125,
16.7150136412525));
#85828=CARTESIAN_POINT('Ctrl Pts',(-8.68604885631471,-3.51602159070716,
16.7121893293927));
#85829=CARTESIAN_POINT('Ctrl Pts',(-8.71975805295934,-3.43156991874006,
16.7106604031516));
#85830=CARTESIAN_POINT('Ctrl Pts',(-8.78934440374716,-3.24958566665368,
16.7074005401155));
#85831=CARTESIAN_POINT('Ctrl Pts',(-8.82483905176287,-3.15191970458903,
16.7056721783171));
#85832=CARTESIAN_POINT('Ctrl Pts',(-8.92300631952262,-2.86713754845002,
16.7006844083225));
#85833=CARTESIAN_POINT('Ctrl Pts',(-8.98140220320273,-2.67860675160458,
16.6974475151484));
#85834=CARTESIAN_POINT('Ctrl Pts',(-9.10203752618945,-2.24065166865257,
16.6900015982356));
#85835=CARTESIAN_POINT('Ctrl Pts',(-9.16005424429774,-1.99022921663034,
16.6857987266927));
#85836=CARTESIAN_POINT('Ctrl Pts',(-9.21929447170523,-1.67633513054968,
16.680464029308));
#85837=CARTESIAN_POINT('Ctrl Pts',(-9.230268799106,-1.61481512757205,16.6794151657529));
#85838=CARTESIAN_POINT('Ctrl Pts',(-9.24763336297542,-1.51150552066212,
16.6776451265327));
#85839=CARTESIAN_POINT('Ctrl Pts',(-9.25435764363617,-1.46977425305238,
16.6769276505856));
#85840=CARTESIAN_POINT('Ctrl Pts',(-9.26703970870357,-1.38752904068702,
16.6755083229828));
#85841=CARTESIAN_POINT('Ctrl Pts',(-9.2730147117165,-1.34701891219052,16.6748068519934));
#85842=CARTESIAN_POINT('Ctrl Pts',(-9.28669218998233,-1.24987971195934,
16.6731201305645));
#85843=CARTESIAN_POINT('Ctrl Pts',(-9.29414249731049,-1.19321680688366,
16.6721324524756));
#85844=CARTESIAN_POINT('Ctrl Pts',(-9.3471401732769,-0.759481734484727,
16.6645515043299));
#85845=CARTESIAN_POINT('Ctrl Pts',(-9.37024148570975,-0.380022225320088,
16.6578162803345));
#85846=CARTESIAN_POINT('Ctrl Pts',(-9.3702499976469,-0.000209995816083108,
16.6511809802189));
#85847=CARTESIAN_POINT('Origin',(0.,0.,0.));
#85848=CARTESIAN_POINT('',(-9.94199999699462,0.000244456475345012,4.321310091674));
#85849=CARTESIAN_POINT('',(-9.94181728593973,0.000151535147386895,4.17868990831418));
#85850=CARTESIAN_POINT('',(-9.942,-1.2175438477123E-15,0.));
#85851=CARTESIAN_POINT('',(4.30700280829072,8.96064120525846,4.00000358309546));
#85852=CARTESIAN_POINT('Ctrl Pts',(-9.94199999699462,0.000244456475334202,
4.321310091674));
#85853=CARTESIAN_POINT('Ctrl Pts',(-9.94199371857738,0.255586533386308,
4.31722274465953));
#85854=CARTESIAN_POINT('Ctrl Pts',(-9.9321461097209,0.510880897282077,4.31313539764506));
#85855=CARTESIAN_POINT('Ctrl Pts',(-9.9124941605588,0.765391087541386,4.30904805063059));
#85856=CARTESIAN_POINT('Ctrl Pts',(-9.89766379861191,0.957457442363556,
4.30596353035593));
#85857=CARTESIAN_POINT('Ctrl Pts',(-9.87725095393373,1.14907722439271,4.30287901008128));
#85858=CARTESIAN_POINT('Ctrl Pts',(-9.85129109814319,1.3399357072803,4.29979448980662));
#85859=CARTESIAN_POINT('Ctrl Pts',(-9.8183833284707,1.58187568743978,4.29588442637762));
#85860=CARTESIAN_POINT('Ctrl Pts',(-9.77655344436225,1.82263975150708,4.29197436294863));
#85861=CARTESIAN_POINT('Ctrl Pts',(-9.72590990526167,2.06156263905151,4.28806429951963));
#85862=CARTESIAN_POINT('Ctrl Pts',(-9.67527512730493,2.30044419382526,4.28415491251706));
#85863=CARTESIAN_POINT('Ctrl Pts',(-9.61582979615066,2.53748493387791,4.28024552551449));
#85864=CARTESIAN_POINT('Ctrl Pts',(-9.54773345703507,2.77202991207041,4.27633613851192));
#85865=CARTESIAN_POINT('Ctrl Pts',(-9.47964453321882,3.00654934966495,4.27242717721909));
#85866=CARTESIAN_POINT('Ctrl Pts',(-9.40290656051405,3.23857329900516,4.26851821592626));
#85867=CARTESIAN_POINT('Ctrl Pts',(-9.31772921026913,3.46746108328521,4.26460925463343));
#85868=CARTESIAN_POINT('Ctrl Pts',(-9.23254528386269,3.69636653896539,4.26069999154721));
#85869=CARTESIAN_POINT('Ctrl Pts',(-9.13892077283841,3.92213508202157,4.256790728461));
#85870=CARTESIAN_POINT('Ctrl Pts',(-9.03711430361115,4.14414394820773,4.25288146537478));
#85871=CARTESIAN_POINT('Ctrl Pts',(-8.935309270365,4.36614968295696,4.24897225742876));
#85872=CARTESIAN_POINT('Ctrl Pts',(-8.8253226284171,4.58439559298429,4.24506304948273));
#85873=CARTESIAN_POINT('Ctrl Pts',(-8.7074602835775,4.79828088068221,4.2411538415367));
#85874=CARTESIAN_POINT('Ctrl Pts',(-8.58957211277988,5.01221303485363,4.23724377700633));
#85875=CARTESIAN_POINT('Ctrl Pts',(-8.46380492523922,5.22178241140812,4.23333371247595));
#85876=CARTESIAN_POINT('Ctrl Pts',(-8.33051021589283,5.42641350644283,4.22942364794557));
#85877=CARTESIAN_POINT('Ctrl Pts',(-8.23544445933727,5.57235635713554,4.22663499080693));
#85878=CARTESIAN_POINT('Ctrl Pts',(-8.13655075276863,5.71578786046067,4.22384633366829));
#85879=CARTESIAN_POINT('Ctrl Pts',(-8.03397008202494,5.8565082362384,4.22105767652965));
#85880=CARTESIAN_POINT('Ctrl Pts',(-7.89015201606858,6.05379815585272,4.21714798015716));
#85881=CARTESIAN_POINT('Ctrl Pts',(-7.73904114242797,6.24581814187268,4.21323828378467));
#85882=CARTESIAN_POINT('Ctrl Pts',(-7.58104868104173,6.43203427351529,4.20932858741217));
#85883=CARTESIAN_POINT('Ctrl Pts',(-7.4230835710149,6.61821816776949,4.20541956787901));
#85884=CARTESIAN_POINT('Ctrl Pts',(-7.258239432691,6.79859999967778,4.20151054834584));
#85885=CARTESIAN_POINT('Ctrl Pts',(-7.08696755126958,6.97267917856917,4.19760152881267));
#85886=CARTESIAN_POINT('Ctrl Pts',(-6.91571429346933,7.1467394285818,4.19369293433525));
#85887=CARTESIAN_POINT('Ctrl Pts',(-6.73803488467048,7.31449819419016,4.18978433985784));
#85888=CARTESIAN_POINT('Ctrl Pts',(-6.55441795136341,7.47549124264386,4.18587574538043));
#85889=CARTESIAN_POINT('Ctrl Pts',(-6.37078667023574,7.63649687108861,4.18196684548558));
#85890=CARTESIAN_POINT('Ctrl Pts',(-6.18121714631811,7.79073553883579,4.17805794559074));
#85891=CARTESIAN_POINT('Ctrl Pts',(-5.98623258749013,7.93778202072035,4.17414904569589));
#85892=CARTESIAN_POINT('Ctrl Pts',(-5.7912506492937,8.08482652627072,4.17024019833744));
#85893=CARTESIAN_POINT('Ctrl Pts',(-5.59085404685443,8.22467887212325,4.16633135097899));
#85894=CARTESIAN_POINT('Ctrl Pts',(-5.38559716822796,8.35695561443131,4.16242250362055));
#85895=CARTESIAN_POINT('Ctrl Pts',(-5.18029496458159,8.48926156621589,4.15851279310669));
#85896=CARTESIAN_POINT('Ctrl Pts',(-4.97013057542729,8.61398841903633,4.15460308259284));
#85897=CARTESIAN_POINT('Ctrl Pts',(-4.75568650205221,8.7307966357142,4.15069337207899));
#85898=CARTESIAN_POINT('Ctrl Pts',(-4.602611665205,8.81417687760648,4.14790253580355));
#85899=CARTESIAN_POINT('Ctrl Pts',(-4.44735674001143,8.89352316422356,4.14511169952811));
#85900=CARTESIAN_POINT('Ctrl Pts',(-4.29014120223573,8.96872635689591,4.14232086325267));
#85901=CARTESIAN_POINT('Ctrl Pts',(-4.0698917999291,9.07408145393005,4.13841107144521));
#85902=CARTESIAN_POINT('Ctrl Pts',(-3.84572585590248,9.17133563349291,4.13450127963775));
#85903=CARTESIAN_POINT('Ctrl Pts',(-3.61825880447004,9.26021421047456,4.13059148783029));
#85904=CARTESIAN_POINT('Ctrl Pts',(-3.3908312192436,9.34907736676031,4.12668237438327));
#85905=CARTESIAN_POINT('Ctrl Pts',(-3.16010393093553,9.42956771938564,4.12277326093625));
#85906=CARTESIAN_POINT('Ctrl Pts',(-2.92671181169661,9.50145893909328,4.11886414748923));
#85907=CARTESIAN_POINT('Ctrl Pts',(-2.69334517628228,9.573342309079,4.11495546087393));
#85908=CARTESIAN_POINT('Ctrl Pts',(-2.45731455872118,9.63662833838923,4.11104677425864));
#85909=CARTESIAN_POINT('Ctrl Pts',(-2.2192704343439,9.69114042511236,4.10713808764335));
#85910=CARTESIAN_POINT('Ctrl Pts',(-1.98120791360177,9.74565672460167,4.10322909895958));
#85911=CARTESIAN_POINT('Ctrl Pts',(-1.74113184770521,9.79139766103141,4.09932011027581));
#85912=CARTESIAN_POINT('Ctrl Pts',(-1.49970462775759,9.82823738162049,4.09541112159205));
#85913=CARTESIAN_POINT('Ctrl Pts',(-1.25828077687107,9.86507658811979,4.09150218745731));
#85914=CARTESIAN_POINT('Ctrl Pts',(-1.01550608710088,9.89301478694713,4.08759325332258));
#85915=CARTESIAN_POINT('Ctrl Pts',(-0.77205055605658,9.91197770068581,4.08368431918785));
#85916=CARTESIAN_POINT('Ctrl Pts',(-0.528541500513394,9.93094478348341,
4.0797745256611));
#85917=CARTESIAN_POINT('Ctrl Pts',(-0.284351584124645,9.94093261553057,
4.07586473213434));
#85918=CARTESIAN_POINT('Ctrl Pts',(-0.0401547022073373,9.94191890933992,
4.07195493860759));
#85919=CARTESIAN_POINT('Ctrl Pts',(0.134120903294355,9.94262279609505,4.06916464239696));
#85920=CARTESIAN_POINT('Ctrl Pts',(0.308399974733068,9.93874308293179,4.06637434618633));
#85921=CARTESIAN_POINT('Ctrl Pts',(0.482437680168755,9.93028790543121,4.0635840499757));
#85922=CARTESIAN_POINT('Ctrl Pts',(0.725404420706052,9.91848398677555,4.05968863447517));
#85923=CARTESIAN_POINT('Ctrl Pts',(0.967980146918817,9.8977565807835,4.05579321897465));
#85924=CARTESIAN_POINT('Ctrl Pts',(1.20949750393456,9.86815483198232,4.05189780347412));
#85925=CARTESIAN_POINT('Ctrl Pts',(1.45096980006146,9.83855860610145,4.04800311475732));
#85926=CARTESIAN_POINT('Ctrl Pts',(1.69138383892895,9.80009137703121,4.04410842604052));
#85927=CARTESIAN_POINT('Ctrl Pts',(1.93007805039346,9.75285408069809,4.04021373732372));
#85928=CARTESIAN_POINT('Ctrl Pts',(2.16876458339275,9.70561830392397,4.03631917389371));
#85929=CARTESIAN_POINT('Ctrl Pts',(2.40573111986605,9.64961307557972,4.0324246104637));
#85930=CARTESIAN_POINT('Ctrl Pts',(2.64032578724286,9.58499054445128,4.02853004703369));
#85931=CARTESIAN_POINT('Ctrl Pts',(2.87490700908714,9.52037171709135,4.02463570681626));
#85932=CARTESIAN_POINT('Ctrl Pts',(3.1071163594724,9.44713665029117,4.02074136659882));
#85933=CARTESIAN_POINT('Ctrl Pts',(3.33631586752145,9.36548773060563,4.01684702638139));
#85934=CARTESIAN_POINT('Ctrl Pts',(3.56554539613377,9.28382811654042,4.01295217608307));
#85935=CARTESIAN_POINT('Ctrl Pts',(3.79176402657543,9.19375254278092,4.00905732578475));
#85936=CARTESIAN_POINT('Ctrl Pts',(4.01435139560835,9.09551245794195,4.00516247548644));
#85937=CARTESIAN_POINT('Ctrl Pts',(4.11262682739479,9.05213808859552,4.00344284468944));
#85938=CARTESIAN_POINT('Ctrl Pts',(4.21019465842555,9.0071728053732,4.00172321389245));
#85939=CARTESIAN_POINT('Ctrl Pts',(4.30700280829072,8.96064120525846,4.00000358309546));
#85940=CARTESIAN_POINT('',(-4.3070027565882,8.96064123010969,4.));
#85941=CARTESIAN_POINT('Origin',(0.,0.,4.));
#85942=CARTESIAN_POINT('Ctrl Pts',(-4.30700275658821,8.96064123010968,4.));
#85943=CARTESIAN_POINT('Ctrl Pts',(-5.78466622438202,8.25039065030607,4.02624560442566));
#85944=CARTESIAN_POINT('Ctrl Pts',(-8.38051839602705,6.0857098575996,4.07873681327696));
#85945=CARTESIAN_POINT('Ctrl Pts',(-9.80601533347217,2.52304867962029,4.13830011604837));
#85946=CARTESIAN_POINT('Ctrl Pts',(-9.94223863637244,0.441937600389724,
4.1716178143941));
#85947=CARTESIAN_POINT('Ctrl Pts',(-9.94181728593973,0.000151535147386895,
4.17868990831418));
#85948=CARTESIAN_POINT('Origin',(0.,0.,0.));
#85949=CARTESIAN_POINT('',(-9.94207409670986,-4.38639028224127E-5,5.32131009168581));
#85950=CARTESIAN_POINT('',(-9.94280319079831,-5.01184069386897E-5,5.17868990831418));
#85951=CARTESIAN_POINT('',(-9.942,-1.2175438477123E-15,0.));
#85952=CARTESIAN_POINT('Ctrl Pts',(-9.94199999990324,-4.38635759112934E-5,
5.32131009168581));
#85953=CARTESIAN_POINT('Ctrl Pts',(-9.94200107587134,0.243832168292933,
5.31740472848196));
#85954=CARTESIAN_POINT('Ctrl Pts',(-9.93302443488287,0.487747049262697,
5.3134993652781));
#85955=CARTESIAN_POINT('Ctrl Pts',(-9.91508755863515,0.731028525160635,
5.30959400207425));
#85956=CARTESIAN_POINT('Ctrl Pts',(-9.89715382840315,0.974267331011731,
5.30568932384664));
#85957=CARTESIAN_POINT('Ctrl Pts',(-9.8702630207256,1.21687267283672,5.30178464561903));
#85958=CARTESIAN_POINT('Ctrl Pts',(-9.83448462780497,1.45817560858349,5.29787996739142));
#85959=CARTESIAN_POINT('Ctrl Pts',(-9.79871008838425,1.69945255487779,5.29397570971588));
#85960=CARTESIAN_POINT('Ctrl Pts',(-9.75404991628052,1.93942709670595,5.29007145204033));
#85961=CARTESIAN_POINT('Ctrl Pts',(-9.70062519645207,2.17743766798482,5.28616719436479));
#85962=CARTESIAN_POINT('Ctrl Pts',(-9.64719641649626,2.4154663273929,5.28226263997673));
#85963=CARTESIAN_POINT('Ctrl Pts',(-9.58500181681745,2.65153044260325,5.27835808558866));
#85964=CARTESIAN_POINT('Ctrl Pts',(-9.51421339977782,2.88497961578381,5.27445353120059));
#85965=CARTESIAN_POINT('Ctrl Pts',(-9.44342531074129,3.11842770726125,5.27054899490455));
#85966=CARTESIAN_POINT('Ctrl Pts',(-9.3640435680187,3.349260612132,5.26664445860852));
#85967=CARTESIAN_POINT('Ctrl Pts',(-9.27628997551958,3.57684334156179,5.26273992231248));
#85968=CARTESIAN_POINT('Ctrl Pts',(-9.18851772000748,3.80447447219447,5.25883455561839));
#85969=CARTESIAN_POINT('Ctrl Pts',(-9.09237015821423,4.02885378329661,5.25492918892431));
#85970=CARTESIAN_POINT('Ctrl Pts',(-8.98811764605377,4.24936526797789,5.25102382223022));
#85971=CARTESIAN_POINT('Ctrl Pts',(-8.9312795738624,4.36958728877725,5.24889463119691));
#85972=CARTESIAN_POINT('Ctrl Pts',(-8.87203322919054,4.48866000202154,5.24676544016361));
#85973=CARTESIAN_POINT('Ctrl Pts',(-8.81042829879265,4.60648642588184,5.2446362491303));
#85974=CARTESIAN_POINT('Ctrl Pts',(-8.69730190640501,4.82285349541935,5.24072637213268));
#85975=CARTESIAN_POINT('Ctrl Pts',(-8.57618401983683,5.03508441183726,5.23681649513506));
#85976=CARTESIAN_POINT('Ctrl Pts',(-8.44740258010487,5.24259035684055,5.23290661813745));
#85977=CARTESIAN_POINT('Ctrl Pts',(-8.31864343361715,5.45006038066823,5.22899741797528));
#85978=CARTESIAN_POINT('Ctrl Pts',(-8.182223529961,5.65280682781202,5.2250882178131));
#85979=CARTESIAN_POINT('Ctrl Pts',(-8.03851535595362,5.85026793165047,5.22117901765093));
#85980=CARTESIAN_POINT('Ctrl Pts',(-7.89482282669338,6.04770753894523,5.21727024306266));
#85981=CARTESIAN_POINT('Ctrl Pts',(-7.74384377619892,6.23986272524124,5.21336146847438));
#85982=CARTESIAN_POINT('Ctrl Pts',(-7.58599299013171,6.42620217186423,5.20945269388611));
#85983=CARTESIAN_POINT('Ctrl Pts',(-7.42812995405602,6.61255607935789,5.20554361595743));
#85984=CARTESIAN_POINT('Ctrl Pts',(-7.26339429566316,6.7930931294541,5.20163453802875));
#85985=CARTESIAN_POINT('Ctrl Pts',(-7.0922407608604,6.96731547943613,5.19772546010007));
#85986=CARTESIAN_POINT('Ctrl Pts',(-6.92108958951511,7.14153542358344,5.19381643615181));
#85987=CARTESIAN_POINT('Ctrl Pts',(-6.74352091693189,7.3094406434833,5.18990741220355));
#85988=CARTESIAN_POINT('Ctrl Pts',(-6.56002649548621,7.47057001697454,5.18599838825529));
#85989=CARTESIAN_POINT('Ctrl Pts',(-6.37649171998725,7.63173482600257,5.18208850463533));
#85990=CARTESIAN_POINT('Ctrl Pts',(-6.18702880168393,7.7861206252772,5.17817862101537));
#85991=CARTESIAN_POINT('Ctrl Pts',(-5.99216377963559,7.93330556817418,5.17426873739541));
#85992=CARTESIAN_POINT('Ctrl Pts',(-5.8531243360058,8.03832448001357,5.17147897021472));
#85993=CARTESIAN_POINT('Ctrl Pts',(-5.71133536582068,8.13967821350184,5.16868920303402));
#85994=CARTESIAN_POINT('Ctrl Pts',(-5.56699758600683,8.23722658893114,5.16589943585332));
#85995=CARTESIAN_POINT('Ctrl Pts',(-5.3647072438242,8.37394127492951,5.16198955890828));
#85996=CARTESIAN_POINT('Ctrl Pts',(-5.157347343778,8.5032214925011,5.15807968196324));
#85997=CARTESIAN_POINT('Ctrl Pts',(-4.94548606880177,8.62470472209267,5.15416980501819));
#85998=CARTESIAN_POINT('Ctrl Pts',(-4.73366146894007,8.74616692183177,5.15026060490842));
#85999=CARTESIAN_POINT('Ctrl Pts',(-4.51733729271575,8.85983468858871,5.14635140479866));
#86000=CARTESIAN_POINT('Ctrl Pts',(-4.29710808425141,8.96539046066936,5.14244220468889));
#86001=CARTESIAN_POINT('Ctrl Pts',(-4.07690285095632,9.07093474146091,5.13853343015271));
#86002=CARTESIAN_POINT('Ctrl Pts',(-3.85279368692719,9.16836866975112,5.13462465561653));
#86003=CARTESIAN_POINT('Ctrl Pts',(-3.625397907429,9.25742156395664,5.13071588108035));
#86004=CARTESIAN_POINT('Ctrl Pts',(-3.39798448083671,9.3464813691295,5.12680680320296));
#86005=CARTESIAN_POINT('Ctrl Pts',(-3.16728418902501,9.4271587354904,5.12289772532556));
#86006=CARTESIAN_POINT('Ctrl Pts',(-2.93393362254536,9.49923141619878,5.11898864744816));
#86007=CARTESIAN_POINT('Ctrl Pts',(-2.70058627836868,9.57130310166632,5.11507962355064));
#86008=CARTESIAN_POINT('Ctrl Pts',(-2.46458900117124,9.6347702583646,5.11117059965312));
#86009=CARTESIAN_POINT('Ctrl Pts',(-2.22659351668162,9.68946052737052,5.10726157575559));
#86010=CARTESIAN_POINT('Ctrl Pts',(-1.98854569220281,9.7441628238655,5.10335169218516));
#86011=CARTESIAN_POINT('Ctrl Pts',(-1.74849905541982,9.79008431199061,5.09944180861474));
#86012=CARTESIAN_POINT('Ctrl Pts',(-1.50711686048621,9.82710347807726,5.09553192504431));
#86013=CARTESIAN_POINT('Ctrl Pts',(-1.33488661684927,9.85351727382592,5.09274215755499));
#86014=CARTESIAN_POINT('Ctrl Pts',(-1.16197667358011,9.87539990567294,5.08995239006567));
#86015=CARTESIAN_POINT('Ctrl Pts',(-0.988630237267956,9.89272329816009,
5.08716262257635));
#86016=CARTESIAN_POINT('Ctrl Pts',(-0.74568410805907,9.91700214253127,5.08325274575776));
#86017=CARTESIAN_POINT('Ctrl Pts',(-0.50180601029982,9.93233094993677,5.07934286893916));
#86018=CARTESIAN_POINT('Ctrl Pts',(-0.257668121537375,9.93866042981364,
5.07543299212057));
#86019=CARTESIAN_POINT('Ctrl Pts',(-0.0135724953327912,9.94498881399818,
5.07152379213831));
#86020=CARTESIAN_POINT('Ctrl Pts',(0.230782552021626,9.94232097324931,5.06761459215605));
#86021=CARTESIAN_POINT('Ctrl Pts',(0.474722987673566,9.93065970039122,5.0637053921738));
#86022=CARTESIAN_POINT('Ctrl Pts',(0.718636866802504,9.91899969703509,5.05979661776576));
#86023=CARTESIAN_POINT('Ctrl Pts',(0.962135944468283,9.89834822983191,5.05588784335772));
#86024=CARTESIAN_POINT('Ctrl Pts',(1.20454840477681,9.86876016227721,5.05197906894968));
#86025=CARTESIAN_POINT('Ctrl Pts',(1.44697967754732,9.83916979853527,5.04806999120051));
#86026=CARTESIAN_POINT('Ctrl Pts',(1.68832388582526,9.80064147956073,5.04416091345133));
#86027=CARTESIAN_POINT('Ctrl Pts',(1.92791524550065,9.75328184798154,5.04025183570216));
#86028=CARTESIAN_POINT('Ctrl Pts',(2.16750329670333,9.70592287038273,5.03634281193272));
#86029=CARTESIAN_POINT('Ctrl Pts',(2.40533827310429,9.64973288046047,5.03243378816328));
#86030=CARTESIAN_POINT('Ctrl Pts',(2.64076475604249,9.58486961326255,5.02852476439384));
#86031=CARTESIAN_POINT('Ctrl Pts',(2.8762430140654,9.51999208130941,5.02461488095035));
#86032=CARTESIAN_POINT('Ctrl Pts',(3.10931144962395,9.44643753422734,5.02070499750686));
#86033=CARTESIAN_POINT('Ctrl Pts',(3.33932863834611,9.36441392961255,5.01679511406338));
#86034=CARTESIAN_POINT('Ctrl Pts',(3.50344980983362,9.30588869437342,5.01400534580871));
#86035=CARTESIAN_POINT('Ctrl Pts',(3.66601786421949,9.24305285729568,5.01121557755405));
#86036=CARTESIAN_POINT('Ctrl Pts',(3.82680542478557,9.17599717964384,5.00842580929938));
#86037=CARTESIAN_POINT('Ctrl Pts',(4.05215018450145,9.08201823304599,5.00451593185117));
#86038=CARTESIAN_POINT('Ctrl Pts',(4.27406584119732,8.97971984947631,5.00060605440295));
#86039=CARTESIAN_POINT('Ctrl Pts',(4.49193740712761,8.86937778710816,4.99669617695474));
#86040=CARTESIAN_POINT('Ctrl Pts',(4.70977125761973,8.75905482589814,4.99278697633987));
#86041=CARTESIAN_POINT('Ctrl Pts',(4.92356216489259,8.64069109208017,4.988877775725));
#86042=CARTESIAN_POINT('Ctrl Pts',(5.13271823667751,8.51460906342024,4.98496857511014));
#86043=CARTESIAN_POINT('Ctrl Pts',(5.34185153879447,8.38854076061537,4.98105980006838));
#86044=CARTESIAN_POINT('Ctrl Pts',(5.54635077291072,8.25475598533229,4.97715102502662));
#86045=CARTESIAN_POINT('Ctrl Pts',(5.7456507202051,8.1136219902955,4.97324224998487));
#86046=CARTESIAN_POINT('Ctrl Pts',(5.94496613406024,7.97247704263408,4.96933317160481));
#86047=CARTESIAN_POINT('Ctrl Pts',(6.13908122430094,7.82398189508741,4.96542409322476));
#86048=CARTESIAN_POINT('Ctrl Pts',(6.32746066457328,7.6685465075383,4.9615150148447));
#86049=CARTESIAN_POINT('Ctrl Pts',(6.51583750342458,7.51311326647018,4.95760599044696));
#86050=CARTESIAN_POINT('Ctrl Pts',(6.69847863580534,7.35074015708262,4.95369696604923));
#86051=CARTESIAN_POINT('Ctrl Pts',(6.8748821158566,7.18187718448841,4.94978794165149));
#86052=CARTESIAN_POINT('Ctrl Pts',(7.05132439024468,7.01297707585224,4.94587805758812));
#86053=CARTESIAN_POINT('Ctrl Pts',(7.22152606800094,6.83758444533033,4.94196817352475));
#86054=CARTESIAN_POINT('Ctrl Pts',(7.38502136451266,6.6561868547759,4.93805828946138));
#86055=CARTESIAN_POINT('Ctrl Pts',(7.50167785954103,6.52675678814917,4.93526852498172));
#86056=CARTESIAN_POINT('Ctrl Pts',(7.61492085874833,6.39427035216825,4.93247876050206));
#86057=CARTESIAN_POINT('Ctrl Pts',(7.72459333987783,6.25891537996122,4.9296889960224));
#86058=CARTESIAN_POINT('Ctrl Pts',(7.87830014207589,6.06921437451954,4.9257791202483));
#86059=CARTESIAN_POINT('Ctrl Pts',(8.02503905688031,5.8738194963267,4.92186924447419));
#86060=CARTESIAN_POINT('Ctrl Pts',(8.16439975760317,5.67326542637037,4.91795936870009));
#86061=CARTESIAN_POINT('Ctrl Pts',(8.30373633355847,5.47274607438184,4.91405016976561));
#86062=CARTESIAN_POINT('Ctrl Pts',(8.4356970852241,5.26706954355613,4.91014097083112));
#86063=CARTESIAN_POINT('Ctrl Pts',(8.55991419398573,5.05680066757645,4.90623177189664));
#86064=CARTESIAN_POINT('Ctrl Pts',(8.68411777986816,4.8465546824903,4.90232299853659));
#86065=CARTESIAN_POINT('Ctrl Pts',(8.80057926354646,4.63171759173032,4.89841422517654));
#86066=CARTESIAN_POINT('Ctrl Pts',(8.90897556018459,4.4128809714328,4.89450545181648));
#86067=CARTESIAN_POINT('Ctrl Pts',(9.01738026913759,4.19402736787466,4.89059637510813));
#86068=CARTESIAN_POINT('Ctrl Pts',(9.11771841317532,3.97117386439473,4.88668729839978));
#86069=CARTESIAN_POINT('Ctrl Pts',(9.20971349255164,3.74493543136758,4.88277822169143));
#86070=CARTESIAN_POINT('Ctrl Pts',(9.30170730171872,3.51870012209607,4.87886919895711));
#86071=CARTESIAN_POINT('Ctrl Pts',(9.38535817293,3.28908023720895,4.87496017622279));
#86072=CARTESIAN_POINT('Ctrl Pts',(9.46043799751566,3.05671014248356,4.87105115348847));
#86073=CARTESIAN_POINT('Ctrl Pts',(9.53553433399791,2.8242889438698,4.86714127106408));
#86074=CARTESIAN_POINT('Ctrl Pts',(9.60205577016382,2.5891165933797,4.8632313886397));
#86075=CARTESIAN_POINT('Ctrl Pts',(9.65982385427233,2.35184334181326,4.85932150621531));
#86076=CARTESIAN_POINT('Ctrl Pts',(9.70104246646758,2.1825444237073,4.85653173172535));
#86077=CARTESIAN_POINT('Ctrl Pts',(9.73780570645368,2.01217625026479,4.85374195723539));
#86078=CARTESIAN_POINT('Ctrl Pts',(9.77006455811022,1.84097868818695,4.85095218274543));
#86079=CARTESIAN_POINT('Ctrl Pts',(9.81527545634597,1.6010446806247,4.84704230362422));
#86080=CARTESIAN_POINT('Ctrl Pts',(9.85165052663618,1.35940771688456,4.84313242450301));
#86081=CARTESIAN_POINT('Ctrl Pts',(9.87908249715191,1.11673318857586,4.83922254538179));
#86082=CARTESIAN_POINT('Ctrl Pts',(9.90650971898777,0.874100669048388,4.83531334308998));
#86083=CARTESIAN_POINT('Ctrl Pts',(9.92499689997156,0.630431221893893,4.83140414079818));
#86084=CARTESIAN_POINT('Ctrl Pts',(9.93448849574636,0.386396594036773,4.82749493850637));
#86085=CARTESIAN_POINT('Ctrl Pts',(9.94397905822149,0.14238853293462,4.82358616178867));
#86086=CARTESIAN_POINT('Ctrl Pts',(9.94447597994659,-0.101984349500512,
4.81967738507097));
#86087=CARTESIAN_POINT('Ctrl Pts',(9.93597578375624,-0.346048009110941,
4.81576860835327));
#86088=CARTESIAN_POINT('Ctrl Pts',(9.92747492794263,-0.590130608291953,
4.8118595283108));
#86089=CARTESIAN_POINT('Ctrl Pts',(9.90997556579693,-0.833903656436583,
4.80795044826834));
#86090=CARTESIAN_POINT('Ctrl Pts',(9.8835263270113,-1.07669463789624,4.80404136822587));
#86091=CARTESIAN_POINT('Ctrl Pts',(9.85707745354458,-1.31948226590828,4.80013234217592));
#86092=CARTESIAN_POINT('Ctrl Pts',(9.82167898307732,-1.56128757590726,4.79622331612596));
#86093=CARTESIAN_POINT('Ctrl Pts',(9.77743134303264,-1.80144395757484,4.79231429007601));
#86094=CARTESIAN_POINT('Ctrl Pts',(9.73317397244035,-2.04165315229877,4.7884044043878));
#86095=CARTESIAN_POINT('Ctrl Pts',(9.68006359359426,-2.28021241815636,4.78449451869959));
#86096=CARTESIAN_POINT('Ctrl Pts',(9.61825187905802,-2.51646474066237,4.78058463301138));
#86097=CARTESIAN_POINT('Ctrl Pts',(9.57414841327525,-2.68503385899083,4.77779487849707));
#86098=CARTESIAN_POINT('Ctrl Pts',(9.52561616142817,-2.85242871088613,4.77500512398277));
#86099=CARTESIAN_POINT('Ctrl Pts',(9.4727258673293,-3.01841492217858,4.77221536946846));
#86100=CARTESIAN_POINT('Ctrl Pts',(9.39859949374544,-3.25104656315668,4.7683054954763));
#86101=CARTESIAN_POINT('Ctrl Pts',(9.31588817074526,-3.48098188411319,4.76439562148414));
#86102=CARTESIAN_POINT('Ctrl Pts',(9.22481340416182,-3.70758434272189,4.76048574749199));
#86103=CARTESIAN_POINT('Ctrl Pts',(9.13375440358504,-3.93414757404505,4.75657655034043));
#86104=CARTESIAN_POINT('Ctrl Pts',(9.03433495404485,-4.15737883478786,4.75266735318887));
#86105=CARTESIAN_POINT('Ctrl Pts',(8.92682510426777,-4.37666054861634,4.74875815603731));
#86106=CARTESIAN_POINT('Ctrl Pts',(8.8193269584278,-4.59591839059128,4.74484938445603));
#86107=CARTESIAN_POINT('Ctrl Pts',(8.70374029427993,-4.81122729255618,4.74094061287476));
#86108=CARTESIAN_POINT('Ctrl Pts',(8.58038207571801,-5.02199237700508,4.73703184129349));
#86109=CARTESIAN_POINT('Ctrl Pts',(8.45701428308233,-5.23277381934636,4.73312276634477));
#86110=CARTESIAN_POINT('Ctrl Pts',(8.32587386974536,-5.43901049601501,4.72921369139605));
#86111=CARTESIAN_POINT('Ctrl Pts',(8.18732293327937,-5.64013361421498,4.72530461644733));
#86112=CARTESIAN_POINT('Ctrl Pts',(8.04877390936083,-5.84125395612547,4.72139559545921));
#86113=CARTESIAN_POINT('Ctrl Pts',(7.90281472763088,-6.03726065105612,4.7174865744711));
#86114=CARTESIAN_POINT('Ctrl Pts',(7.74985026922005,-6.2276146962276,4.71357755348298));
#86115=CARTESIAN_POINT('Ctrl Pts',(7.59685216885469,-6.41801060656304,4.70966767277158));
#86116=CARTESIAN_POINT('Ctrl Pts',(7.43684588811653,-6.60275116378262,4.70575779206017));
#86117=CARTESIAN_POINT('Ctrl Pts',(7.27027685317035,-6.7813301407803,4.70184791134877));
#86118=CARTESIAN_POINT('Ctrl Pts',(7.15142621853708,-6.90875013066734,4.69905812629634));
#86119=CARTESIAN_POINT('Ctrl Pts',(7.02923524624691,-7.03303386317473,4.69626834124391));
#86120=CARTESIAN_POINT('Ctrl Pts',(6.90387748118228,-7.15400864724276,4.69347855619148));
#86121=CARTESIAN_POINT('Ctrl Pts',(6.72818879098361,-7.3235545971807,4.68956867728175));
#86122=CARTESIAN_POINT('Ctrl Pts',(6.5462246180508,-7.48665149996543,4.68565879837202));
#86123=CARTESIAN_POINT('Ctrl Pts',(6.35848213136219,-7.6428442994181,4.68174891946229));
#86124=CARTESIAN_POINT('Ctrl Pts',(6.17077214485523,-7.79901006026889,4.67783971739336));
#86125=CARTESIAN_POINT('Ctrl Pts',(5.97728605677042,-7.94827392443534,4.67393051532443));
#86126=CARTESIAN_POINT('Ctrl Pts',(5.77855475406128,-8.09022057513364,4.67002131325549));
#86127=CARTESIAN_POINT('Ctrl Pts',(5.57984508671291,-8.23215177246876,4.66611253677124));
#86128=CARTESIAN_POINT('Ctrl Pts',(5.37589157292128,-8.36676718403924,4.66220376028698));
#86129=CARTESIAN_POINT('Ctrl Pts',(5.16725561277052,-8.49369374490814,4.65829498380273));
#86130=CARTESIAN_POINT('Ctrl Pts',(4.958603463037,-8.62063015493275,4.65438590400805));
#86131=CARTESIAN_POINT('Ctrl Pts',(4.74526837880589,-8.73987637374855,4.65047682421338));
#86132=CARTESIAN_POINT('Ctrl Pts',(4.52783909783716,-8.8511037223669,4.64656774441871));
#86133=CARTESIAN_POINT('Ctrl Pts',(4.31041282044257,-8.96232953448755,4.64265871862417));
#86134=CARTESIAN_POINT('Ctrl Pts',(4.08889270993251,-9.06553657212145,4.63874969282963));
#86135=CARTESIAN_POINT('Ctrl Pts',(3.86389101420379,-9.16044268746632,4.63484066703509));
#86136=CARTESIAN_POINT('Ctrl Pts',(3.63883983869041,-9.25536967347235,4.63093078161257));
#86137=CARTESIAN_POINT('Ctrl Pts',(3.41030580608748,-9.34199197973344,4.62702089619005));
#86138=CARTESIAN_POINT('Ctrl Pts',(3.17892128675169,-9.42007555450788,4.62311101076753));
#86139=CARTESIAN_POINT('Ctrl Pts',(3.01382531333293,-9.4757892376117,4.62032125481652));
#86140=CARTESIAN_POINT('Ctrl Pts',(2.84727857387036,-9.52715684556414,4.61753149886552));
#86141=CARTESIAN_POINT('Ctrl Pts',(2.67951578883477,-9.57410879076404,4.61474174291451));
#86142=CARTESIAN_POINT('Ctrl Pts',(2.4443939330779,-9.63991258917172,4.61083186149373));
#86143=CARTESIAN_POINT('Ctrl Pts',(2.20681090843899,-9.6970610561153,4.60692198007295));
#86144=CARTESIAN_POINT('Ctrl Pts',(1.96742032879298,-9.74538974335312,4.60301209865217));
#86145=CARTESIAN_POINT('Ctrl Pts',(1.72807118751074,-9.79371006492456,4.59910289402949));
#86146=CARTESIAN_POINT('Ctrl Pts',(1.48691539044466,-9.8332135989825,4.59519368940681));
#86147=CARTESIAN_POINT('Ctrl Pts',(1.24461735909541,-9.86378688077953,4.59128448478413));
#86148=CARTESIAN_POINT('Ctrl Pts',(1.00234570392804,-9.89435683441728,4.5873757057113));
#86149=CARTESIAN_POINT('Ctrl Pts',(0.758932340745822,-9.9159984417523,4.58346692663847));
#86150=CARTESIAN_POINT('Ctrl Pts',(0.515048485219441,-9.9286499111346,4.57955814756564));
#86151=CARTESIAN_POINT('Ctrl Pts',(0.27114570285142,-9.94130236234638,4.57564906514825));
#86152=CARTESIAN_POINT('Ctrl Pts',(0.0267726349693093,-9.94496326390372,
4.57173998273085));
#86153=CARTESIAN_POINT('Ctrl Pts',(-0.217396516537479,-9.93962286782539,
4.56783090031346));
#86154=CARTESIAN_POINT('Ctrl Pts',(-0.461562296017011,-9.93428254549904,
4.56392187188131));
#86155=CARTESIAN_POINT('Ctrl Pts',(-0.705523884537556,-9.91994118234583,
4.56001284344917));
#86156=CARTESIAN_POINT('Ctrl Pts',(-0.948608481140175,-9.89664114482833,
4.55610381501702));
#86157=CARTESIAN_POINT('Ctrl Pts',(-1.19174653440938,-9.873335983406,4.55219392695151));
#86158=CARTESIAN_POINT('Ctrl Pts',(-1.43400693115669,-9.84106823678216,
4.548284038886));
#86159=CARTESIAN_POINT('Ctrl Pts',(-1.6747219958265,-9.79993215469857,4.54437415082049));
#86160=CARTESIAN_POINT('Ctrl Pts',(-1.84647436524944,-9.77058118916459,
4.54158441042617));
#86161=CARTESIAN_POINT('Ctrl Pts',(-2.01744012065032,-9.73671648235652,
4.53879467003186));
#86162=CARTESIAN_POINT('Ctrl Pts',(-2.18737964906489,-9.6983882305699,4.53600492963754));
#86163=CARTESIAN_POINT('Ctrl Pts',(-2.42555191910766,-9.64467072988035,
4.53209507529851));
#86164=CARTESIAN_POINT('Ctrl Pts',(-2.66178090260783,-9.58216724556021,
4.52818522095948));
#86165=CARTESIAN_POINT('Ctrl Pts',(-2.89541328308477,-9.51104336653641,
4.52427536662045));
#86166=CARTESIAN_POINT('Ctrl Pts',(-3.12900521299153,-9.43993180173658,
4.52036618922456));
#86167=CARTESIAN_POINT('Ctrl Pts',(-3.36000116928354,-9.36020290322677,
4.51645701182867));
#86168=CARTESIAN_POINT('Ctrl Pts',(-3.587762529562,-9.27207226198496,4.51254783443278));
#86169=CARTESIAN_POINT('Ctrl Pts',(-3.81549909215251,-9.18395121603244,
4.5086390826515));
#86170=CARTESIAN_POINT('Ctrl Pts',(-4.04000150056862,-9.08743035491912,
4.50473033087022));
#86171=CARTESIAN_POINT('Ctrl Pts',(-4.26064968623793,-8.98277397306425,
4.50082157908893));
#86172=CARTESIAN_POINT('Ctrl Pts',(-4.48131500117173,-8.87810946657044,
4.49691252386512));
#86173=CARTESIAN_POINT('Ctrl Pts',(-4.69812524087963,-8.76530829469485,
4.49300346864131));
#86174=CARTESIAN_POINT('Ctrl Pts',(-4.91048241798382,-8.64468197348357,
4.48909441341749));
#86175=CARTESIAN_POINT('Ctrl Pts',(-5.12283666769756,-8.52405731513269,
4.48518541208087));
#86176=CARTESIAN_POINT('Ctrl Pts',(-5.3307377348432,-8.39560786344257,4.48127641074424));
#86177=CARTESIAN_POINT('Ctrl Pts',(-5.53361360808909,-8.25969033538009,
4.47736740940762));
#86178=CARTESIAN_POINT('Ctrl Pts',(-5.73653411367527,-8.12374290569714,
4.47345754809748));
#86179=CARTESIAN_POINT('Ctrl Pts',(-5.93442698278003,-7.98032427197115,
4.46954768678734));
#86180=CARTESIAN_POINT('Ctrl Pts',(-6.12674934828163,-7.82983438032571,
4.4656378254772));
#86181=CARTESIAN_POINT('Ctrl Pts',(-6.26398202980047,-7.72245149057122,
4.46284792243832));
#86182=CARTESIAN_POINT('Ctrl Pts',(-6.3983790349284,-7.61146909301393,4.46005801939944));
#86183=CARTESIAN_POINT('Ctrl Pts',(-6.52975327862434,-7.49704515928074,
4.45726811636056));
#86184=CARTESIAN_POINT('Ctrl Pts',(-6.71386901944704,-7.33668459898784,
4.45335817899099));
#86185=CARTESIAN_POINT('Ctrl Pts',(-6.89210275204051,-7.16951384949421,
4.44944824162141));
#86186=CARTESIAN_POINT('Ctrl Pts',(-7.06395809425259,-6.99598885381068,
4.44553830425183));
#86187=CARTESIAN_POINT('Ctrl Pts',(-7.23578369717028,-6.82249388635242,
4.44162904349071));
#86188=CARTESIAN_POINT('Ctrl Pts',(-7.40123291594315,-6.64264706679494,
4.4377197827296));
#86189=CARTESIAN_POINT('Ctrl Pts',(-7.55984604129784,-6.45694136816135,
4.43381052196848));
#86190=CARTESIAN_POINT('Ctrl Pts',(-7.71844190155171,-6.27125588366579,
4.42990168673193));
#86191=CARTESIAN_POINT('Ctrl Pts',(-7.8702029721684,-6.07971300651,4.42599285149538));
#86192=CARTESIAN_POINT('Ctrl Pts',(-8.0147089969722,-5.88283976442099,4.42208401625883));
#86193=CARTESIAN_POINT('Ctrl Pts',(-8.15922622264439,-5.68595126240579,
4.41817487804287));
#86194=CARTESIAN_POINT('Ctrl Pts',(-8.29648711048636,-5.48373179403123,
4.41426573982692));
#86195=CARTESIAN_POINT('Ctrl Pts',(-8.42611325824664,-5.27673946288807,
4.41035660161097));
#86196=CARTESIAN_POINT('Ctrl Pts',(-8.55573760615249,-5.06975000582602,
4.40644751767326));
#86197=CARTESIAN_POINT('Ctrl Pts',(-8.67772727895973,-4.85798805720064,
4.40253843373555));
#86198=CARTESIAN_POINT('Ctrl Pts',(-8.79174819658104,-4.64203916914905,
4.39862934979784));
#86199=CARTESIAN_POINT('Ctrl Pts',(-8.90579416360266,-4.42604283901178,
4.39471940706851));
#86200=CARTESIAN_POINT('Ctrl Pts',(-9.01186774549705,-4.2058579789586,4.39080946433918));
#86201=CARTESIAN_POINT('Ctrl Pts',(-9.10968103650867,-3.98209435009699,
4.38689952160985));
#86202=CARTESIAN_POINT('Ctrl Pts',(-9.17946236500216,-3.82245834226004,
4.38411011543443));
#86203=CARTESIAN_POINT('Ctrl Pts',(-9.24504051037593,-3.6610013945544,4.38132070925901));
#86204=CARTESIAN_POINT('Ctrl Pts',(-9.30632586764886,-3.49795123538475,
4.37853130308359));
#86205=CARTESIAN_POINT('Ctrl Pts',(-9.39202256166296,-3.26995452913916,
4.374630813666));
#86206=CARTESIAN_POINT('Ctrl Pts',(-9.46935111084644,-3.03876848928669,
4.37073032424842));
#86207=CARTESIAN_POINT('Ctrl Pts',(-9.53809144555643,-2.80502684054953,
4.36682983483083));
#86208=CARTESIAN_POINT('Ctrl Pts',(-9.60682298126833,-2.57131511154334,
4.36292984468924));
#86209=CARTESIAN_POINT('Ctrl Pts',(-9.66696841488264,-2.33504869741452,
4.35902985454765));
#86210=CARTESIAN_POINT('Ctrl Pts',(-9.7183574872742,-2.09687666531474,4.35512986440605));
#86211=CARTESIAN_POINT('Ctrl Pts',(-9.76973981138758,-1.85873590934144,
4.35123038640094));
#86212=CARTESIAN_POINT('Ctrl Pts',(-9.81236801113123,-1.61869031178751,
4.34733090839582));
#86213=CARTESIAN_POINT('Ctrl Pts',(-9.84612272724908,-1.37740017422287,
4.3434314303907));
#86214=CARTESIAN_POINT('Ctrl Pts',(-9.8798799731463,-1.13609195293888,4.33953166013549));
#86215=CARTESIAN_POINT('Ctrl Pts',(-9.90476236463304,-0.893539285235661,
4.33563188988028));
#86216=CARTESIAN_POINT('Ctrl Pts',(-9.9207021378468,-0.650409941592197,
4.33173211962506));
#86217=CARTESIAN_POINT('Ctrl Pts',(-9.93490167191397,-0.433824463775272,
4.32825811031198));
#86218=CARTESIAN_POINT('Ctrl Pts',(-9.94200533327122,-0.216781588312717,
4.32478410099889));
#86219=CARTESIAN_POINT('Ctrl Pts',(-9.94199999699464,0.000244455737705986,
4.32131009168581));
#86220=CARTESIAN_POINT('Ctrl Pts',(-9.94181728593973,0.000151535147386895,
4.17868990831418));
#86221=CARTESIAN_POINT('Ctrl Pts',(-9.94067494153095,-1.19759694767415,
4.19786341881976));
#86222=CARTESIAN_POINT('Ctrl Pts',(-9.42716810349573,-4.0356543903417,4.24328253375099));
#86223=CARTESIAN_POINT('Ctrl Pts',(-6.78745657491302,-7.82265052093215,
4.3149472531079));
#86224=CARTESIAN_POINT('Ctrl Pts',(-2.25961972835393,-10.1071926315035,
4.39368406638486));
#86225=CARTESIAN_POINT('Ctrl Pts',(2.81004432863975,-9.9682562140793,4.47242087966184));
#86226=CARTESIAN_POINT('Ctrl Pts',(7.2058836988398,-7.4388954948298,4.55115769293881));
#86227=CARTESIAN_POINT('Ctrl Pts',(9.87378550027097,-3.1257728072169,4.62989450621579));
#86228=CARTESIAN_POINT('Ctrl Pts',(10.1740080784303,1.9369173557757,4.70863131949275));
#86229=CARTESIAN_POINT('Ctrl Pts',(8.03455597735996,6.5351327702113,4.78736813276973));
#86230=CARTESIAN_POINT('Ctrl Pts',(3.96846040700314,9.5662641254359,4.86610494604671));
#86231=CARTESIAN_POINT('Ctrl Pts',(-1.04925135204577,10.3034526025732,4.94484175932367));
#86232=CARTESIAN_POINT('Ctrl Pts',(-5.81535800483383,8.56992920228316,5.02357857260066));
#86233=CARTESIAN_POINT('Ctrl Pts',(-9.15325378605286,4.81926962775394,5.10152795559748));
#86234=CARTESIAN_POINT('Ctrl Pts',(-9.94235238109963,1.58985384631345,5.15323173416867));
#86235=CARTESIAN_POINT('Ctrl Pts',(-9.94280319079831,-5.01184069386897E-5,
5.17868990831418));
#86236=CARTESIAN_POINT('Origin',(0.,0.,0.));
#86237=CARTESIAN_POINT('',(-9.94155665446311,-0.000214602085816251,6.32131009168581));
#86238=CARTESIAN_POINT('',(-9.94154134406803,-0.000211681655451256,6.17868990831418));
#86239=CARTESIAN_POINT('',(-9.942,-1.2175438477123E-15,0.));
#86240=CARTESIAN_POINT('Ctrl Pts',(-9.94155665446311,-0.000214602085816251,
6.32131009168581));
#86241=CARTESIAN_POINT('Ctrl Pts',(-9.94066724770169,1.10548046214137,6.30361166836752));
#86242=CARTESIAN_POINT('Ctrl Pts',(-9.48359125834515,3.85156620137575,6.25966764062359));
#86243=CARTESIAN_POINT('Ctrl Pts',(-7.00230141619256,7.63084835322035,6.18947800845398));
#86244=CARTESIAN_POINT('Ctrl Pts',(-2.53974329043462,10.0405067467589,6.110741195177));
#86245=CARTESIAN_POINT('Ctrl Pts',(2.53183186998833,10.0425046226134,6.03200438190005));
#86246=CARTESIAN_POINT('Ctrl Pts',(6.99628711260754,7.63636290068329,5.95326756862306));
#86247=CARTESIAN_POINT('Ctrl Pts',(9.7830696364778,3.39906166477283,5.87453075534608));
#86248=CARTESIAN_POINT('Ctrl Pts',(10.2239237027893,-1.65331661598174,5.79579394206911));
#86249=CARTESIAN_POINT('Ctrl Pts',(8.21313483354066,-6.30923829939991,5.71705712879214));
#86250=CARTESIAN_POINT('Ctrl Pts',(4.23287958537107,-9.45223794295327,5.63832031551517));
#86251=CARTESIAN_POINT('Ctrl Pts',(-0.762397843559365,-10.3286408224073,
5.55958350223819));
#86252=CARTESIAN_POINT('Ctrl Pts',(-5.57485629398454,-8.72829015437749,
5.48084668896123));
#86253=CARTESIAN_POINT('Ctrl Pts',(-9.05049363283098,-5.03494157965019,
5.40210987568424));
#86254=CARTESIAN_POINT('Ctrl Pts',(-9.93214544881101,-1.72500676017719,
5.34893100992577));
#86255=CARTESIAN_POINT('Ctrl Pts',(-9.9428190193766,-0.0429890845476765,
5.32199774859297));
#86256=CARTESIAN_POINT('Ctrl Pts',(-9.9428082600987,-4.38671419117354E-5,
5.32131009168581));
#86257=CARTESIAN_POINT('Ctrl Pts',(-9.94280319079831,-5.01184069386897E-5,
5.17868990831418));
#86258=CARTESIAN_POINT('Ctrl Pts',(-9.94281713450084,-0.0492264072162153,
5.17947733859432));
#86259=CARTESIAN_POINT('Ctrl Pts',(-9.93054952213869,-1.73747597041708,
5.20651037330044));
#86260=CARTESIAN_POINT('Ctrl Pts',(-9.04100851487771,-5.05195381719555,
5.25978901243127));
#86261=CARTESIAN_POINT('Ctrl Pts',(-5.55843129702091,-8.73875925129238,
5.3385258257087));
#86262=CARTESIAN_POINT('Ctrl Pts',(-0.742971601277903,-10.3300564063074,
5.41726263898546));
#86263=CARTESIAN_POINT('Ctrl Pts',(4.25064876577104,-9.44426053244652,5.49599945226253));
#86264=CARTESIAN_POINT('Ctrl Pts',(8.2249859947697,-6.29378085182736,5.57473626553945));
#86265=CARTESIAN_POINT('Ctrl Pts',(10.2270149997805,-1.63408573721985,5.65347307881644));
#86266=CARTESIAN_POINT('Ctrl Pts',(9.77665979209908,3.41745450715161,5.7322098920934));
#86267=CARTESIAN_POINT('Ctrl Pts',(6.9819131739284,7.64950720241167,5.81094670537039));
#86268=CARTESIAN_POINT('Ctrl Pts',(2.51294063151338,10.0472484483636,5.88968351864737));
#86269=CARTESIAN_POINT('Ctrl Pts',(-2.55862180937833,10.035712552753,5.96842033192432));
#86270=CARTESIAN_POINT('Ctrl Pts',(-7.01664024644669,7.61766576156723,6.04715714520133));
#86271=CARTESIAN_POINT('Ctrl Pts',(-9.48730107152748,3.83910257889644,6.11724700399791));
#86272=CARTESIAN_POINT('Ctrl Pts',(-9.94067098893944,1.09925498394695,6.16109125836888));
#86273=CARTESIAN_POINT('Ctrl Pts',(-9.94154134406803,-0.000211681655451256,
6.17868990831418));
#86274=CARTESIAN_POINT('Origin',(0.,0.,0.));
#86275=CARTESIAN_POINT('',(-9.94199999856713,0.00016879341615152,7.32131009168581));
#86276=CARTESIAN_POINT('',(-9.94199999849644,0.000172907010996282,7.17868990831418));
#86277=CARTESIAN_POINT('',(-9.942,-1.2175438477123E-15,0.));
#86278=CARTESIAN_POINT('Ctrl Pts',(-9.94137899628422,0.000169123441638015,
7.32131008623474));
#86279=CARTESIAN_POINT('Ctrl Pts',(-9.94175804919024,0.614877989386383,
7.3114711889337));
#86280=CARTESIAN_POINT('Ctrl Pts',(-9.73589259794127,2.86909352714112,7.27538668720702));
#86281=CARTESIAN_POINT('Ctrl Pts',(-8.05196685992069,6.5136703477983,7.21305658105461));
#86282=CARTESIAN_POINT('Ctrl Pts',(-3.99397426891797,9.55563923828576,7.13431976777767));
#86283=CARTESIAN_POINT('Ctrl Pts',(1.02175226903423,10.3062162801764,7.05558295450068));
#86284=CARTESIAN_POINT('Ctrl Pts',(5.7924680063296,8.58541706084741,6.97684614122372));
#86285=CARTESIAN_POINT('Ctrl Pts',(9.17418049203979,4.8058801496214,6.89810932794675));
#86286=CARTESIAN_POINT('Ctrl Pts',(10.3559729229203,-0.126081452991023,
6.81937251466976));
#86287=CARTESIAN_POINT('Ctrl Pts',(9.05445771229864,-5.02780938871426,6.74063570139281));
#86288=CARTESIAN_POINT('Ctrl Pts',(5.58173133745689,-8.72389517300014,6.66189888811582));
#86289=CARTESIAN_POINT('Ctrl Pts',(0.770535251822135,-10.3280369450708,
6.58316207483886));
#86290=CARTESIAN_POINT('Ctrl Pts',(-4.22543111982425,-9.45556997566333,
6.50442526156187));
#86291=CARTESIAN_POINT('Ctrl Pts',(-8.20816141345054,-6.31570723860668,
6.42568844828491));
#86292=CARTESIAN_POINT('Ctrl Pts',(-9.7698093539024,-2.70757066804228,6.36465005832621));
#86293=CARTESIAN_POINT('Ctrl Pts',(-9.94198617976778,-0.534193013242581,
6.32985727279318));
#86294=CARTESIAN_POINT('Ctrl Pts',(-9.94155665446311,-0.000214602085816251,
6.32131009168581));
#86295=CARTESIAN_POINT('Ctrl Pts',(-9.94154134406803,-0.000211681655451256,
6.17868990831418));
#86296=CARTESIAN_POINT('Ctrl Pts',(-9.94196898602932,-0.540425745784602,
6.18733686279454));
#86297=CARTESIAN_POINT('Ctrl Pts',(-9.76726376589108,-2.72004674445215,
6.22222942170057));
#86298=CARTESIAN_POINT('Ctrl Pts',(-8.1962690674157,-6.33113302482017,6.28336758503222));
#86299=CARTESIAN_POINT('Ctrl Pts',(-4.20764072636975,-9.46349996150261,
6.36210439830921));
#86300=CARTESIAN_POINT('Ctrl Pts',(0.789957650256369,-10.3265695617805,
6.44084121158617));
#86301=CARTESIAN_POINT('Ctrl Pts',(5.5981283522494,-8.71338229135328,6.51957802486315));
#86302=CARTESIAN_POINT('Ctrl Pts',(9.06389742585678,-5.0107719422322,6.59831483814014));
#86303=CARTESIAN_POINT('Ctrl Pts',(10.3561917417607,-0.106604931408537,
6.67705165141709));
#86304=CARTESIAN_POINT('Ctrl Pts',(9.1651259445603,4.82312537923973,6.75578846469407));
#86305=CARTESIAN_POINT('Ctrl Pts',(5.77631132522008,8.59629568347027,6.83452527797105));
#86306=CARTESIAN_POINT('Ctrl Pts',(1.00236774113876,10.3081196595228,6.91326209124801));
#86307=CARTESIAN_POINT('Ctrl Pts',(-4.0119383361334,9.54811095403596,6.99199890452499));
#86308=CARTESIAN_POINT('Ctrl Pts',(-8.06420277796297,6.49851564277618,7.07073571780195));
#86309=CARTESIAN_POINT('Ctrl Pts',(-9.73858672170967,2.85661735838654,7.13296605057013));
#86310=CARTESIAN_POINT('Ctrl Pts',(-9.94177600318943,0.608646416867156,
7.16895077891262));
#86311=CARTESIAN_POINT('Ctrl Pts',(-9.9413910139488,0.000173239089263606,
7.17868990282947));
#86312=CARTESIAN_POINT('Origin',(0.,0.,0.));
#86313=CARTESIAN_POINT('',(-9.94201937032046,0.000120688446031495,8.32131009183368));
#86314=CARTESIAN_POINT('',(-9.94202513961595,0.000115166331718865,8.17868990849874));
#86315=CARTESIAN_POINT('',(-9.942,-1.2175438477123E-15,0.));
#86316=CARTESIAN_POINT('Ctrl Pts',(-9.94199999926736,0.000120697445917958,
8.32131009168581));
#86317=CARTESIAN_POINT('Ctrl Pts',(-9.94199849861958,0.123730936968088,
8.31933071676796));
#86318=CARTESIAN_POINT('Ctrl Pts',(-9.93969150660321,0.247335251271708,
8.31735134185011));
#86319=CARTESIAN_POINT('Ctrl Pts',(-9.93508086580521,0.370853326682161,
8.31537196693226));
#86320=CARTESIAN_POINT('Ctrl Pts',(-9.92597342585771,0.614839684222309,
8.31146208997856));
#86321=CARTESIAN_POINT('Ctrl Pts',(-9.90787250252231,0.858527721681658,
8.30755221302486));
#86322=CARTESIAN_POINT('Ctrl Pts',(-9.88082101026864,1.10124482429378,8.30364233607117));
#86323=CARTESIAN_POINT('Ctrl Pts',(-9.8537742008759,1.34391991035369,8.29973313595296));
#86324=CARTESIAN_POINT('Ctrl Pts',(-9.81777994660197,1.58562411863887,8.29582393583475));
#86325=CARTESIAN_POINT('Ctrl Pts',(-9.7729330111231,1.82569010516582,8.29191473571654));
#86326=CARTESIAN_POINT('Ctrl Pts',(-9.72809095789121,2.0657299569876,8.28800596117213));
#86327=CARTESIAN_POINT('Ctrl Pts',(-9.67439819919527,2.30413166770891,8.28409718662772));
#86328=CARTESIAN_POINT('Ctrl Pts',(-9.61200077950874,2.54023719654748,8.2801884120833));
#86329=CARTESIAN_POINT('Ctrl Pts',(-9.54959851746434,2.77636104837876,8.27627933419805));
#86330=CARTESIAN_POINT('Ctrl Pts',(-9.47849031325711,3.0101880904526,8.27237025631281));
#86331=CARTESIAN_POINT('Ctrl Pts',(-9.39887268267154,3.2410733245224,8.26846117842756));
#86332=CARTESIAN_POINT('Ctrl Pts',(-9.31925615151854,3.47195537031916,8.26455215452241));
#86333=CARTESIAN_POINT('Ctrl Pts',(-9.23113052233324,3.69989542501469,8.26064313061727));
#86334=CARTESIAN_POINT('Ctrl Pts',(-9.13474151043455,3.9242657322796,8.25673410671212));
#86335=CARTESIAN_POINT('Ctrl Pts',(-9.03833130066592,4.14868538305886,8.2528242231345));
#86336=CARTESIAN_POINT('Ctrl Pts',(-8.93365418670862,4.36953345967599,8.24891433955687));
#86337=CARTESIAN_POINT('Ctrl Pts',(-8.82100372639414,4.58620292387293,8.24500445597925));
#86338=CARTESIAN_POINT('Ctrl Pts',(-8.74062573554202,4.74080021679601,8.24221468853793));
#86339=CARTESIAN_POINT('Ctrl Pts',(-8.65618946552648,4.89327058548648,8.23942492109661));
#86340=CARTESIAN_POINT('Ctrl Pts',(-8.56781586218719,5.04340116901815,8.23663515365529));
#86341=CARTESIAN_POINT('Ctrl Pts',(-8.44395969055699,5.2538101443029,8.2327252767015));
#86342=CARTESIAN_POINT('Ctrl Pts',(-8.31232996790346,5.45968661003823,8.2288153997477));
#86343=CARTESIAN_POINT('Ctrl Pts',(-8.17328380973805,5.66045897127379,8.2249055227939));
#86344=CARTESIAN_POINT('Ctrl Pts',(-8.03426172173523,5.86119657697606,8.22099632267559));
#86345=CARTESIAN_POINT('Ctrl Pts',(-7.88782592059668,6.05683161164939,8.21708712255727));
#86346=CARTESIAN_POINT('Ctrl Pts',(-7.73437665197683,6.24682173631965,8.21317792243896));
#86347=CARTESIAN_POINT('Ctrl Pts',(-7.58094408856136,6.4367911777772,8.20926914789444));
#86348=CARTESIAN_POINT('Ctrl Pts',(-7.42049975822438,6.62111671826791,8.20536037334992));
#86349=CARTESIAN_POINT('Ctrl Pts',(-7.25348462197907,6.79928855386453,8.2014515988054));
#86350=CARTESIAN_POINT('Ctrl Pts',(-7.08645652450817,6.97747421650344,8.19754252092005));
#86351=CARTESIAN_POINT('Ctrl Pts',(-6.91285679167045,7.14950501337471,8.19363344303471));
#86352=CARTESIAN_POINT('Ctrl Pts',(-6.7331646120328,7.31490658226537,8.18972436514936));
#86353=CARTESIAN_POINT('Ctrl Pts',(-6.55347491374794,7.48030586714096,8.18581534124412));
#86354=CARTESIAN_POINT('Ctrl Pts',(-6.36769314457287,7.63907591878491,8.18190631733887));
#86355=CARTESIAN_POINT('Ctrl Pts',(-6.17633360753728,7.79078090876682,8.17799729343363));
#86356=CARTESIAN_POINT('Ctrl Pts',(-5.98493198671523,7.9425192617078,8.1740874098559));
#86357=CARTESIAN_POINT('Ctrl Pts',(-5.78795036607489,8.08718927333725,8.17017752627818));
#86358=CARTESIAN_POINT('Ctrl Pts',(-5.58593531836972,8.22439606408822,8.16626764270046));
#86359=CARTESIAN_POINT('Ctrl Pts',(-5.44179419717811,8.32229540811536,8.16347787525975));
#86360=CARTESIAN_POINT('Ctrl Pts',(-5.2950912022544,8.41639603664618,8.16068810781903));
#86361=CARTESIAN_POINT('Ctrl Pts',(-5.14603384120051,8.50656803330339,8.15789834037832));
#86362=CARTESIAN_POINT('Ctrl Pts',(-4.93712899405506,8.63294466472426,8.15398846342456));
#86363=CARTESIAN_POINT('Ctrl Pts',(-4.72353458475305,8.75164146899183,8.1500785864708));
#86364=CARTESIAN_POINT('Ctrl Pts',(-4.50583629543312,8.86232493642371,8.14616870951704));
#86365=CARTESIAN_POINT('Ctrl Pts',(-4.28817569167947,8.9729892435344,8.14225950939876));
#86366=CARTESIAN_POINT('Ctrl Pts',(-4.06641287581174,9.07564285596032,8.13835030928048));
#86367=CARTESIAN_POINT('Ctrl Pts',(-3.84115759866731,9.16999848975998,8.1344411091622));
#86368=CARTESIAN_POINT('Ctrl Pts',(-3.61592684386395,9.26434385156485,8.1305323346177));
#86369=CARTESIAN_POINT('Ctrl Pts',(-3.38720464537729,9.35039293019651,8.12662356007319));
#86370=CARTESIAN_POINT('Ctrl Pts',(-3.15562114063695,9.42790640687343,8.12271478552869));
#86371=CARTESIAN_POINT('Ctrl Pts',(-2.92401966383752,9.50542589899081,8.11880570764338));
#86372=CARTESIAN_POINT('Ctrl Pts',(-2.6895567019394,9.57440837365246,8.11489662975807));
#86373=CARTESIAN_POINT('Ctrl Pts',(-2.45287920940295,9.63466385423377,8.11098755187276));
#86374=CARTESIAN_POINT('Ctrl Pts',(-2.21620498512436,9.69491850275266,8.10707852796755));
#86375=CARTESIAN_POINT('Ctrl Pts',(-1.97731656353971,9.7464463310455,8.10316950406234));
#86376=CARTESIAN_POINT('Ctrl Pts',(-1.73687350823773,9.78910794793795,8.09926048015713));
#86377=CARTESIAN_POINT('Ctrl Pts',(-1.49637757470285,9.83177894697251,8.09535059657944));
#86378=CARTESIAN_POINT('Ctrl Pts',(-1.25432660022208,9.86557978848185,8.09144071300176));
#86379=CARTESIAN_POINT('Ctrl Pts',(-1.01138910720974,9.89042244162591,8.08753082942407));
#86380=CARTESIAN_POINT('Ctrl Pts',(-0.838049135644045,9.90814809087096,
8.08474106198316));
#86381=CARTESIAN_POINT('Ctrl Pts',(-0.664258019573462,9.92131414527844,
8.08195129454226));
#86382=CARTESIAN_POINT('Ctrl Pts',(-0.490260069134713,9.92990478628129,
8.07916152710135));
#86383=CARTESIAN_POINT('Ctrl Pts',(-0.246400826084693,9.94194462472183,
8.07525165014757));
#86384=CARTESIAN_POINT('Ctrl Pts',(-0.00206054199540842,9.94499890041737,
8.07134177319379));
#86385=CARTESIAN_POINT('Ctrl Pts',(0.242086977852535,9.93905216281483,8.06743189624002));
#86386=CARTESIAN_POINT('Ctrl Pts',(0.486192233530556,9.933106454647,8.06352269612172));
#86387=CARTESIAN_POINT('Ctrl Pts',(0.730104511490238,9.91816285043824,8.05961349600342));
#86388=CARTESIAN_POINT('Ctrl Pts',(0.973150770743396,9.8942580104524,8.05570429588512));
#86389=CARTESIAN_POINT('Ctrl Pts',(1.21617057084558,9.87035577285909,8.05179552134061));
#86390=CARTESIAN_POINT('Ctrl Pts',(1.45832426162768,9.83749427479797,8.0478867467961));
#86391=CARTESIAN_POINT('Ctrl Pts',(1.69894363287301,9.79576207001376,8.04397797225158));
#86392=CARTESIAN_POINT('Ctrl Pts',(1.93958167740699,9.75402662659793,8.04006889436626));
#86393=CARTESIAN_POINT('Ctrl Pts',(2.17868488774968,9.70341914576017,8.03615981648093));
#86394=CARTESIAN_POINT('Ctrl Pts',(2.41559367981177,9.644079591856,8.03225073859561));
#86395=CARTESIAN_POINT('Ctrl Pts',(2.65249920042207,9.58474085736629,8.02834171469038));
#86396=CARTESIAN_POINT('Ctrl Pts',(2.88721009192831,9.51667036108042,8.02443269078515));
#86397=CARTESIAN_POINT('Ctrl Pts',(3.11907969004966,9.44005857434792,8.02052366687993));
#86398=CARTESIAN_POINT('Ctrl Pts',(3.35100028092948,9.36342993915245,8.01661378330222));
#86399=CARTESIAN_POINT('Ctrl Pts',(3.58007806327249,9.27825634717009,8.01270389972452));
#86400=CARTESIAN_POINT('Ctrl Pts',(3.80568287314964,9.18477772561838,8.00879401614681));
#86401=CARTESIAN_POINT('Ctrl Pts',(3.96665568489176,9.11807916295409,8.006004248706));
#86402=CARTESIAN_POINT('Ctrl Pts',(4.12586072984047,9.04715349288538,8.00321448126518));
#86403=CARTESIAN_POINT('Ctrl Pts',(4.28307547960545,8.97210278786431,8.00042471382436));
#86404=CARTESIAN_POINT('Ctrl Pts',(4.50341295931977,8.86691874362008,7.99651483687059));
#86405=CARTESIAN_POINT('Ctrl Pts',(4.71990760785408,8.75359809155395,7.99260495991682));
#86406=CARTESIAN_POINT('Ctrl Pts',(4.93195907173531,8.63244714520325,7.98869508296305));
#86407=CARTESIAN_POINT('Ctrl Pts',(5.14397382756745,8.51131717119014,7.98478588284476));
#86408=CARTESIAN_POINT('Ctrl Pts',(5.35154669088702,8.38235974775407,7.98087668272647));
#86409=CARTESIAN_POINT('Ctrl Pts',(5.55410272223126,8.24592668842643,7.97696748260818));
#86410=CARTESIAN_POINT('Ctrl Pts',(5.75663670237951,8.1095084818391,7.97305870806369));
#86411=CARTESIAN_POINT('Ctrl Pts',(5.95415470864741,7.96561642085696,7.96914993351919));
#86412=CARTESIAN_POINT('Ctrl Pts',(6.14611069131394,7.81464569703045,7.9652411589747));
#86413=CARTESIAN_POINT('Ctrl Pts',(6.33808157074289,7.66366325710645,7.96133208108938));
#86414=CARTESIAN_POINT('Ctrl Pts',(6.5244893418278,7.50560122753595,7.95742300320406));
#86415=CARTESIAN_POINT('Ctrl Pts',(6.70481995563336,7.34089595094091,7.95351392531874));
#86416=CARTESIAN_POINT('Ctrl Pts',(6.88514807926968,7.17619294874623,7.94960490141353));
#86417=CARTESIAN_POINT('Ctrl Pts',(7.05939900786635,7.00484707357231,7.94569587750831));
#86418=CARTESIAN_POINT('Ctrl Pts',(7.22709404313149,6.82733298526836,7.9417868536031));
#86419=CARTESIAN_POINT('Ctrl Pts',(7.39482595788652,6.6497798580685,7.9378769700254));
#86420=CARTESIAN_POINT('Ctrl Pts',(7.55599890510306,6.46605601035192,7.9339670864477));
#86421=CARTESIAN_POINT('Ctrl Pts',(7.71017218932104,6.27667179411354,7.93005720287));
#86422=CARTESIAN_POINT('Ctrl Pts',(7.82017741070812,6.14154298278805,7.92726743542914));
#86423=CARTESIAN_POINT('Ctrl Pts',(7.92661985514905,6.00353318953312,7.92447766798827));
#86424=CARTESIAN_POINT('Ctrl Pts',(8.02935213713326,5.86283790138475,7.92168790054741));
#86425=CARTESIAN_POINT('Ctrl Pts',(8.17333208895804,5.66565255303739,7.91777802359364));
#86426=CARTESIAN_POINT('Ctrl Pts',(8.3100668280156,5.46313066739671,7.91386814663987));
#86427=CARTESIAN_POINT('Ctrl Pts',(8.43917341423422,5.25582686972111,7.9099582696861));
#86428=CARTESIAN_POINT('Ctrl Pts',(8.56825765092119,5.04855895823009,7.90604906956781));
#86429=CARTESIAN_POINT('Ctrl Pts',(8.68971622267877,4.83651102498741,7.90213986944953));
#86430=CARTESIAN_POINT('Ctrl Pts',(8.80321015901788,4.62026567376427,7.89823066933124));
#86431=CARTESIAN_POINT('Ctrl Pts',(8.91669173987671,4.40404386402059,7.89432189478675));
#86432=CARTESIAN_POINT('Ctrl Pts',(9.02221028635395,4.18362579678715,7.89041312024226));
#86433=CARTESIAN_POINT('Ctrl Pts',(9.11947284906492,3.95961853657239,7.88650434569776));
#86434=CARTESIAN_POINT('Ctrl Pts',(9.21674295984642,3.73559389225267,7.88259526781245));
#86435=CARTESIAN_POINT('Ctrl Pts',(9.30575569214643,3.50797975428848,7.87868618992713));
#86436=CARTESIAN_POINT('Ctrl Pts',(9.38626579840481,3.27740421091083,7.87477711204181));
#86437=CARTESIAN_POINT('Ctrl Pts',(9.46677479290646,3.0468318515299,7.87086808813659));
#86438=CARTESIAN_POINT('Ctrl Pts',(9.53878130572403,2.8132984338617,7.86695906423138));
#86439=CARTESIAN_POINT('Ctrl Pts',(9.60208939387815,2.57744898532885,7.86305004032616));
#86440=CARTESIAN_POINT('Ctrl Pts',(9.66541140474609,2.34154766878874,7.85914015674846));
#86441=CARTESIAN_POINT('Ctrl Pts',(9.72003109486716,2.10332957420899,7.85523027317077));
#86442=CARTESIAN_POINT('Ctrl Pts',(9.76580291369538,1.86345309864746,7.85132038959307));
#86443=CARTESIAN_POINT('Ctrl Pts',(9.79846187331387,1.69229721432065,7.84853062215219));
#86444=CARTESIAN_POINT('Ctrl Pts',(9.82661738093856,1.52029731779854,7.84574085471131));
#86445=CARTESIAN_POINT('Ctrl Pts',(9.85023253620607,1.34769543394173,7.84295108727042));
#86446=CARTESIAN_POINT('Ctrl Pts',(9.88332932771172,1.10579278715493,7.83904121031665));
#86447=CARTESIAN_POINT('Ctrl Pts',(9.90751588863965,0.862633347076693,7.83513133336288));
#86448=CARTESIAN_POINT('Ctrl Pts',(9.92271851932728,0.618887054477162,7.83122145640911));
#86449=CARTESIAN_POINT('Ctrl Pts',(9.93791851830041,0.375182956591622,7.82731225629082));
#86450=CARTESIAN_POINT('Ctrl Pts',(9.94413767412424,0.130892488609745,7.82340305617253));
#86451=CARTESIAN_POINT('Ctrl Pts',(9.94135426861737,-0.113310660766393,
7.81949385605424));
#86452=CARTESIAN_POINT('Ctrl Pts',(9.93857116612502,-0.357487225046637,
7.81558508150975));
#86453=CARTESIAN_POINT('Ctrl Pts',(9.92678746236054,-0.601576209516069,
7.81167630696525));
#86454=CARTESIAN_POINT('Ctrl Pts',(9.90603355599169,-0.844904247572915,
7.80776753242075));
#86455=CARTESIAN_POINT('Ctrl Pts',(9.88527803901394,-1.0882511691254,7.80385845453544));
#86456=CARTESIAN_POINT('Ctrl Pts',(9.85555094918939,-1.330836746692,7.79994937665012));
#86457=CARTESIAN_POINT('Ctrl Pts',(9.81693464940344,-1.57199175867503,7.7960402987648));
#86458=CARTESIAN_POINT('Ctrl Pts',(9.77831888286646,-1.81314344057035,7.79213127485958));
#86459=CARTESIAN_POINT('Ctrl Pts',(9.73081419822735,-2.05286431991402,7.78822225095437));
#86460=CARTESIAN_POINT('Ctrl Pts',(9.67455439391132,-2.29049367588109,7.78431322704915));
#86461=CARTESIAN_POINT('Ctrl Pts',(9.61828221693993,-2.52817529129268,7.78040334347145));
#86462=CARTESIAN_POINT('Ctrl Pts',(9.55325113659201,-2.76376419112236,7.77649345989376));
#86463=CARTESIAN_POINT('Ctrl Pts',(9.47964564948824,-2.99661181338835,7.77258357631606));
#86464=CARTESIAN_POINT('Ctrl Pts',(9.42712690121589,-3.16275249312277,7.76979380887519));
#86465=CARTESIAN_POINT('Ctrl Pts',(9.37024392991821,-3.32749782564914,7.76700404143432));
#86466=CARTESIAN_POINT('Ctrl Pts',(9.30907916889137,-3.49061728456626,7.76421427399346));
#86467=CARTESIAN_POINT('Ctrl Pts',(9.22335636418052,-3.71923025200932,7.76030439703968));
#86468=CARTESIAN_POINT('Ctrl Pts',(9.12919493734011,-3.94471889634479,7.7563945200859));
#86469=CARTESIAN_POINT('Ctrl Pts',(9.02684810190676,-4.16645860955107,7.75248464313212));
#86470=CARTESIAN_POINT('Ctrl Pts',(8.92451898364732,-4.38815993758361,7.74857544301383));
#86471=CARTESIAN_POINT('Ctrl Pts',(8.81400740279927,-4.60611337560326,7.74466624289554));
#86472=CARTESIAN_POINT('Ctrl Pts',(8.69561410139413,-4.81971569697172,7.74075704277724));
#86473=CARTESIAN_POINT('Ctrl Pts',(8.57723368883694,-5.03329476459347,7.73684826823274));
#86474=CARTESIAN_POINT('Ctrl Pts',(8.45097340479124,-5.24252341628014,7.73293949368823));
#86475=CARTESIAN_POINT('Ctrl Pts',(8.31717970653713,-5.44682345309328,7.72903071914373));
#86476=CARTESIAN_POINT('Ctrl Pts',(8.18337562521034,-5.65113934463021,7.7251216412584));
#86477=CARTESIAN_POINT('Ctrl Pts',(8.04203711248242,-5.85052562081983,7.72121256337308));
#86478=CARTESIAN_POINT('Ctrl Pts',(7.89355439149914,-6.04443240250436,7.71730348548776));
#86479=CARTESIAN_POINT('Ctrl Pts',(7.74507372090031,-6.2383365065477,7.71339446158253));
#86480=CARTESIAN_POINT('Ctrl Pts',(7.58944921142076,-6.42676104609965,7.70948543767731));
#86481=CARTESIAN_POINT('Ctrl Pts',(7.42711231873426,-6.60918804429907,7.70557641377209));
#86482=CARTESIAN_POINT('Ctrl Pts',(7.2647397249207,-6.79165516184126,7.70166653019439));
#86483=CARTESIAN_POINT('Ctrl Pts',(7.09565198389555,-6.96812189232981,7.69775664661669));
#86484=CARTESIAN_POINT('Ctrl Pts',(6.92031939813044,-7.13810503059878,7.69384676303898));
#86485=CARTESIAN_POINT('Ctrl Pts',(6.79521666057704,-7.25939084773635,7.69105699559815));
#86486=CARTESIAN_POINT('Ctrl Pts',(6.66693544661113,-7.37737655515755,7.68826722815731));
#86487=CARTESIAN_POINT('Ctrl Pts',(6.53565775611913,-7.49189840393474,7.68547746071647));
#86488=CARTESIAN_POINT('Ctrl Pts',(6.35167123126217,-7.65240150920526,7.6815675837627));
#86489=CARTESIAN_POINT('Ctrl Pts',(6.16174122976612,-7.80614837115822,7.67765770680893));
#86490=CARTESIAN_POINT('Ctrl Pts',(5.96638715909732,-7.95270949222708,7.67374782985516));
#86491=CARTESIAN_POINT('Ctrl Pts',(5.77106690600597,-8.09924524222459,7.66983862973687));
#86492=CARTESIAN_POINT('Ctrl Pts',(5.57032468222324,-8.23859756634138,7.66592942961858));
#86493=CARTESIAN_POINT('Ctrl Pts',(5.36471157364193,-8.3703783505665,7.66202022950029));
#86494=CARTESIAN_POINT('Ctrl Pts',(5.15912084906475,-8.50214478851945,7.6581114549558));
#86495=CARTESIAN_POINT('Ctrl Pts',(4.9486605343707,-8.62634118119008,7.65420268041131));
#86496=CARTESIAN_POINT('Ctrl Pts',(4.7339100668253,-8.7426231463566,7.65029390586682));
#86497=CARTESIAN_POINT('Ctrl Pts',(4.51914293354909,-8.85891413559627,7.6463848279815));
#86498=CARTESIAN_POINT('Ctrl Pts',(4.30008522719591,-8.9672893338659,7.64247575009619));
#86499=CARTESIAN_POINT('Ctrl Pts',(4.07734145772143,-9.06745006256699,7.63856667221087));
#86500=CARTESIAN_POINT('Ctrl Pts',(3.85460076409528,-9.16760940815774,7.63465764830566));
#86501=CARTESIAN_POINT('Ctrl Pts',(3.62817436566375,-9.25955439795779,7.63074862440044));
#86502=CARTESIAN_POINT('Ctrl Pts',(3.39868791455605,-9.34303400718689,7.62683960049522));
#86503=CARTESIAN_POINT('Ctrl Pts',(3.16915099479163,-9.42653197525033,7.62292971691752));
#86504=CARTESIAN_POINT('Ctrl Pts',(2.93655294083511,-9.50156074593007,7.61901983333983));
#86505=CARTESIAN_POINT('Ctrl Pts',(2.70153708495892,-9.56791834092409,7.61510994976214));
#86506=CARTESIAN_POINT('Ctrl Pts',(2.53384933421514,-9.61526559674149,7.61232018232126));
#86507=CARTESIAN_POINT('Ctrl Pts',(2.36493103553724,-9.65819932922395,7.60953041488038));
#86508=CARTESIAN_POINT('Ctrl Pts',(2.19502011278985,-9.69666183304585,7.6067406474395));
#86509=CARTESIAN_POINT('Ctrl Pts',(1.95688886524932,-9.75056727873787,7.60283077048573));
#86510=CARTESIAN_POINT('Ctrl Pts',(1.71673450088473,-9.79570467238615,7.59892089353196));
#86511=CARTESIAN_POINT('Ctrl Pts',(1.47521806992349,-9.83194261812849,7.59501101657819));
#86512=CARTESIAN_POINT('Ctrl Pts',(1.23374344766685,-9.86817429075075,7.5911018164599));
#86513=CARTESIAN_POINT('Ctrl Pts',(0.99090750656723,-9.89550954923192,7.58719261634161));
#86514=CARTESIAN_POINT('Ctrl Pts',(0.747379528890581,-9.91386845987959,
7.58328341622332));
#86515=CARTESIAN_POINT('Ctrl Pts',(0.503878062807174,-9.93222537189048,
7.57937464167882));
#86516=CARTESIAN_POINT('Ctrl Pts',(0.259684989983711,-9.94160786617092,
7.57546586713432));
#86517=CARTESIAN_POINT('Ctrl Pts',(0.0154737816735091,-9.94198795825466,
7.57155709258982));
#86518=CARTESIAN_POINT('Ctrl Pts',(-0.228756378670423,-9.94236807983549,
7.5676480147045));
#86519=CARTESIAN_POINT('Ctrl Pts',(-0.473004396991685,-9.93374439971354,
7.56373893681918));
#86520=CARTESIAN_POINT('Ctrl Pts',(-0.71659643482113,-9.91614106140093,
7.55982985893386));
#86521=CARTESIAN_POINT('Ctrl Pts',(-0.960185108910316,-9.89853796617122,
7.55592083502865));
#86522=CARTESIAN_POINT('Ctrl Pts',(-1.20311754117273,-9.87195548300951,
7.55201181112343));
#86523=CARTESIAN_POINT('Ctrl Pts',(-1.4447239111017,-9.83646973363366,7.54810278721821));
#86524=CARTESIAN_POINT('Ctrl Pts',(-1.6863834151002,-9.8009761802323,7.54419290364051));
#86525=CARTESIAN_POINT('Ctrl Pts',(-1.92671599645066,-9.75657548794391,
7.54028302006281));
#86526=CARTESIAN_POINT('Ctrl Pts',(-2.16505956076288,-9.70339533866106,
7.53637313648511));
#86527=CARTESIAN_POINT('Ctrl Pts',(-2.33512168722852,-9.66545041114058,
7.53358336904425));
#86528=CARTESIAN_POINT('Ctrl Pts',(-2.50417135425084,-9.62303688626508,
7.53079360160339));
#86529=CARTESIAN_POINT('Ctrl Pts',(-2.67197176687381,-9.57621693974344,
7.52800383416253));
#86530=CARTESIAN_POINT('Ctrl Pts',(-2.90714512094575,-9.51059848452723,
7.52409395720876));
#86531=CARTESIAN_POINT('Ctrl Pts',(-3.13993609929161,-9.43630270113784,
7.52018408025499));
#86532=CARTESIAN_POINT('Ctrl Pts',(-3.36970052527798,-9.35352780345156,
7.51627420330122));
#86533=CARTESIAN_POINT('Ctrl Pts',(-3.59942517693922,-9.27076723485769,
7.51236500318294));
#86534=CARTESIAN_POINT('Ctrl Pts',(-3.82612405852241,-9.17953057701249,
7.50845580306465));
#86535=CARTESIAN_POINT('Ctrl Pts',(-4.04917018174292,-9.08006524421956,
7.50454660294637));
#86536=CARTESIAN_POINT('Ctrl Pts',(-4.27219202312049,-8.98061073968741,
7.50063782840187));
#86537=CARTESIAN_POINT('Ctrl Pts',(-4.49156164421575,-8.8729294629758,7.49672905385738));
#86538=CARTESIAN_POINT('Ctrl Pts',(-4.70667303463914,-8.75731653790137,
7.49282027931288));
#86539=CARTESIAN_POINT('Ctrl Pts',(-4.92180111880257,-8.64169464067482,
7.48891120142756));
#86540=CARTESIAN_POINT('Ctrl Pts',(-5.13267006359499,-8.5181399951333,7.48500212354224));
#86541=CARTESIAN_POINT('Ctrl Pts',(-5.33869828494172,-8.38699377741276,
7.48109304565692));
#86542=CARTESIAN_POINT('Ctrl Pts',(-5.54472366126301,-8.25584937067871,
7.47718402175172));
#86543=CARTESIAN_POINT('Ctrl Pts',(-5.74590821245139,-8.11711375369856,
7.47327499784651));
#86544=CARTESIAN_POINT('Ctrl Pts',(-5.9416985690445,-7.97117194110217,7.4693659739413));
#86545=CARTESIAN_POINT('Ctrl Pts',(-6.1375319838504,-7.82519803298416,7.4654560903636));
#86546=CARTESIAN_POINT('Ctrl Pts',(-6.32796860821478,-7.67201492936341,
7.4615462067859));
#86547=CARTESIAN_POINT('Ctrl Pts',(-6.5124863523695,-7.5120493548832,7.4576363232082));
#86548=CARTESIAN_POINT('Ctrl Pts',(-6.64414285432868,-7.3979112373464,7.45484655576732));
#86549=CARTESIAN_POINT('Ctrl Pts',(-6.77278667189716,-7.28032099449203,
7.45205678832644));
#86550=CARTESIAN_POINT('Ctrl Pts',(-6.89823892120803,-7.15944577365669,
7.44926702088556));
#86551=CARTESIAN_POINT('Ctrl Pts',(-7.07406105290008,-6.99003837671675,
7.44535714393178));
#86552=CARTESIAN_POINT('Ctrl Pts',(-7.24366659743927,-6.81412515296562,
7.441447266978));
#86553=CARTESIAN_POINT('Ctrl Pts',(-7.40658272194256,-6.63218639537686,
7.43753739002422));
#86554=CARTESIAN_POINT('Ctrl Pts',(-7.56947064417336,-6.45027913305252,
7.43362818990593));
#86555=CARTESIAN_POINT('Ctrl Pts',(-7.72567127109786,-6.26234862782684,
7.42971898978765));
#86556=CARTESIAN_POINT('Ctrl Pts',(-7.87475025689373,-6.06891031335545,
7.42580978966936));
#86557=CARTESIAN_POINT('Ctrl Pts',(-8.02381301325494,-5.87549305748242,
7.42190101512485));
#86558=CARTESIAN_POINT('Ctrl Pts',(-8.1657555054564,-5.67656941152338,7.41799224058034));
#86559=CARTESIAN_POINT('Ctrl Pts',(-8.30018450206481,-5.47268683844445,
7.41408346603584));
#86560=CARTESIAN_POINT('Ctrl Pts',(-8.43462393104828,-5.26878844303907,
7.41017438815051));
#86561=CARTESIAN_POINT('Ctrl Pts',(-8.5615485424511,-5.05993058387834,7.40626531026519));
#86562=CARTESIAN_POINT('Ctrl Pts',(-8.68060846738418,-4.84668965748562,
7.40235623237986));
#86563=CARTESIAN_POINT('Ctrl Pts',(-8.7996667482294,-4.6334516757178,7.39844720847464));
#86564=CARTESIAN_POINT('Ctrl Pts',(-8.91086042494945,-4.4158309935355,7.39453818456942));
#86565=CARTESIAN_POINT('Ctrl Pts',(-9.01388527420231,-4.19442919400469,
7.3906291606642));
#86566=CARTESIAN_POINT('Ctrl Pts',(-9.11693278067868,-3.97297870379297,
7.3867192770865));
#86567=CARTESIAN_POINT('Ctrl Pts',(-9.21180775078023,-3.74774568848959,
7.38280939350879));
#86568=CARTESIAN_POINT('Ctrl Pts',(-9.29825329373128,-3.51935358917165,
7.37889950993109));
#86569=CARTESIAN_POINT('Ctrl Pts',(-9.35993363697869,-3.35639199971292,
7.37610974249025));
#86570=CARTESIAN_POINT('Ctrl Pts',(-9.41732349670219,-3.19182255840282,
7.37331997504941));
#86571=CARTESIAN_POINT('Ctrl Pts',(-9.47034479553102,-3.02587730315665,
7.37053020760858));
#86572=CARTESIAN_POINT('Ctrl Pts',(-9.54829975444413,-2.78189505752545,
7.36642853128168));
#86573=CARTESIAN_POINT('Ctrl Pts',(-9.61683348021652,-2.53486048040967,
7.36232685495478));
#86574=CARTESIAN_POINT('Ctrl Pts',(-9.67573071718072,-2.28551943518437,
7.35822517862788));
#86575=CARTESIAN_POINT('Ctrl Pts',(-9.73198857835279,-2.04735216911533,
7.35430731169108));
#86576=CARTESIAN_POINT('Ctrl Pts',(-9.77945461065712,-1.80708091427208,
7.35038944475427));
#86577=CARTESIAN_POINT('Ctrl Pts',(-9.81799288608731,-1.56536886666977,
7.34647157781746));
#86578=CARTESIAN_POINT('Ctrl Pts',(-9.85652590123158,-1.32368981157854,
7.34255424565031));
#86579=CARTESIAN_POINT('Ctrl Pts',(-9.88613354943089,-1.08057063060592,
7.33863691348316));
#86580=CARTESIAN_POINT('Ctrl Pts',(-9.90673132562275,-0.836682999662867,
7.33471958131601));
#86581=CARTESIAN_POINT('Ctrl Pts',(-9.92732820978895,-0.592805930735089,
7.33080241879634));
#86582=CARTESIAN_POINT('Ctrl Pts',(-9.93891597733403,-0.348160754885544,
7.32688525627666));
#86583=CARTESIAN_POINT('Ctrl Pts',(-9.94146204244371,-0.103423685154355,
7.32296809375699));
#86584=CARTESIAN_POINT('Ctrl Pts',(-9.94182126345331,-0.0688940508019636,
7.32241542639993));
#86585=CARTESIAN_POINT('Ctrl Pts',(-9.94200058483451,-0.0343625907378737,
7.32186275904287));
#86586=CARTESIAN_POINT('Ctrl Pts',(-9.94199999856713,0.00016879341615152,
7.32131009168581));
#86587=CARTESIAN_POINT('Ctrl Pts',(-9.94199999849644,0.000172907010996282,
7.17868990831418));
#86588=CARTESIAN_POINT('Ctrl Pts',(-9.94200425406554,-0.244518547686264,
7.18260616056646));
#86589=CARTESIAN_POINT('Ctrl Pts',(-9.93297068691858,-0.489214384721641,
7.18652241281874));
#86590=CARTESIAN_POINT('Ctrl Pts',(-9.9149243805595,-0.733238384010886,
7.19043866507102));
#86591=CARTESIAN_POINT('Ctrl Pts',(-9.89687582244228,-0.977292831803824,
7.19435540598024));
#86592=CARTESIAN_POINT('Ctrl Pts',(-9.86981229670883,-1.22067499698101,
7.19827214688947));
#86593=CARTESIAN_POINT('Ctrl Pts',(-9.83381087633608,-1.46271242848835,
7.20218888779869));
#86594=CARTESIAN_POINT('Ctrl Pts',(-9.79780826943771,-1.70475783700344,
7.20610575779485));
#86595=CARTESIAN_POINT('Ctrl Pts',(-9.75286722345113,-1.94545814884843,
7.21002262779102));
#86596=CARTESIAN_POINT('Ctrl Pts',(-9.69911630576427,-2.1841490075674,7.21393949778719));
#86597=CARTESIAN_POINT('Ctrl Pts',(-9.64535454834625,-2.42288800211082,
7.21785715768276));
#86598=CARTESIAN_POINT('Ctrl Pts',(-9.58277943156352,-2.659616462913,7.22177481757832));
#86599=CARTESIAN_POINT('Ctrl Pts',(-9.51157027869964,-2.89368188185186,
7.22569247747389));
#86600=CARTESIAN_POINT('Ctrl Pts',(-9.49632104290438,-2.94380631981191,
7.22653143310123));
#86601=CARTESIAN_POINT('Ctrl Pts',(-9.48067604143394,-2.99380868649339,
7.22737038872857));
#86602=CARTESIAN_POINT('Ctrl Pts',(-9.46463733237618,-3.043682665225,7.22820934435591));
#86603=CARTESIAN_POINT('Ctrl Pts',(-9.38989037691179,-3.27611584009324,
7.23211922130968));
#86604=CARTESIAN_POINT('Ctrl Pts',(-9.30656568547276,-3.5058297900949,7.23602909826345));
#86605=CARTESIAN_POINT('Ctrl Pts',(-9.21488646225066,-3.73218856541701,
7.23993897521723));
#86606=CARTESIAN_POINT('Ctrl Pts',(-9.12322310954142,-3.9585081559628,7.24384817533551));
#86607=CARTESIAN_POINT('Ctrl Pts',(-9.02320821725852,-4.18147347157786,
7.24775737545379));
#86608=CARTESIAN_POINT('Ctrl Pts',(-8.91511348169684,-4.40046765792766,
7.25166657557206));
#86609=CARTESIAN_POINT('Ctrl Pts',(-8.80703051383299,-4.61943800354738,
7.25557535011656));
#86610=CARTESIAN_POINT('Ctrl Pts',(-8.69086958300834,-4.83443783183468,
7.25948412466105));
#86611=CARTESIAN_POINT('Ctrl Pts',(-8.56694923994193,-5.04487311240415,
7.26339289920555));
#86612=CARTESIAN_POINT('Ctrl Pts',(-8.44301928002533,-5.2553247238239,7.26730197709087));
#86613=CARTESIAN_POINT('Ctrl Pts',(-8.31132884421814,-5.46121083658938,
7.27121105497619));
#86614=CARTESIAN_POINT('Ctrl Pts',(-8.17224154714534,-5.66196362537871,
7.27512013286151));
#86615=CARTESIAN_POINT('Ctrl Pts',(-8.03315617071619,-5.86271364199129,
7.27902915676673));
#86616=CARTESIAN_POINT('Ctrl Pts',(-7.88667429864726,-6.05833024714368,
7.28293818067196));
#86617=CARTESIAN_POINT('Ctrl Pts',(-7.73320224947866,-6.24827551958604,
7.28684720457718));
#86618=CARTESIAN_POINT('Ctrl Pts',(-7.57969644873958,-6.43826256478954,
7.29075708815488));
#86619=CARTESIAN_POINT('Ctrl Pts',(-7.41919757461236,-6.62257556633314,
7.29466697173257));
#86620=CARTESIAN_POINT('Ctrl Pts',(-7.25215240306761,-6.80070948671392,
7.29857685531027));
#86621=CARTESIAN_POINT('Ctrl Pts',(-7.13296287441027,-6.92781102345233,
7.30136662275114));
#86622=CARTESIAN_POINT('Ctrl Pts',(-7.01044143160069,-7.05176743944137,
7.30415639019201));
#86623=CARTESIAN_POINT('Ctrl Pts',(-6.88476207621815,-7.17240651063981,
7.30694615763288));
#86624=CARTESIAN_POINT('Ctrl Pts',(-6.70862165391008,-7.34148294235024,
7.31085603458667));
#86625=CARTESIAN_POINT('Ctrl Pts',(-6.52622298655171,-7.50409360981993,
7.31476591154045));
#86626=CARTESIAN_POINT('Ctrl Pts',(-6.33806445520069,-7.6597847856008,7.31867578849423));
#86627=CARTESIAN_POINT('Ctrl Pts',(-6.14993849581341,-7.81544900981432,
7.32258498861253));
#86628=CARTESIAN_POINT('Ctrl Pts',(-5.95605487869896,-7.96419595486187,
7.32649418873084));
#86629=CARTESIAN_POINT('Ctrl Pts',(-5.75694559672558,-8.10561172252545,
7.33040338884914));
#86630=CARTESIAN_POINT('Ctrl Pts',(-5.55785799071956,-8.24701209500738,
7.33431216339364));
#86631=CARTESIAN_POINT('Ctrl Pts',(-5.35354608419188,-8.38108272141303,
7.33822093793813));
#86632=CARTESIAN_POINT('Ctrl Pts',(-5.14457227027934,-8.5074520366484,7.34212971248263));
#86633=CARTESIAN_POINT('Ctrl Pts',(-4.93558223893361,-8.63383115878678,
7.34603879036796));
#86634=CARTESIAN_POINT('Ctrl Pts',(-4.7219298155718,-8.75250762783033,7.34994786825329));
#86635=CARTESIAN_POINT('Ctrl Pts',(-4.50420461246222,-8.8631543374283,7.35385694613861));
#86636=CARTESIAN_POINT('Ctrl Pts',(-4.28648241590029,-8.97379951911586,
7.35776597004384));
#86637=CARTESIAN_POINT('Ctrl Pts',(-4.06468780291484,-9.07641503795604,
7.36167499394906));
#86638=CARTESIAN_POINT('Ctrl Pts',(-3.83943377164353,-9.17072038136389,
7.36558401785429));
#86639=CARTESIAN_POINT('Ctrl Pts',(-3.61413020250931,-9.26504646440134,
7.36949390143199));
#86640=CARTESIAN_POINT('Ctrl Pts',(-3.38536595317228,-9.35105861098243,
7.37340378500969));
#86641=CARTESIAN_POINT('Ctrl Pts',(-3.15377401580192,-9.42852445811393,
7.37731366858738));
#86642=CARTESIAN_POINT('Ctrl Pts',(-2.98852928828145,-9.48379763794366,
7.38010343602821));
#86643=CARTESIAN_POINT('Ctrl Pts',(-2.82184538566752,-9.53472085093501,
7.38289320346904));
#86644=CARTESIAN_POINT('Ctrl Pts',(-2.65395721633737,-9.58122513532851,
7.38568297090986));
#86645=CARTESIAN_POINT('Ctrl Pts',(-2.4186608706746,-9.64640118804926,7.38959284786364));
#86646=CARTESIAN_POINT('Ctrl Pts',(-2.18092646501398,-9.70291539328967,
7.39350272481741));
#86647=CARTESIAN_POINT('Ctrl Pts',(-1.94140804813236,-9.75060504741356,
7.39741260177118));
#86648=CARTESIAN_POINT('Ctrl Pts',(-1.70193109408101,-9.79828644602183,
7.40132180188947));
#86649=CARTESIAN_POINT('Ctrl Pts',(-1.46067102007947,-9.83714628825918,
7.40523100200776));
#86650=CARTESIAN_POINT('Ctrl Pts',(-1.21829254648774,-9.86707288263203,
7.40914020212605));
#86651=CARTESIAN_POINT('Ctrl Pts',(-0.975940459349413,-9.89699621905596,
7.41304897667054));
#86652=CARTESIAN_POINT('Ctrl Pts',(-0.732470493816496,-9.91798821507781,
7.41695775121503));
#86653=CARTESIAN_POINT('Ctrl Pts',(-0.488554026537994,-9.92998887024319,
7.42086652575952));
#86654=CARTESIAN_POINT('Ctrl Pts',(-0.244618630098674,-9.94199045672056,
7.42477560364484));
#86655=CARTESIAN_POINT('Ctrl Pts',(-0.00023694251214787,-9.94499929121525,
7.42868468153016));
#86656=CARTESIAN_POINT('Ctrl Pts',(0.243916812219465,-9.93900742472389,
7.43259375941547));
#86657=CARTESIAN_POINT('Ctrl Pts',(0.488067195453498,-9.93301564097369,
7.43650278332068));
#86658=CARTESIAN_POINT('Ctrl Pts',(0.731989371933233,-9.91802341375415,
7.44041180722589));
#86659=CARTESIAN_POINT('Ctrl Pts',(0.975010657641103,-9.89407490458235,
7.44432083113109));
#86660=CARTESIAN_POINT('Ctrl Pts',(1.21808538858709,-9.87012112865472,7.44823071470879));
#86661=CARTESIAN_POINT('Ctrl Pts',(1.4602585537056,-9.83720716155028,7.45214059828648));
#86662=CARTESIAN_POINT('Ctrl Pts',(1.70086273280917,-9.79542903420472,7.45605048186417));
#86663=CARTESIAN_POINT('Ctrl Pts',(1.87253784580596,-9.76561964037139,7.45884024930506));
#86664=CARTESIAN_POINT('Ctrl Pts',(2.04341428824696,-9.73129853269632,7.46163001674595));
#86665=CARTESIAN_POINT('Ctrl Pts',(2.21325257474585,-9.69251654836766,7.46441978418684));
#86666=CARTESIAN_POINT('Ctrl Pts',(2.4512820221177,-9.63816334869736,7.46832966114061));
#86667=CARTESIAN_POINT('Ctrl Pts',(2.68734471051714,-9.57502928361013,7.47223953809439));
#86668=CARTESIAN_POINT('Ctrl Pts',(2.92078776089226,-9.50328168875478,7.47614941504817));
#86669=CARTESIAN_POINT('Ctrl Pts',(3.15419040013818,-9.43154651406496,7.48005861516645));
#86670=CARTESIAN_POINT('Ctrl Pts',(3.38497403880572,-9.3512008684512,7.48396781528473));
#86671=CARTESIAN_POINT('Ctrl Pts',(3.61250062547665,-9.26246205017493,7.48787701540301));
#86672=CARTESIAN_POINT('Ctrl Pts',(3.84000244254066,-9.17373289242089,7.4917857899475));
#86673=CARTESIAN_POINT('Ctrl Pts',(4.06424765453406,-9.07661248822206,7.495694564492));
#86674=CARTESIAN_POINT('Ctrl Pts',(4.28461689387206,-8.97136678955588,7.49960333903649));
#86675=CARTESIAN_POINT('Ctrl Pts',(4.50500323498623,-8.86611292328706,7.50351241692182));
#86676=CARTESIAN_POINT('Ctrl Pts',(4.72151274811741,-8.75273262060361,7.50742149480714));
#86677=CARTESIAN_POINT('Ctrl Pts',(4.93354827288646,-8.63153899597859,7.51133057269246));
#86678=CARTESIAN_POINT('Ctrl Pts',(5.14558086967583,-8.51034704490553,7.51523959659768));
#86679=CARTESIAN_POINT('Ctrl Pts',(5.35313935930815,-8.38134212857493,7.51914862050289));
#86680=CARTESIAN_POINT('Ctrl Pts',(5.5556526779625,-8.24488249290723,7.52305764440811));
#86681=CARTESIAN_POINT('Ctrl Pts',(5.75821053334288,-8.10839284703848,7.5269675279858));
#86682=CARTESIAN_POINT('Ctrl Pts',(5.95572076759188,-7.96444536181908,7.53087741156349));
#86683=CARTESIAN_POINT('Ctrl Pts',(6.14764157634194,-7.81344143440213,7.53478729514119));
#86684=CARTESIAN_POINT('Ctrl Pts',(6.28458028892445,-7.70569760219314,7.53757706258206));
#86685=CARTESIAN_POINT('Ctrl Pts',(6.41867400228529,-7.59436219430282,7.54036683002293));
#86686=CARTESIAN_POINT('Ctrl Pts',(6.54973608136051,-7.47959365637762,7.54315659746381));
#86687=CARTESIAN_POINT('Ctrl Pts',(6.7334204254323,-7.31874481468657,7.54706647441758));
#86688=CARTESIAN_POINT('Ctrl Pts',(6.91120480998118,-7.151101694818,7.55097635137135));
#86689=CARTESIAN_POINT('Ctrl Pts',(7.08259408263057,-6.97712154550043,7.55488622832512));
#86690=CARTESIAN_POINT('Ctrl Pts',(7.25395368622877,-6.80317151373853,7.55879542844342));
#86691=CARTESIAN_POINT('Ctrl Pts',(7.41892019123391,-6.6228868419756,7.56270462856172));
#86692=CARTESIAN_POINT('Ctrl Pts',(7.57703521653159,-6.43676171125202,7.56661382868002));
#86693=CARTESIAN_POINT('Ctrl Pts',(7.73513302868866,-6.25065684298004,7.57052260322452));
#86694=CARTESIAN_POINT('Ctrl Pts',(7.88638066901538,-6.05871299882367,7.57443137776902));
#86695=CARTESIAN_POINT('Ctrl Pts',(8.03035930006862,-5.86145830931189,7.57834015231353));
#86696=CARTESIAN_POINT('Ctrl Pts',(8.17434910459688,-5.66418831183164,7.58224923019884));
#86697=CARTESIAN_POINT('Ctrl Pts',(8.31106860489795,-5.46160687006061,7.58615830808415));
#86698=CARTESIAN_POINT('Ctrl Pts',(8.44014090012236,-5.25427307875045,7.59006738596947));
#86699=CARTESIAN_POINT('Ctrl Pts',(8.56921141299867,-5.04694215049458,7.59397640987466));
#86700=CARTESIAN_POINT('Ctrl Pts',(8.69063478559434,-4.83485924302001,7.59788543377986));
#86701=CARTESIAN_POINT('Ctrl Pts',(8.8040785123749,-4.61861078116988,7.60179445768506));
#86702=CARTESIAN_POINT('Ctrl Pts',(8.91754718769865,-4.4023147619603,7.60570434126275));
#86703=CARTESIAN_POINT('Ctrl Pts',(9.02303257948988,-4.18185160573529,7.60961422484044));
#86704=CARTESIAN_POINT('Ctrl Pts',(9.12024842102828,-3.95783182294689,7.61352410841814));
#86705=CARTESIAN_POINT('Ctrl Pts',(9.18961355277002,-3.797989954585,7.61631387585902));
#86706=CARTESIAN_POINT('Ctrl Pts',(9.2547695724198,-3.63633788959191,7.61910364329989));
#86707=CARTESIAN_POINT('Ctrl Pts',(9.31562744933925,-3.47310368764268,7.62189341074077));
#86708=CARTESIAN_POINT('Ctrl Pts',(9.40092015400574,-3.24432990710551,7.62580328769455));
#86709=CARTESIAN_POINT('Ctrl Pts',(9.47779447774866,-3.01237766767267,7.62971316464833));
#86710=CARTESIAN_POINT('Ctrl Pts',(9.54603172979293,-2.77788448532092,7.6336230416021));
#86711=CARTESIAN_POINT('Ctrl Pts',(9.61425716934443,-2.54343189588486,7.6375322417204));
#86712=CARTESIAN_POINT('Ctrl Pts',(9.67384844358402,-2.30643951060475,7.6414414418387));
#86713=CARTESIAN_POINT('Ctrl Pts',(9.7246367590727,-2.06755989129506,7.64535064195699));
#86714=CARTESIAN_POINT('Ctrl Pts',(9.77541954550824,-1.82870627753594,7.64925941650152));
#86715=CARTESIAN_POINT('Ctrl Pts',(9.81740122839898,-1.58796611404812,7.65316819104604));
#86716=CARTESIAN_POINT('Ctrl Pts',(9.85046393545143,-1.34600306699901,7.65707696559056));
#86717=CARTESIAN_POINT('Ctrl Pts',(9.88352920833822,-1.10402124238596,7.66098604347588));
#86718=CARTESIAN_POINT('Ctrl Pts',(9.90767408132998,-0.860816621909657,
7.6648951213612));
#86719=CARTESIAN_POINT('Ctrl Pts',(9.92283229194109,-0.617060212630194,
7.66880419924652));
#86720=CARTESIAN_POINT('Ctrl Pts',(9.93799029323388,-0.373307169360157,
7.67271322315175));
#86721=CARTESIAN_POINT('Ctrl Pts',(9.94416186499507,-0.129002632442874,
7.67662224705698));
#86722=CARTESIAN_POINT('Ctrl Pts',(9.94133279304864,0.11517941593772,7.68053127096221));
#86723=CARTESIAN_POINT('Ctrl Pts',(9.93850309893275,0.359415164830415,7.68444115453991));
#86724=CARTESIAN_POINT('Ctrl Pts',(9.9266688081334,0.603528090943824,7.68835103811762));
#86725=CARTESIAN_POINT('Ctrl Pts',(9.90586783682596,0.846844967710685,7.69226092169532));
#86726=CARTESIAN_POINT('Ctrl Pts',(9.89102599528838,1.02045563593478,7.69505068913613));
#86727=CARTESIAN_POINT('Ctrl Pts',(9.87162025165008,1.19366104614316,7.69784045657694));
#86728=CARTESIAN_POINT('Ctrl Pts',(9.84768052877536,1.36621821213837,7.70063022401775));
#86729=CARTESIAN_POINT('Ctrl Pts',(9.81412885368649,1.60805818656187,7.70454010097152));
#86730=CARTESIAN_POINT('Ctrl Pts',(9.77165905958133,1.84869862293395,7.70844997792529));
#86731=CARTESIAN_POINT('Ctrl Pts',(9.72038135817977,2.0874746109956,7.71235985487907));
#86732=CARTESIAN_POINT('Ctrl Pts',(9.66911253341755,2.3262092647487,7.71626905499736));
#86733=CARTESIAN_POINT('Ctrl Pts',(9.60903890388976,2.56307984055212,7.72017825511565));
#86734=CARTESIAN_POINT('Ctrl Pts',(9.54032173960847,2.79743187669584,7.72408745523394));
#86735=CARTESIAN_POINT('Ctrl Pts',(9.47161205619935,3.03175840017991,7.72799622977841));
#86736=CARTESIAN_POINT('Ctrl Pts',(9.39426079570349,3.26356666257054,7.73190500432288));
#86737=CARTESIAN_POINT('Ctrl Pts',(9.3084793161308,3.49221660570547,7.73581377886735));
#86738=CARTESIAN_POINT('Ctrl Pts',(9.22269117947747,3.72088429324302,7.73972285675267));
#86739=CARTESIAN_POINT('Ctrl Pts',(9.12847161206856,3.94639290822294,7.743631934638));
#86740=CARTESIAN_POINT('Ctrl Pts',(9.02608087917656,4.16812043522776,7.74754101252332));
#86741=CARTESIAN_POINT('Ctrl Pts',(8.92369156018958,4.38984490041583,7.75145003642852));
#86742=CARTESIAN_POINT('Ctrl Pts',(8.81313142078586,4.60778812841426,7.75535906033371));
#86743=CARTESIAN_POINT('Ctrl Pts',(8.69470794663225,4.82135019706825,7.75926808423891));
#86744=CARTESIAN_POINT('Ctrl Pts',(8.57625842878933,5.03495923229034,7.76317796781661));
#86745=CARTESIAN_POINT('Ctrl Pts',(8.44994225586479,5.24418493719256,7.7670878513943));
#86746=CARTESIAN_POINT('Ctrl Pts',(8.31611243483096,5.44845280526958,7.770997734972));
#86747=CARTESIAN_POINT('Ctrl Pts',(8.2206226152689,5.59420135155263,7.77378750241291));
#86748=CARTESIAN_POINT('Ctrl Pts',(8.12130850322945,5.73742636390593,7.77657726985382));
#86749=CARTESIAN_POINT('Ctrl Pts',(8.01831179973468,5.87792819641713,7.77936703729473));
#86750=CARTESIAN_POINT('Ctrl Pts',(7.87396125947004,6.07484241544546,7.78327691424849));
#86751=CARTESIAN_POINT('Ctrl Pts',(7.72233137996099,6.2664667423681,7.78718679120226));
#86752=CARTESIAN_POINT('Ctrl Pts',(7.56383484723372,6.45226831461408,7.79109666815602));
#86753=CARTESIAN_POINT('Ctrl Pts',(7.4053657517068,6.63803772290749,7.7950058682743));
#86754=CARTESIAN_POINT('Ctrl Pts',(7.24003255766605,6.8179861755101,7.79891506839259));
#86755=CARTESIAN_POINT('Ctrl Pts',(7.06828792687707,6.99161424727965,7.80282426851087));
#86756=CARTESIAN_POINT('Ctrl Pts',(6.89656199300847,7.16522341708867,7.80673304305542));
#86757=CARTESIAN_POINT('Ctrl Pts',(6.71842621308035,7.33251338069906,7.81064181759997));
#86758=CARTESIAN_POINT('Ctrl Pts',(6.53437049287093,7.49302117052246,7.81455059214452));
#86759=CARTESIAN_POINT('Ctrl Pts',(6.35030048900216,7.65354141656613,7.81845967002984));
#86760=CARTESIAN_POINT('Ctrl Pts',(6.16030983610599,7.80727825055503,7.82236874791516));
#86761=CARTESIAN_POINT('Ctrl Pts',(5.96492291697458,7.95380780472796,7.82627782580048));
#86762=CARTESIAN_POINT('Ctrl Pts',(5.7695386959235,8.10033533548751,7.8301868497057));
#86763=CARTESIAN_POINT('Ctrl Pts',(5.56875858317553,8.23965561893869,7.83409587361092));
#86764=CARTESIAN_POINT('Ctrl Pts',(5.36313803080051,8.37138665112186,7.83800489751614));
#86765=CARTESIAN_POINT('Ctrl Pts',(5.15747225835721,8.50314665359132,7.84191478109382));
#86766=CARTESIAN_POINT('Ctrl Pts',(4.94696415479746,8.62731391767307,7.84582466467151));
#86767=CARTESIAN_POINT('Ctrl Pts',(4.73219716868203,8.74355042055101,7.8497345482492));
#86768=CARTESIAN_POINT('Ctrl Pts',(4.5789573257747,8.82648711283918,7.85252431569003));
#86769=CARTESIAN_POINT('Ctrl Pts',(4.42354984516279,8.90538712539935,7.85531408313087));
#86770=CARTESIAN_POINT('Ctrl Pts',(4.26619422686902,8.98014202664019,7.8581038505717));
#86771=CARTESIAN_POINT('Ctrl Pts',(4.04565931900907,9.08491149998974,7.86201372752548));
#86772=CARTESIAN_POINT('Ctrl Pts',(3.82122939880236,9.18156921538278,7.86592360447926));
#86773=CARTESIAN_POINT('Ctrl Pts',(3.59352066665073,9.26984213556812,7.86983348143305));
#86774=CARTESIAN_POINT('Ctrl Pts',(3.36585135296539,9.35809977490281,7.87374268155133));
#86775=CARTESIAN_POINT('Ctrl Pts',(3.13490462160849,9.43797541525348,7.87765188166961));
#86776=CARTESIAN_POINT('Ctrl Pts',(2.90131598019713,9.50924442755852,7.8815610817879));
#86777=CARTESIAN_POINT('Ctrl Pts',(2.66775276833403,9.5805056811867,7.88546985633244));
#86778=CARTESIAN_POINT('Ctrl Pts',(2.43154848868883,9.64316209580086,7.88937863087698));
#86779=CARTESIAN_POINT('Ctrl Pts',(2.1933541179885,9.69703881157041,7.89328740542152));
#86780=CARTESIAN_POINT('Ctrl Pts',(1.95514126219346,9.75091970844714,7.89719648330684));
#86781=CARTESIAN_POINT('Ctrl Pts',(1.71493827948303,9.79601948017549,7.90110556119217));
#86782=CARTESIAN_POINT('Ctrl Pts',(1.47340792594346,9.83221404790228,7.90501463907749));
#86783=CARTESIAN_POINT('Ctrl Pts',(1.23188090767481,9.86840811582155,7.90892366298271));
#86784=CARTESIAN_POINT('Ctrl Pts',(0.989026832775131,9.89569718617389,7.91283268688793));
#86785=CARTESIAN_POINT('Ctrl Pts',(0.745515925243001,9.91400877572786,7.91674171079315));
#86786=CARTESIAN_POINT('Ctrl Pts',(0.501951464795785,9.93232439236633,7.92065159437085));
#86787=CARTESIAN_POINT('Ctrl Pts',(0.257730162638098,9.94165856113522,7.92456147794855));
#86788=CARTESIAN_POINT('Ctrl Pts',(0.0135260010340399,9.94199079899474,
7.92847136152625));
#86789=CARTESIAN_POINT('Ctrl Pts',(-0.160717759787675,9.94222785627398,
7.93126112896706));
#86790=CARTESIAN_POINT('Ctrl Pts',(-0.334952715461978,9.9378830625175,7.93405089640787));
#86791=CARTESIAN_POINT('Ctrl Pts',(-0.50893420191229,9.92896520177828,7.93684066384868));
#86792=CARTESIAN_POINT('Ctrl Pts',(-0.752770370584818,9.91646676277897,
7.94075054080245));
#86793=CARTESIAN_POINT('Ctrl Pts',(-0.996183221306001,9.89497985671139,
7.94466041775621));
#86794=CARTESIAN_POINT('Ctrl Pts',(-1.23850080090203,9.86455674453571,7.94857029470998));
#86795=CARTESIAN_POINT('Ctrl Pts',(-1.48077643310591,9.83413889887937,7.95247949482824));
#86796=CARTESIAN_POINT('Ctrl Pts',(-1.72195689468176,9.79478797005676,7.9563886949465));
#86797=CARTESIAN_POINT('Ctrl Pts',(-1.96137622353292,9.74660798995013,7.96029789506476));
#86798=CARTESIAN_POINT('Ctrl Pts',(-2.20076948807947,9.69843325494082,7.96420666960927));
#86799=CARTESIAN_POINT('Ctrl Pts',(-2.43840172801783,9.64143144307598,7.96811544415377));
#86800=CARTESIAN_POINT('Ctrl Pts',(-2.67361699645525,9.57575773274709,7.97202421869828));
#86801=CARTESIAN_POINT('Ctrl Pts',(-2.90885051879443,9.51007892580408,7.97593329658358));
#86802=CARTESIAN_POINT('Ctrl Pts',(-3.14166642400791,9.43572694807743,7.97984237446888));
#86803=CARTESIAN_POINT('Ctrl Pts',(-3.37142250812632,9.35290726307597,7.98375145235419));
#86804=CARTESIAN_POINT('Ctrl Pts',(-3.60117541956527,9.27008872172351,7.98766047625941));
#86805=CARTESIAN_POINT('Ctrl Pts',(-3.82786833139425,9.17880280395587,7.99156950016463));
#86806=CARTESIAN_POINT('Ctrl Pts',(-4.05087696386306,9.07930392836607,7.99547852406986));
#86807=CARTESIAN_POINT('Ctrl Pts',(-4.27393464038622,8.97978317098538,7.99938840764754));
#86808=CARTESIAN_POINT('Ctrl Pts',(-4.49330616203895,8.87204596004266,8.00329829122523));
#86809=CARTESIAN_POINT('Ctrl Pts',(-4.70838863024301,8.75639426399921,8.00720817480292));
#86810=CARTESIAN_POINT('Ctrl Pts',(-4.86185357491026,8.67387484118349,8.00999794224383));
#86811=CARTESIAN_POINT('Ctrl Pts',(-5.01313538300588,8.58732709971643,8.01278770968474));
#86812=CARTESIAN_POINT('Ctrl Pts',(-5.16202289555346,8.49687493292575,8.01557747712564));
#86813=CARTESIAN_POINT('Ctrl Pts',(-5.3706896989147,8.37010564127491,8.01948735407942));
#86814=CARTESIAN_POINT('Ctrl Pts',(-5.57471636343669,8.23562656040008,8.0233972310332));
#86815=CARTESIAN_POINT('Ctrl Pts',(-5.77353631399771,8.09380271757039,8.02730710798698));
#86816=CARTESIAN_POINT('Ctrl Pts',(-5.97232184700733,7.95200342574468,8.03121630810531));
#86817=CARTESIAN_POINT('Ctrl Pts',(-6.16590223722477,7.80286207275889,8.03512550822363));
#86818=CARTESIAN_POINT('Ctrl Pts',(-6.35374076226922,7.64678640514292,8.03903470834196));
#86819=CARTESIAN_POINT('Ctrl Pts',(-6.54155883833198,7.49072772865519,8.04294348288645));
#86820=CARTESIAN_POINT('Ctrl Pts',(-6.72363608180163,7.32773642390535,8.04685225743094));
#86821=CARTESIAN_POINT('Ctrl Pts',(-6.89946886822186,7.15826049654784,8.05076103197544));
#86822=CARTESIAN_POINT('Ctrl Pts',(-7.07531530016244,6.98877141699464,8.05467010986075));
#86823=CARTESIAN_POINT('Ctrl Pts',(-7.24491610276115,6.81279690159378,8.05857918774607));
#86824=CARTESIAN_POINT('Ctrl Pts',(-7.40780362128749,6.63082268715127,8.06248826563139));
#86825=CARTESIAN_POINT('Ctrl Pts',(-7.57068889051531,6.44885098557368,8.06639728953661));
#86826=CARTESIAN_POINT('Ctrl Pts',(-7.72686087564606,6.26087996090083,8.07030631344184));
#86827=CARTESIAN_POINT('Ctrl Pts',(-7.87589094016651,6.06742992531459,8.07421533734707));
#86828=CARTESIAN_POINT('Ctrl Pts',(-8.02495377937637,5.87393734619963,8.07812522092477));
#86829=CARTESIAN_POINT('Ctrl Pts',(-8.1668713876149,5.67496357002263,8.08203510450247));
#86830=CARTESIAN_POINT('Ctrl Pts',(-8.30125652188631,5.47106060630295,8.08594498808017));
#86831=CARTESIAN_POINT('Ctrl Pts',(-8.39714256674417,5.32557242539756,8.08873475552099));
#86832=CARTESIAN_POINT('Ctrl Pts',(-8.48919464823231,5.17757542777426,8.09152452296181));
#86833=CARTESIAN_POINT('Ctrl Pts',(-8.57728574728243,5.02727890706948,8.09431429040262));
#86834=CARTESIAN_POINT('Ctrl Pts',(-8.70074598736116,4.81663736973718,8.09822416735638));
#86835=CARTESIAN_POINT('Ctrl Pts',(-8.81646194851285,4.60141348778399,8.10213404431014));
#86836=CARTESIAN_POINT('Ctrl Pts',(-8.92410829539135,4.3821975231757,8.1060439212639));
#86837=CARTESIAN_POINT('Ctrl Pts',(-9.03173600770174,4.16301950685775,8.10995312138216));
#86838=CARTESIAN_POINT('Ctrl Pts',(-9.13129677082162,3.93985103889644,8.11386232150042));
#86839=CARTESIAN_POINT('Ctrl Pts',(-9.2225118052798,3.71330580500376,8.11777152161869));
#86840=CARTESIAN_POINT('Ctrl Pts',(-9.31371690964388,3.48678523388193,8.12168029616319));
#86841=CARTESIAN_POINT('Ctrl Pts',(-9.3965779947819,3.25688889075372,8.1255890707077));
#86842=CARTESIAN_POINT('Ctrl Pts',(-9.47086452516024,3.02425017914547,8.1294978452522));
#86843=CARTESIAN_POINT('Ctrl Pts',(-9.54515682055158,2.79159341358864,8.13340692313752));
#86844=CARTESIAN_POINT('Ctrl Pts',(-9.61087314333275,2.5561941204022,8.13731600102283));
#86845=CARTESIAN_POINT('Ctrl Pts',(-9.66783252914784,2.31870183256729,8.14122507890814));
#86846=CARTESIAN_POINT('Ctrl Pts',(-9.7247911284166,2.08121282423906,8.1451341028134));
#86847=CARTESIAN_POINT('Ctrl Pts',(-9.77299296919053,1.84163115214548,8.14904312671865));
#86848=CARTESIAN_POINT('Ctrl Pts',(-9.8123078429667,1.60061825394256,8.15295215062391));
#86849=CARTESIAN_POINT('Ctrl Pts',(-9.85163136286887,1.3595523521895,8.1568620342016));
#86850=CARTESIAN_POINT('Ctrl Pts',(-9.88206396436873,1.11705487199665,8.16077191777929));
#86851=CARTESIAN_POINT('Ctrl Pts',(-9.90352691887924,0.873795494972577,
8.16468180135698));
#86852=CARTESIAN_POINT('Ctrl Pts',(-9.91884109652381,0.700225853773725,
8.16747156879785));
#86853=CARTESIAN_POINT('Ctrl Pts',(-9.92958984817822,0.526268498795954,
8.17026133623872));
#86854=CARTESIAN_POINT('Ctrl Pts',(-9.93576075318437,0.352167936475189,
8.1730511036796));
#86855=CARTESIAN_POINT('Ctrl Pts',(-9.93991839099059,0.234867948990494,
8.17493070522446));
#86856=CARTESIAN_POINT('Ctrl Pts',(-9.94199863950366,0.117494126326893,
8.17681030676932));
#86857=CARTESIAN_POINT('Ctrl Pts',(-9.94199999933284,0.000115177566633559,
8.17868990831418));
#86858=CARTESIAN_POINT('Origin',(0.,0.,0.));
#86859=CARTESIAN_POINT('',(-9.94203306522525,-0.000246459597145754,9.32131009168581));
#86860=CARTESIAN_POINT('',(-9.94201384449759,-0.000246996700943528,9.17868990831418));
#86861=CARTESIAN_POINT('',(-9.942,-1.2175438477123E-15,0.));
#86862=CARTESIAN_POINT('Ctrl Pts',(-9.94203306522525,-0.000246459597145754,
9.32131009168581));
#86863=CARTESIAN_POINT('Ctrl Pts',(-9.94075486143226,1.27189406067909,9.30094463654252));
#86864=CARTESIAN_POINT('Ctrl Pts',(-9.37944397540424,4.184577855052,9.25433357697359));
#86865=CARTESIAN_POINT('Ctrl Pts',(-6.60999555386334,7.97308161822977,9.18147691297896));
#86866=CARTESIAN_POINT('Ctrl Pts',(-2.03198716815049,10.1554468075767,9.102740099702));
#86867=CARTESIAN_POINT('Ctrl Pts',(3.03328101436287,9.90258945937622,9.02400328642504));
#86868=CARTESIAN_POINT('Ctrl Pts',(7.37118442122004,7.27514343098548,8.94526647314806));
#86869=CARTESIAN_POINT('Ctrl Pts',(9.94151671366969,2.90315641067999,8.86652965987108));
#86870=CARTESIAN_POINT('Ctrl Pts',(10.127925775832,-2.16499219219985,8.7877928465941));
#86871=CARTESIAN_POINT('Ctrl Pts',(7.88571169858605,-6.71398709559572,8.70905603331714));
#86872=CARTESIAN_POINT('Ctrl Pts',(3.75254558182297,-9.65300333416441,8.63031922004016));
#86873=CARTESIAN_POINT('Ctrl Pts',(-1.28046115713836,-10.2772803278934,
8.55158240676318));
#86874=CARTESIAN_POINT('Ctrl Pts',(-6.00642006970657,-8.43711974901828,
8.47284559348621));
#86875=CARTESIAN_POINT('Ctrl Pts',(-9.20947267408825,-4.67090341485341,
8.39608815690507));
#86876=CARTESIAN_POINT('Ctrl Pts',(-9.9417658544231,-1.51539093007022,8.34557632474959));
#86877=CARTESIAN_POINT('Ctrl Pts',(-9.94269874599832,0.000120372804752957,
8.32131009701976));
#86878=CARTESIAN_POINT('Ctrl Pts',(-9.94271026920365,0.000114860154877621,
8.17868991352832));
#86879=CARTESIAN_POINT('Ctrl Pts',(-9.94180931568194,-1.52162252819528,
8.20305591467107));
#86880=CARTESIAN_POINT('Ctrl Pts',(-9.20484461096283,-4.68332756624991,
8.25366752023947));
#86881=CARTESIAN_POINT('Ctrl Pts',(-5.99054191069908,-8.44840100963923,
8.33052473023354));
#86882=CARTESIAN_POINT('Ctrl Pts',(-1.26113059141423,-10.2796703076955,
8.40926154351052));
#86883=CARTESIAN_POINT('Ctrl Pts',(3.7706931866413,-9.64592892860662,8.48799835678748));
#86884=CARTESIAN_POINT('Ctrl Pts',(7.89832464265885,-6.69914470978837,8.56673517006446));
#86885=CARTESIAN_POINT('Ctrl Pts',(10.1319795417494,-2.14594095191081,8.64547198334144));
#86886=CARTESIAN_POINT('Ctrl Pts',(9.93603922976301,2.9218481185934,8.72420879661841));
#86887=CARTESIAN_POINT('Ctrl Pts',(7.35748915921657,7.28899343363155,8.80294560989537));
#86888=CARTESIAN_POINT('Ctrl Pts',(3.01465202579901,9.90827659923074,8.88168242317236));
#86889=CARTESIAN_POINT('Ctrl Pts',(-2.05108275015378,10.1516073385222,8.96041923644931));
#86890=CARTESIAN_POINT('Ctrl Pts',(-6.6249787095393,7.96063622467871,9.03915604972631));
#86891=CARTESIAN_POINT('Ctrl Pts',(-9.38351441362882,4.17212598300604,9.11191294034793));
#86892=CARTESIAN_POINT('Ctrl Pts',(-9.94074419905553,1.26566817442551,9.15842422654388));
#86893=CARTESIAN_POINT('Ctrl Pts',(-9.94201384449759,-0.000246996700943528,
9.17868990831418));
#86894=CARTESIAN_POINT('Origin',(0.,0.,0.));
#86895=CARTESIAN_POINT('',(-9.94192231880967,3.46674950698458E-5,10.321310091553));
#86896=CARTESIAN_POINT('',(-9.94192360013012,4.02297458262757E-5,10.1786899081637));
#86897=CARTESIAN_POINT('',(-9.942,-1.2175438477123E-15,0.));
#86898=CARTESIAN_POINT('Ctrl Pts',(-9.94118463298723,3.47437145860917E-5,
10.321310090292));
#86899=CARTESIAN_POINT('Ctrl Pts',(-9.94128107438378,0.7814167037778,10.3088041598135));
#86900=CARTESIAN_POINT('Ctrl Pts',(-9.65921574289398,3.20257951356252,10.2700526249096));
#86901=CARTESIAN_POINT('Ctrl Pts',(-7.71447438862192,6.91006198382807,10.2050554855795));
#86902=CARTESIAN_POINT('Ctrl Pts',(-3.50874605737789,9.74426871642388,10.1263186723027));
#86903=CARTESIAN_POINT('Ctrl Pts',(1.53836105703164,10.2418512472725,10.0475818590256));
#86904=CARTESIAN_POINT('Ctrl Pts',(6.21657731041338,8.28349191203197,9.96884504574875));
#86905=CARTESIAN_POINT('Ctrl Pts',(9.40409113980849,4.338794941827,9.8901082324717));
#86906=CARTESIAN_POINT('Ctrl Pts',(10.3365535546535,-0.646322152507229,
9.81137141919478));
#86907=CARTESIAN_POINT('Ctrl Pts',(8.79036498999971,-5.47645460637042,9.73263460591779));
#86908=CARTESIAN_POINT('Ctrl Pts',(5.13629330188293,-8.99336215383757,9.65389779264081));
#86909=CARTESIAN_POINT('Ctrl Pts',(0.250565592598979,-10.3537089295021,
9.57516097936385));
#86910=CARTESIAN_POINT('Ctrl Pts',(-4.69524642314623,-9.23129095733535,
9.49642416608685));
#86911=CARTESIAN_POINT('Ctrl Pts',(-8.51516313111776,-5.89525814222708,
9.41768735280992));
#86912=CARTESIAN_POINT('Ctrl Pts',(-9.8332983350383,-2.37409022605825,9.35931599467621));
#86913=CARTESIAN_POINT('Ctrl Pts',(-9.94240212297835,-0.36755355461397,
9.32719024096818));
#86914=CARTESIAN_POINT('Ctrl Pts',(-9.94203306522525,-0.000246459597145754,
9.32131009168581));
#86915=CARTESIAN_POINT('Ctrl Pts',(-9.94201384449759,-0.000246996700943528,
9.17868990831418));
#86916=CARTESIAN_POINT('Ctrl Pts',(-9.94238848679333,-0.373788577851782,
9.18466983096953));
#86917=CARTESIAN_POINT('Ctrl Pts',(-9.83108043390191,-2.386564907723,9.21689535805057));
#86918=CARTESIAN_POINT('Ctrl Pts',(-8.50406097389976,-5.91126204424316,
9.2753664895572));
#86919=CARTESIAN_POINT('Ctrl Pts',(-4.67787699712806,-9.24010491300058,
9.35410330283421));
#86920=CARTESIAN_POINT('Ctrl Pts',(0.270037190743816,-10.353219398773,9.43284011611116));
#86921=CARTESIAN_POINT('Ctrl Pts',(5.15319788570366,-8.98368652359915,9.51157692938814));
#86922=CARTESIAN_POINT('Ctrl Pts',(8.80064892952824,-5.45991304167992,9.59031374266511));
#86923=CARTESIAN_POINT('Ctrl Pts',(10.3377508154774,-0.626881233260456,
9.66905055594209));
#86924=CARTESIAN_POINT('Ctrl Pts',(9.39591462510088,4.35647338581691,9.74778736921906));
#86925=CARTESIAN_POINT('Ctrl Pts',(6.20098770524082,8.29516868321373,9.82652418249605));
#86926=CARTESIAN_POINT('Ctrl Pts',(1.51909666642319,10.2447263175536,9.905260995773));
#86927=CARTESIAN_POINT('Ctrl Pts',(-3.52706573424475,9.73765265912863,9.98399780904999));
#86928=CARTESIAN_POINT('Ctrl Pts',(-7.72745638993747,6.89554129457067,10.062734622327));
#86929=CARTESIAN_POINT('Ctrl Pts',(-9.66224715534303,3.19010468602984,10.1276319882147));
#86930=CARTESIAN_POINT('Ctrl Pts',(-9.94129826951133,0.775187770297893,
10.1662837496767));
#86931=CARTESIAN_POINT('Ctrl Pts',(-9.94118721097574,4.03173988009065E-5,
10.1786899067132));
#86932=CARTESIAN_POINT('Origin',(0.,0.,0.));
#86933=CARTESIAN_POINT('',(-9.94199999738095,0.000228204292448325,11.3213100916997));
#86934=CARTESIAN_POINT('',(-9.94199999743591,0.000225797020978443,11.1786899083289));
#86935=CARTESIAN_POINT('',(-9.942,-1.2175438477123E-15,0.));
#86936=CARTESIAN_POINT('Ctrl Pts',(-9.94199999738093,0.000228205157929791,
11.3213100916858));
#86937=CARTESIAN_POINT('Ctrl Pts',(-9.94199401568914,0.260826958870159,
11.3171378156917));
#86938=CARTESIAN_POINT('Ctrl Pts',(-9.93173751176087,0.52137996381255,11.3129655396974));
#86939=CARTESIAN_POINT('Ctrl Pts',(-9.91126722981454,0.781118364400918,
11.3087932637032));
#86940=CARTESIAN_POINT('Ctrl Pts',(-9.90894101982313,0.810634619437711,
11.3083191329546));
#86941=CARTESIAN_POINT('Ctrl Pts',(-9.90648296757901,0.840140358466671,
11.3078450022059));
#86942=CARTESIAN_POINT('Ctrl Pts',(-9.90389316948274,0.869634456236144,
11.3073708714572));
#86943=CARTESIAN_POINT('Ctrl Pts',(-9.88253663034234,1.11285490432175,11.3034609945034));
#86944=CARTESIAN_POINT('Ctrl Pts',(-9.85221296102367,1.35532547595535,11.2995511175496));
#86945=CARTESIAN_POINT('Ctrl Pts',(-9.81299882147288,1.59637656264802,11.2956412405958));
#86946=CARTESIAN_POINT('Ctrl Pts',(-9.77379147024857,1.83738592119121,11.2917320404775));
#86947=CARTESIAN_POINT('Ctrl Pts',(-9.72569676601436,2.07697600878047,11.2878228403592));
#86948=CARTESIAN_POINT('Ctrl Pts',(-9.66884288755413,2.31448508653521,11.2839136402409));
#86949=CARTESIAN_POINT('Ctrl Pts',(-9.61199519847276,2.55196830794197,11.2800048656963));
#86950=CARTESIAN_POINT('Ctrl Pts',(-9.54639030435697,2.78737069935341,11.2760960911518));
#86951=CARTESIAN_POINT('Ctrl Pts',(-9.47220713250327,3.02004239025783,11.2721873166073));
#86952=CARTESIAN_POINT('Ctrl Pts',(-9.3980182036574,3.25273213767116,11.268278238722));
#86953=CARTESIAN_POINT('Ctrl Pts',(-9.31524974907149,3.4826904931156,11.2643691608367));
#86954=CARTESIAN_POINT('Ctrl Pts',(-9.22413044818521,3.7092831483809,11.2604600829514));
#86955=CARTESIAN_POINT('Ctrl Pts',(-9.13301240555704,3.93587267464892,11.2565510590461));
#86956=CARTESIAN_POINT('Ctrl Pts',(-9.03354385376056,4.15909633437172,11.2526420351409));
#86957=CARTESIAN_POINT('Ctrl Pts',(-8.92600174318481,4.37833951180831,11.2487330112357));
#86958=CARTESIAN_POINT('Ctrl Pts',(-8.81843598194971,4.59763090520117,11.244823127658));
#86959=CARTESIAN_POINT('Ctrl Pts',(-8.70279323670446,4.81293981492584,11.2409132440803));
#86960=CARTESIAN_POINT('Ctrl Pts',(-8.57939719879916,5.02367472128095,11.2370033605026));
#86961=CARTESIAN_POINT('Ctrl Pts',(-8.49135205831714,5.17403760771933,11.2342135930618));
#86962=CARTESIAN_POINT('Ctrl Pts',(-8.39936064633872,5.32207232369151,11.2314238256211));
#86963=CARTESIAN_POINT('Ctrl Pts',(-8.30355445241722,5.46757235487032,11.2286340581803));
#86964=CARTESIAN_POINT('Ctrl Pts',(-8.16928145741151,5.67149158138516,11.2247241812266));
#86965=CARTESIAN_POINT('Ctrl Pts',(-8.02747249641354,5.87049339446522,11.2208143042728));
#86966=CARTESIAN_POINT('Ctrl Pts',(-7.87851295708677,6.0640248667874,11.216904427319));
#86967=CARTESIAN_POINT('Ctrl Pts',(-7.72957920401926,6.25752283704086,11.2129952272008));
#86968=CARTESIAN_POINT('Ctrl Pts',(-7.57349751450093,6.44555213487252,11.2090860270825));
#86969=CARTESIAN_POINT('Ctrl Pts',(-7.41069488170033,6.62759121931495,11.2051768269642));
#86970=CARTESIAN_POINT('Ctrl Pts',(-7.24790997235539,6.80961048613165,11.2012680524197));
#86971=CARTESIAN_POINT('Ctrl Pts',(-7.07840576743427,6.98564063277572,11.1973592778752));
#86972=CARTESIAN_POINT('Ctrl Pts',(-6.90264828910006,7.15519465821749,11.1934505033307));
#86973=CARTESIAN_POINT('Ctrl Pts',(-6.72687717108975,7.32476184191579,11.1895414254454));
#86974=CARTESIAN_POINT('Ctrl Pts',(-6.54485200959105,7.48785170332357,11.1856323475601));
#86975=CARTESIAN_POINT('Ctrl Pts',(-6.35707522503604,7.64401455932896,11.1817232696748));
#86976=CARTESIAN_POINT('Ctrl Pts',(-6.16930103347395,7.80017525889535,11.1778142457695));
#86977=CARTESIAN_POINT('Ctrl Pts',(-5.97577559455427,7.9494089667049,11.1739052218643));
#86978=CARTESIAN_POINT('Ctrl Pts',(-5.77703446244014,8.09130624928873,11.1699961979591));
#86979=CARTESIAN_POINT('Ctrl Pts',(-5.57824962317884,8.2332347379211,11.1660863143814));
#86980=CARTESIAN_POINT('Ctrl Pts',(-5.37424702639142,8.36782341366317,11.1621764308037));
#86981=CARTESIAN_POINT('Ctrl Pts',(-5.16559239746636,8.49470536176728,11.158266547226));
#86982=CARTESIAN_POINT('Ctrl Pts',(-5.01671382382033,8.5852377575856,11.1554767797851));
#86983=CARTESIAN_POINT('Ctrl Pts',(-4.86546750306949,8.67184749995319,11.1526870123442));
#86984=CARTESIAN_POINT('Ctrl Pts',(-4.71206720910581,8.75441526413214,11.1498972449033));
#86985=CARTESIAN_POINT('Ctrl Pts',(-4.49707571365825,8.87013451497527,11.1459873679495));
#86986=CARTESIAN_POINT('Ctrl Pts',(-4.27778650126964,8.97794798518521,11.1420774909958));
#86987=CARTESIAN_POINT('Ctrl Pts',(-4.05480127339336,9.07755201765804,11.138167614042));
#86988=CARTESIAN_POINT('Ctrl Pts',(-3.83185464630065,9.17713880776134,11.1342584139237));
#86989=CARTESIAN_POINT('Ctrl Pts',(-3.60521353674567,9.26851888275453,11.1303492138054));
#86990=CARTESIAN_POINT('Ctrl Pts',(-3.37550136157379,9.35143596235431,11.1264400136871));
#86991=CARTESIAN_POINT('Ctrl Pts',(-3.14581419394281,9.43434401521331,11.1225312391426));
#86992=CARTESIAN_POINT('Ctrl Pts',(-2.91305689180422,9.50879081712528,11.1186224645981));
#86993=CARTESIAN_POINT('Ctrl Pts',(-2.67787082253296,9.57456901681881,11.1147136900536));
#86994=CARTESIAN_POINT('Ctrl Pts',(-2.44266650162415,9.64035232123585,11.1108046121683));
#86995=CARTESIAN_POINT('Ctrl Pts',(-2.2050333060942,9.69746560073451,11.106895534283));
#86996=CARTESIAN_POINT('Ctrl Pts',(-1.9656269196001,9.74575162893778,11.1029864563977));
#86997=CARTESIAN_POINT('Ctrl Pts',(-1.72622383904753,9.79403699036358,11.0990774324924));
#86998=CARTESIAN_POINT('Ctrl Pts',(-1.48504789170557,9.83349529087901,11.0951684085872));
#86999=CARTESIAN_POINT('Ctrl Pts',(-1.24276481245015,9.86402045927196,11.091259384682));
#87000=CARTESIAN_POINT('Ctrl Pts',(-1.00042845030313,9.89455234075953,11.0873495011043));
#87001=CARTESIAN_POINT('Ctrl Pts',(-0.756984747826042,9.91614712852152,
11.0834396175266));
#87002=CARTESIAN_POINT('Ctrl Pts',(-0.513105806483867,9.92875049698362,
11.0795297339489));
#87003=CARTESIAN_POINT('Ctrl Pts',(-0.339094095764794,9.93774321154456,
11.0767399665081));
#87004=CARTESIAN_POINT('Ctrl Pts',(-0.164860935590121,9.94215942126182,
11.0739501990672));
#87005=CARTESIAN_POINT('Ctrl Pts',(0.00934887766037717,9.94199560442905,
11.0711604316263));
#87006=CARTESIAN_POINT('Ctrl Pts',(0.25350504780319,9.94176601408768,11.0672505546726));
#87007=CARTESIAN_POINT('Ctrl Pts',(0.497690115999459,9.93253804037882,11.0633406777188));
#87008=CARTESIAN_POINT('Ctrl Pts',(0.741230351838202,9.91433011178838,11.059430800765));
#87009=CARTESIAN_POINT('Ctrl Pts',(0.984728428633159,9.89612533515702,11.0555216006467));
#87010=CARTESIAN_POINT('Ctrl Pts',(1.22758161650919,9.86894372769043,11.0516124005284));
#87011=CARTESIAN_POINT('Ctrl Pts',(1.46911956701285,9.83285572444852,11.0477032004101));
#87012=CARTESIAN_POINT('Ctrl Pts',(1.71063122256676,9.79677164991524,11.0437944258656));
#87013=CARTESIAN_POINT('Ctrl Pts',(1.95082764951087,9.75178315697382,11.0398856513211));
#87014=CARTESIAN_POINT('Ctrl Pts',(2.18904593176937,9.69801226585139,11.0359768767766));
#87015=CARTESIAN_POINT('Ctrl Pts',(2.42728270098026,9.64423720183386,11.0320677988913));
#87016=CARTESIAN_POINT('Ctrl Pts',(2.66354074463202,9.58167843647964,11.028158721006));
#87017=CARTESIAN_POINT('Ctrl Pts',(2.89716834532257,9.51050890220186,11.0242496431207));
#87018=CARTESIAN_POINT('Ctrl Pts',(3.13079271987071,9.43934035069775,11.0203406192154));
#87019=CARTESIAN_POINT('Ctrl Pts',(3.36178645654225,9.35956135174123,11.0164315953102));
#87020=CARTESIAN_POINT('Ctrl Pts',(3.58951327945751,9.27139463169367,11.012522571405));
#87021=CARTESIAN_POINT('Ctrl Pts',(3.81729018405234,9.18320852202232,11.0086126878273));
#87022=CARTESIAN_POINT('Ctrl Pts',(4.04179847741524,9.08663110568986,11.0047028042496));
#87023=CARTESIAN_POINT('Ctrl Pts',(4.26242084838829,8.98193367328132,11.0007929206719));
#87024=CARTESIAN_POINT('Ctrl Pts',(4.41983860649652,8.90723030110401,10.998003153231));
#87025=CARTESIAN_POINT('Ctrl Pts',(4.57527841400071,8.82839399439376,10.9952133857902));
#87026=CARTESIAN_POINT('Ctrl Pts',(4.72852315291297,8.74553787896239,10.9924236183493));
#87027=CARTESIAN_POINT('Ctrl Pts',(4.94329663696212,8.6294145019885,10.9885137413956));
#87028=CARTESIAN_POINT('Ctrl Pts',(5.15382327057646,8.50535790374517,10.9846038644418));
#87029=CARTESIAN_POINT('Ctrl Pts',(5.35951885138358,8.37370417925449,10.980693987488));
#87030=CARTESIAN_POINT('Ctrl Pts',(5.56517882440315,8.2420732452284,10.9767847873697));
#87031=CARTESIAN_POINT('Ctrl Pts',(5.76600917808123,8.1028479612908,10.9728755872514));
#87032=CARTESIAN_POINT('Ctrl Pts',(5.96145337837691,7.95640858788929,10.9689663871331));
#87033=CARTESIAN_POINT('Ctrl Pts',(6.15687630170379,7.80998515656217,10.9650576125886));
#87034=CARTESIAN_POINT('Ctrl Pts',(6.34691401818147,7.65634937189688,10.9611488380441));
#87035=CARTESIAN_POINT('Ctrl Pts',(6.53104102680897,7.49592336581278,10.9572400634996));
#87036=CARTESIAN_POINT('Ctrl Pts',(6.71518232463051,7.33548490985321,10.9533309856143));
#87037=CARTESIAN_POINT('Ctrl Pts',(6.89341178465676,7.16825536135321,10.949421907729));
#87038=CARTESIAN_POINT('Ctrl Pts',(7.06523793413341,6.99469634323623,10.9455128298437));
#87039=CARTESIAN_POINT('Ctrl Pts',(7.23706171087819,6.82113972178014,10.9416038059385));
#87040=CARTESIAN_POINT('Ctrl Pts',(7.40248215815702,6.64125400617729,10.9376947820333));
#87041=CARTESIAN_POINT('Ctrl Pts',(7.56104503468376,6.45553731175678,10.933785758128));
#87042=CARTESIAN_POINT('Ctrl Pts',(7.71964278235607,6.26977977452347,10.9298758745504));
#87043=CARTESIAN_POINT('Ctrl Pts',(7.87137976295408,6.07818890873618,10.9259659909727));
#87044=CARTESIAN_POINT('Ctrl Pts',(8.01584148358403,5.88129656708904,10.922056107395));
#87045=CARTESIAN_POINT('Ctrl Pts',(8.11891734163886,5.74081058248908,10.9192663399541));
#87046=CARTESIAN_POINT('Ctrl Pts',(8.21829015114393,5.59762628955164,10.9164765725132));
#87047=CARTESIAN_POINT('Ctrl Pts',(8.31382253625065,5.45194633463416,10.9136868050724));
#87048=CARTESIAN_POINT('Ctrl Pts',(8.44771178644265,5.24777494385274,10.9097769281186));
#87049=CARTESIAN_POINT('Ctrl Pts',(8.57409681002822,5.03863783848373,10.9058670511648));
#87050=CARTESIAN_POINT('Ctrl Pts',(8.69262302131867,4.82510818627321,10.901957174211));
#87051=CARTESIAN_POINT('Ctrl Pts',(8.8111287146372,4.61161549799969,10.8980479740928));
#87052=CARTESIAN_POINT('Ctrl Pts',(8.92177817541596,4.39373202575933,10.8941387739745));
#87053=CARTESIAN_POINT('Ctrl Pts',(9.02426213795181,4.17205667093934,10.8902295738562));
#87054=CARTESIAN_POINT('Ctrl Pts',(9.12673494360457,3.95040544873441,10.8863207993117));
#87055=CARTESIAN_POINT('Ctrl Pts',(9.22104390834463,3.72496342252037,10.8824120247672));
#87056=CARTESIAN_POINT('Ctrl Pts',(9.30692695861191,3.49635161090283,10.8785032502227));
#87057=CARTESIAN_POINT('Ctrl Pts',(9.39281667384156,3.26772205784369,10.8745941723374));
#87058=CARTESIAN_POINT('Ctrl Pts',(9.47027906653661,3.03592248918386,10.870685094452));
#87059=CARTESIAN_POINT('Ctrl Pts',(9.53910076116268,2.8015925236168,10.8667760165667));
#87060=CARTESIAN_POINT('Ctrl Pts',(9.60792150543619,2.56726579389107,10.8628669926615));
#87061=CARTESIAN_POINT('Ctrl Pts',(9.66810171325942,2.33040900669161,10.8589579687563));
#87062=CARTESIAN_POINT('Ctrl Pts',(9.71947810260246,2.09167622088871,10.8550489448511));
#87063=CARTESIAN_POINT('Ctrl Pts',(9.77086579064031,1.85289093297496,10.8511390612734));
#87064=CARTESIAN_POINT('Ctrl Pts',(9.81344573149039,1.6122290960096,10.8472291776957));
#87065=CARTESIAN_POINT('Ctrl Pts',(9.84710564373104,1.37035558932723,10.843319294118));
#87066=CARTESIAN_POINT('Ctrl Pts',(9.87112255506979,1.19777478983935,10.8405295266771));
#87067=CARTESIAN_POINT('Ctrl Pts',(9.89059929140837,1.02457734830544,10.8377397592363));
#87068=CARTESIAN_POINT('Ctrl Pts',(9.90551116104081,0.851006838101755,10.8349499917954));
#87069=CARTESIAN_POINT('Ctrl Pts',(9.92641024193192,0.607746655276199,10.8310401148417));
#87070=CARTESIAN_POINT('Ctrl Pts',(9.93834719397318,0.363679016690832,10.8271302378879));
#87071=CARTESIAN_POINT('Ctrl Pts',(9.94128207593601,0.119476720215765,10.8232203609341));
#87072=CARTESIAN_POINT('Ctrl Pts',(9.9442164498439,-0.12468330260688,10.8193111608158));
#87073=CARTESIAN_POINT('Ctrl Pts',(9.9381518611066,-0.368977656633764,10.8154019606975));
#87074=CARTESIAN_POINT('Ctrl Pts',(9.92310047264189,-0.612732412929361,
10.8114927605793));
#87075=CARTESIAN_POINT('Ctrl Pts',(9.90805072274167,-0.856460632943218,
10.8075839860348));
#87076=CARTESIAN_POINT('Ctrl Pts',(9.88401614382216,-1.099649092846,10.8036752114903));
#87077=CARTESIAN_POINT('Ctrl Pts',(9.85106093362055,-1.34162680432937,10.7997664369458));
#87078=CARTESIAN_POINT('Ctrl Pts',(9.8181031659267,-1.58362329451614,10.7958573590604));
#87079=CARTESIAN_POINT('Ctrl Pts',(9.77622341841801,-1.82440857035617,10.7919482811751));
#87080=CARTESIAN_POINT('Ctrl Pts',(9.72553757910684,-2.06331839457237,10.7880392032898));
#87081=CARTESIAN_POINT('Ctrl Pts',(9.67485243971184,-2.30222491970443,10.7841301793846));
#87082=CARTESIAN_POINT('Ctrl Pts',(9.61536151191283,-2.53925577121022,10.7802211554794));
#87083=CARTESIAN_POINT('Ctrl Pts',(9.54723162710495,-2.77375778654283,10.7763121315741));
#87084=CARTESIAN_POINT('Ctrl Pts',(9.47908675917379,-3.00831137355526,10.7724022479964));
#87085=CARTESIAN_POINT('Ctrl Pts',(9.40229921522416,-3.24033474355998,10.7684923644187));
#87086=CARTESIAN_POINT('Ctrl Pts',(9.31708584979874,-3.46918942513668,10.764582480841));
#87087=CARTESIAN_POINT('Ctrl Pts',(9.25628468585954,-3.63248107478965,10.7617927134002));
#87088=CARTESIAN_POINT('Ctrl Pts',(9.19119493046871,-3.79415983268962,10.7590029459593));
#87089=CARTESIAN_POINT('Ctrl Pts',(9.12191049700365,-3.95399960605141,10.7562131785184));
#87090=CARTESIAN_POINT('Ctrl Pts',(9.02480791931507,-4.1780160731618,10.7523033015647));
#87091=CARTESIAN_POINT('Ctrl Pts',(8.91943438172357,-4.39848811357532,10.7483934246109));
#87092=CARTESIAN_POINT('Ctrl Pts',(8.80607416515645,-4.6148046326756,10.7444835476571));
#87093=CARTESIAN_POINT('Ctrl Pts',(8.69273357228029,-4.83108370540671,10.7405743475388));
#87094=CARTESIAN_POINT('Ctrl Pts',(8.57140919039356,-5.04320844466578,10.7366651474205));
#87095=CARTESIAN_POINT('Ctrl Pts',(8.4424316944315,-5.25059149857028,10.7327559473023));
#87096=CARTESIAN_POINT('Ctrl Pts',(8.31346823956229,-5.45795197578654,10.7288471727578));
#87097=CARTESIAN_POINT('Ctrl Pts',(8.17685348213841,-5.66057156039699,10.7249383982133));
#87098=CARTESIAN_POINT('Ctrl Pts',(8.03296249691575,-5.85789019384498,10.7210296236688));
#87099=CARTESIAN_POINT('Ctrl Pts',(7.88906034501943,-6.05522414022437,10.7171205457834));
#87100=CARTESIAN_POINT('Ctrl Pts',(7.73788099969172,-6.24725608511637,10.7132114678981));
#87101=CARTESIAN_POINT('Ctrl Pts',(7.5798418231581,-6.43345645325305,10.7093023900128));
#87102=CARTESIAN_POINT('Ctrl Pts',(7.42180482897308,-6.6196542501658,10.7053933661076));
#87103=CARTESIAN_POINT('Ctrl Pts',(7.25690837600702,-6.80002041898686,10.7014843422024));
#87104=CARTESIAN_POINT('Ctrl Pts',(7.0856094037922,-6.97405931842363,10.6975753182972));
#87105=CARTESIAN_POINT('Ctrl Pts',(6.91427275951001,-7.14813649249254,10.6936654347195));
#87106=CARTESIAN_POINT('Ctrl Pts',(6.73653097846631,-7.31588341617678,10.6897555511418));
#87107=CARTESIAN_POINT('Ctrl Pts',(6.55287805059349,-7.47684112804666,10.6858456675641));
#87108=CARTESIAN_POINT('Ctrl Pts',(6.42183860954114,-7.59168715223366,10.6830559001232));
#87109=CARTESIAN_POINT('Ctrl Pts',(6.28779054217795,-7.7030775137971,10.6802661326823));
#87110=CARTESIAN_POINT('Ctrl Pts',(6.15092384703256,-7.81085781639931,10.6774763652415));
#87111=CARTESIAN_POINT('Ctrl Pts',(5.9591042963248,-7.961912601483,10.6735664882877));
#87112=CARTESIAN_POINT('Ctrl Pts',(5.76168828718638,-8.10592101222527,10.6696566113339));
#87113=CARTESIAN_POINT('Ctrl Pts',(5.55921615363473,-8.24248019452681,10.6657467343802));
#87114=CARTESIAN_POINT('Ctrl Pts',(5.35677906986235,-8.37901573718415,10.6618375342619));
#87115=CARTESIAN_POINT('Ctrl Pts',(5.14928784117524,-8.50810446893057,10.6579283341436));
#87116=CARTESIAN_POINT('Ctrl Pts',(4.93731236042211,-8.62938645881751,10.6540191340253));
#87117=CARTESIAN_POINT('Ctrl Pts',(4.72535995631054,-8.7506552453802,10.6501103594808));
#87118=CARTESIAN_POINT('Ctrl Pts',(4.50892451807305,-8.86411884786377,10.6462015849363));
#87119=CARTESIAN_POINT('Ctrl Pts',(4.28860205653772,-8.96946243654883,10.6422928103918));
#87120=CARTESIAN_POINT('Ctrl Pts',(4.06826249685655,-9.07481420043323,10.6383837325065));
#87121=CARTESIAN_POINT('Ctrl Pts',(3.84403556269861,-9.17204456765895,10.6344746546212));
#87122=CARTESIAN_POINT('Ctrl Pts',(3.61654000924394,-9.26088561432101,10.6305655767359));
#87123=CARTESIAN_POINT('Ctrl Pts',(3.38904759725478,-9.3497254341851,10.6266565528307));
#87124=CARTESIAN_POINT('Ctrl Pts',(3.15828691811466,-9.43017606512544,10.6227475289255));
#87125=CARTESIAN_POINT('Ctrl Pts',(2.92489544780518,-9.50201823926941,10.6188385050203));
#87126=CARTESIAN_POINT('Ctrl Pts',(2.69145265004704,-9.57387621294324,10.6149286214426));
#87127=CARTESIAN_POINT('Ctrl Pts',(2.45537817276939,-9.6371218634826,10.6110187378649));
#87128=CARTESIAN_POINT('Ctrl Pts',(2.2173246851161,-9.69158579597657,10.6071088542872));
#87129=CARTESIAN_POINT('Ctrl Pts',(2.04746953320531,-9.73044672432767,10.6043190868463));
#87130=CARTESIAN_POINT('Ctrl Pts',(1.87660717283238,-9.76483786884059,10.6015293194054));
#87131=CARTESIAN_POINT('Ctrl Pts',(1.70497812703294,-9.79471355305193,10.5987395519645));
#87132=CARTESIAN_POINT('Ctrl Pts',(1.46443891901959,-9.83658451600917,10.5948296750108));
#87133=CARTESIAN_POINT('Ctrl Pts',(1.22231975523784,-9.86959684035226,10.590919798057));
#87134=CARTESIAN_POINT('Ctrl Pts',(0.979287453550111,-9.89365251478539,
10.5870099211032));
#87135=CARTESIAN_POINT('Ctrl Pts',(0.736297222977956,-9.91770402496113,
10.5831007209849));
#87136=CARTESIAN_POINT('Ctrl Pts',(0.492394448858487,-9.93280195273444,
10.5791915208666));
#87137=CARTESIAN_POINT('Ctrl Pts',(0.248251584657012,-9.9389000976323,10.5752823207483));
#87138=CARTESIAN_POINT('Ctrl Pts',(0.00413529898891532,-9.9449975786576,
10.5713735462038));
#87139=CARTESIAN_POINT('Ctrl Pts',(-0.240220744457244,-9.9420972260719,
10.5674647716593));
#87140=CARTESIAN_POINT('Ctrl Pts',(-0.484142519031698,-9.93020493349788,
10.5635559971148));
#87141=CARTESIAN_POINT('Ctrl Pts',(-0.72808322317909,-9.91831171802134,
10.5596469192295));
#87142=CARTESIAN_POINT('Ctrl Pts',(-0.971589310969119,-9.89742517876364,
10.5557378413442));
#87143=CARTESIAN_POINT('Ctrl Pts',(-1.21398900849319,-9.8676032899209,10.5518287634588));
#87144=CARTESIAN_POINT('Ctrl Pts',(-1.45638535874182,-9.83778181288591,
10.5479197395536));
#87145=CARTESIAN_POINT('Ctrl Pts',(-1.69767507130053,-9.79902526931551,
10.5440107156484));
#87146=CARTESIAN_POINT('Ctrl Pts',(-1.93719299711377,-9.75144334403546,
10.5401016917431));
#87147=CARTESIAN_POINT('Ctrl Pts',(-2.17676359770571,-9.70385095453909,
10.5361918081654));
#87148=CARTESIAN_POINT('Ctrl Pts',(-2.41456135771808,-9.64742935878473,
10.5322819245877));
#87149=CARTESIAN_POINT('Ctrl Pts',(-2.64993143541098,-9.58233934838569,
10.52837204101));
#87150=CARTESIAN_POINT('Ctrl Pts',(-2.81787192935261,-9.53589653541546,
10.5255822735692));
#87151=CARTESIAN_POINT('Ctrl Pts',(-2.98457669063517,-9.48504164796262,
10.5227925061284));
#87152=CARTESIAN_POINT('Ctrl Pts',(-3.14981234787036,-9.42984868241285,
10.5200027386875));
#87153=CARTESIAN_POINT('Ctrl Pts',(-3.38139118082571,-9.35249538734794,
10.5160928617338));
#87154=CARTESIAN_POINT('Ctrl Pts',(-3.61015460183394,-9.26659544417436,
10.51218298478));
#87155=CARTESIAN_POINT('Ctrl Pts',(-3.83546920859118,-9.17237918699118,
10.5082731078262));
#87156=CARTESIAN_POINT('Ctrl Pts',(-4.06074481132836,-9.07817923950419,
10.5043639077079));
#87157=CARTESIAN_POINT('Ctrl Pts',(-4.28257253311977,-8.97566595992073,
10.5004547075896));
#87158=CARTESIAN_POINT('Ctrl Pts',(-4.50033861067485,-8.86511795687283,
10.4965455074713));
#87159=CARTESIAN_POINT('Ctrl Pts',(-4.71808098119718,-8.7545819885971,10.4926367329268));
#87160=CARTESIAN_POINT('Ctrl Pts',(-4.93176234050012,-8.63601317018212,
10.4887279583823));
#87161=CARTESIAN_POINT('Ctrl Pts',(-5.14079227414487,-8.50973670533304,
10.4848191838378));
#87162=CARTESIAN_POINT('Ctrl Pts',(-5.34983842957712,-8.38345044078712,
10.4809101059525));
#87163=CARTESIAN_POINT('Ctrl Pts',(-5.5542321965262,-8.24945547690787,10.4770010280672));
#87164=CARTESIAN_POINT('Ctrl Pts',(-5.7534098701922,-8.10812178408631,10.4730919501819));
#87165=CARTESIAN_POINT('Ctrl Pts',(-5.95258479343194,-7.96679004292877,
10.4691829262767));
#87166=CARTESIAN_POINT('Ctrl Pts',(-6.14654354001739,-7.81811993941443,
10.4652739023714));
#87167=CARTESIAN_POINT('Ctrl Pts',(-6.33475278705149,-7.66252380922522,
10.4613648784662));
#87168=CARTESIAN_POINT('Ctrl Pts',(-6.52300342506034,-7.50689346033742,
10.4574549948885));
#87169=CARTESIAN_POINT('Ctrl Pts',(-6.70550182020335,-7.34433421912267,
10.4535451113108));
#87170=CARTESIAN_POINT('Ctrl Pts',(-6.88174798573715,-7.17529850673843,
10.4496352277331));
#87171=CARTESIAN_POINT('Ctrl Pts',(-7.00750257776358,-7.05468869384181,
10.4468454602923));
#87172=CARTESIAN_POINT('Ctrl Pts',(-7.13007481817835,-6.93078250798911,
10.4440556928514));
#87173=CARTESIAN_POINT('Ctrl Pts',(-7.24929444846751,-6.80375587447243,
10.4412659254105));
#87174=CARTESIAN_POINT('Ctrl Pts',(-7.41638152464334,-6.62572723322198,
10.4373560484568));
#87175=CARTESIAN_POINT('Ctrl Pts',(-7.57693294207992,-6.44151337547009,
10.433446171503));
#87176=CARTESIAN_POINT('Ctrl Pts',(-7.73050060056086,-6.25161774780961,
10.4295362945492));
#87177=CARTESIAN_POINT('Ctrl Pts',(-7.88404167507496,-6.06175499281985,
10.4256270944309));
#87178=CARTESIAN_POINT('Ctrl Pts',(-8.0306012278009,-5.86621264919321,10.4217178943126));
#87179=CARTESIAN_POINT('Ctrl Pts',(-8.16977136282007,-5.66552732578752,
10.4178086941943));
#87180=CARTESIAN_POINT('Ctrl Pts',(-8.30892634712724,-5.46486384992503,
10.4138999196498));
#87181=CARTESIAN_POINT('Ctrl Pts',(-8.44069336027146,-5.25905874245601,
10.4099911451054));
#87182=CARTESIAN_POINT('Ctrl Pts',(-8.56470717829073,-5.0486785350362,10.4060823705609));
#87183=CARTESIAN_POINT('Ctrl Pts',(-8.68873062041477,-4.83828200103931,
10.4021732926755));
#87184=CARTESIAN_POINT('Ctrl Pts',(-8.80499952012981,-4.62330989756555,
10.3982642147902));
#87185=CARTESIAN_POINT('Ctrl Pts',(-8.91319341518002,-4.40435547425404,
10.3943551369049));
#87186=CARTESIAN_POINT('Ctrl Pts',(-9.02138581619064,-4.1854040744641,10.3904461129997));
#87187=CARTESIAN_POINT('Ctrl Pts',(-9.12150331320995,-3.96247071705256,
10.3865370890944));
#87188=CARTESIAN_POINT('Ctrl Pts',(-9.21327229751492,-3.73617151263753,
10.3826280651892));
#87189=CARTESIAN_POINT('Ctrl Pts',(-9.30506146365344,-3.50982254050509,
10.3787181816115));
#87190=CARTESIAN_POINT('Ctrl Pts',(-9.38849834211504,-3.2801065017816,10.3748082980338));
#87191=CARTESIAN_POINT('Ctrl Pts',(-9.46335769533473,-3.04765895896324,
10.3708984144561));
#87192=CARTESIAN_POINT('Ctrl Pts',(-9.51677109808855,-2.88180374261834,
10.3681086470153));
#87193=CARTESIAN_POINT('Ctrl Pts',(-9.56581864139616,-2.71455830767852,
10.3653188795744));
#87194=CARTESIAN_POINT('Ctrl Pts',(-9.61043400671089,-2.54615832238587,
10.3625291121336));
#87195=CARTESIAN_POINT('Ctrl Pts',(-9.67358840539533,-2.30778305111777,
10.3585801119639));
#87196=CARTESIAN_POINT('Ctrl Pts',(-9.72787744028907,-2.06702769942914,
10.3546311117943));
#87197=CARTESIAN_POINT('Ctrl Pts',(-9.77314381814786,-1.82456129242024,
10.3506821116246));
#87198=CARTESIAN_POINT('Ctrl Pts',(-9.8184012216236,-1.58214295611016,10.3467338943725));
#87199=CARTESIAN_POINT('Ctrl Pts',(-9.85463949074573,-1.33801450552071,
10.3427856771203));
#87200=CARTESIAN_POINT('Ctrl Pts',(-9.88175247637308,-1.09285497468534,
10.3388374598682));
#87201=CARTESIAN_POINT('Ctrl Pts',(-9.90886135115302,-0.847732614725825,
10.3348898412414));
#87202=CARTESIAN_POINT('Ctrl Pts',(-9.92684767526548,-0.60157975325512,
10.3309422226145));
#87203=CARTESIAN_POINT('Ctrl Pts',(-9.93565705376861,-0.35508155386905,
10.3269946039877));
#87204=CARTESIAN_POINT('Ctrl Pts',(-9.93988551191906,-0.236763636220732,
10.3250997665537));
#87205=CARTESIAN_POINT('Ctrl Pts',(-9.9420004127048,-0.118366224562907,
10.3232049291198));
#87206=CARTESIAN_POINT('Ctrl Pts',(-9.94199999993959,3.46594688641578E-5,
10.3213100916858));
#87207=CARTESIAN_POINT('Ctrl Pts',(-9.94199999991864,4.02206518999385E-5,
10.1786899083142));
#87208=CARTESIAN_POINT('Ctrl Pts',(-9.94200099753697,-0.246557507493905,
10.1826363574975));
#87209=CARTESIAN_POINT('Ctrl Pts',(-9.9328228723075,-0.493140709085339,
10.1865828066807));
#87210=CARTESIAN_POINT('Ctrl Pts',(-9.91449490077624,-0.739022910661104,
10.190529255864));
#87211=CARTESIAN_POINT('Ctrl Pts',(-9.89616588732431,-0.984919090311048,
10.1944759293976));
#87212=CARTESIAN_POINT('Ctrl Pts',(-9.8686860119547,-1.23011392251438,10.1984226029312));
#87213=CARTESIAN_POINT('Ctrl Pts',(-9.83213649965829,-1.47392532106863,
10.2023692764648));
#87214=CARTESIAN_POINT('Ctrl Pts',(-9.79557838003627,-1.71779413664332,
10.2063168794309));
#87215=CARTESIAN_POINT('Ctrl Pts',(-9.74994639552095,-1.96027860167608,
10.210264482397));
#87216=CARTESIAN_POINT('Ctrl Pts',(-9.69537327931219,-2.20070465415039,
10.2142120853631));
#87217=CARTESIAN_POINT('Ctrl Pts',(-9.66774222224862,-2.32243539699589,
10.2162108065357));
#87218=CARTESIAN_POINT('Ctrl Pts',(-9.63781989743059,-2.44363862069704,
10.2182095277083));
#87219=CARTESIAN_POINT('Ctrl Pts',(-9.6056284949816,-2.56422799618083,10.2202082488808));
#87220=CARTESIAN_POINT('Ctrl Pts',(-9.54265601824438,-2.80012364112642,
10.2241181258346));
#87221=CARTESIAN_POINT('Ctrl Pts',(-9.47097999825955,-3.03373453810706,
10.2280280027884));
#87222=CARTESIAN_POINT('Ctrl Pts',(-9.39079139998841,-3.26441432448513,
10.2319378797422));
#87223=CARTESIAN_POINT('Ctrl Pts',(-9.31061668309735,-3.49505417808148,
10.2358470798605));
#87224=CARTESIAN_POINT('Ctrl Pts',(-9.22193242156242,-3.72276366932522,
10.2397562799788));
#87225=CARTESIAN_POINT('Ctrl Pts',(-9.12497897075438,-3.94691307014613,
10.2436654800971));
#87226=CARTESIAN_POINT('Ctrl Pts',(-9.02803607475191,-4.17103806901615,
10.2475742546416));
#87227=CARTESIAN_POINT('Ctrl Pts',(-8.92282589816911,-4.39160349413485,
10.2514830291861));
#87228=CARTESIAN_POINT('Ctrl Pts',(-8.80963673853617,-4.60800005805489,
10.2553918037306));
#87229=CARTESIAN_POINT('Ctrl Pts',(-8.69643879484802,-4.82441341545029,
10.259300881616));
#87230=CARTESIAN_POINT('Ctrl Pts',(-8.5752607580191,-5.03665701536165,10.2632099595013));
#87231=CARTESIAN_POINT('Ctrl Pts',(-8.44643724938797,-5.24414547778295,
10.2671190373867));
#87232=CARTESIAN_POINT('Ctrl Pts',(-8.31761551966884,-5.45163107501514,
10.2710280612919));
#87233=CARTESIAN_POINT('Ctrl Pts',(-8.18114867891522,-5.65436142901064,
10.2749370851971));
#87234=CARTESIAN_POINT('Ctrl Pts',(-8.03741550114447,-5.85177888013231,
10.2788461091024));
#87235=CARTESIAN_POINT('Ctrl Pts',(-7.89365071357565,-6.04923974729657,
10.2827559926801));
#87236=CARTESIAN_POINT('Ctrl Pts',(-7.7426165601319,-6.24138514960407,10.2866658762578));
#87237=CARTESIAN_POINT('Ctrl Pts',(-7.58473387359504,-6.42768823658553,
10.2905757598355));
#87238=CARTESIAN_POINT('Ctrl Pts',(-7.47208193150732,-6.56061861055974,
10.2933655272763));
#87239=CARTESIAN_POINT('Ctrl Pts',(-7.35594423870371,-6.69057526995616,
10.2961552947171));
#87240=CARTESIAN_POINT('Ctrl Pts',(-7.23648592246827,-6.81737746453272,
10.2989450621579));
#87241=CARTESIAN_POINT('Ctrl Pts',(-7.06906432640432,-6.99509155317414,
10.3028549391117));
#87242=CARTESIAN_POINT('Ctrl Pts',(-6.89506747952576,-7.16666253062903,
10.3067648160654));
#87243=CARTESIAN_POINT('Ctrl Pts',(-6.71497033289561,-7.33161219844121,
10.3106746930192));
#87244=CARTESIAN_POINT('Ctrl Pts',(-6.53490436273011,-7.49653331195598,
10.3145838931375));
#87245=CARTESIAN_POINT('Ctrl Pts',(-6.34874040747306,-7.65483521468815,
10.3184930932557));
#87246=CARTESIAN_POINT('Ctrl Pts',(-6.15698898899959,-7.80607779805824,
10.322402293374));
#87247=CARTESIAN_POINT('Ctrl Pts',(-5.96525844548086,-7.95730391645452,
10.3263110679185));
#87248=CARTESIAN_POINT('Ctrl Pts',(-5.76794187328411,-8.10147207642846,
10.330219842463));
#87249=CARTESIAN_POINT('Ctrl Pts',(-5.56558228343562,-8.23818292139156,
10.3341286170075));
#87250=CARTESIAN_POINT('Ctrl Pts',(-5.36320698945194,-8.37490437581277,
10.3380376948928));
#87251=CARTESIAN_POINT('Ctrl Pts',(-5.15578812636428,-8.50416719934732,
10.3419467727781));
#87252=CARTESIAN_POINT('Ctrl Pts',(-4.94389812404694,-8.62561507018747,
10.3458558506635));
#87253=CARTESIAN_POINT('Ctrl Pts',(-4.73201104769909,-8.74706126396518,
10.3497648745687));
#87254=CARTESIAN_POINT('Ctrl Pts',(-4.51565319984096,-8.86069258326714,
10.3536738984739));
#87255=CARTESIAN_POINT('Ctrl Pts',(-4.29542270806301,-8.96619806601754,
10.3575829223791));
#87256=CARTESIAN_POINT('Ctrl Pts',(-4.07514378319907,-9.07172675153191,
10.3614928059568));
#87257=CARTESIAN_POINT('Ctrl Pts',(-3.85099076509672,-9.16912590763516,
10.3654026895345));
#87258=CARTESIAN_POINT('Ctrl Pts',(-3.62358416969242,-9.2581316562876,10.3693125731122));
#87259=CARTESIAN_POINT('Ctrl Pts',(-3.46132575378416,-9.32163874919929,
10.3721023405531));
#87260=CARTESIAN_POINT('Ctrl Pts',(-3.29741138999951,-9.38087369123851,
10.374892107994));
#87261=CARTESIAN_POINT('Ctrl Pts',(-3.13207222452432,-9.43575580334523,
10.3776818754349));
#87262=CARTESIAN_POINT('Ctrl Pts',(-2.90034832411135,-9.51267343531538,
10.3815917523886));
#87263=CARTESIAN_POINT('Ctrl Pts',(-2.66575417575368,-9.58106267851264,
10.3855016293424));
#87264=CARTESIAN_POINT('Ctrl Pts',(-2.42893482585825,-9.64072816812781,
10.3894115062962));
#87265=CARTESIAN_POINT('Ctrl Pts',(-2.19215647155972,-9.70038332910065,
10.3933207064145));
#87266=CARTESIAN_POINT('Ctrl Pts',(-1.95315395635775,-9.75131768266605,
10.3972299065328));
#87267=CARTESIAN_POINT('Ctrl Pts',(-1.71258554818099,-9.79338627544945,
10.401139106651));
#87268=CARTESIAN_POINT('Ctrl Pts',(-1.47204332940521,-9.83545028844927,
10.4050478811955));
#87269=CARTESIAN_POINT('Ctrl Pts',(-1.22993583404403,-9.86865041952894,
10.40895665574));
#87270=CARTESIAN_POINT('Ctrl Pts',(-0.986930575442055,-9.8928930065607,
10.4128654302845));
#87271=CARTESIAN_POINT('Ctrl Pts',(-0.743906458393762,-9.91713747494075,
10.4167745081699));
#87272=CARTESIAN_POINT('Ctrl Pts',(-0.499984717526206,-9.93242297934668,
10.4206835860552));
#87273=CARTESIAN_POINT('Ctrl Pts',(-0.25583832558724,-9.93870770025765,
10.4245926639405));
#87274=CARTESIAN_POINT('Ctrl Pts',(-0.0116953050438629,-9.94499233438348,
10.4285016878457));
#87275=CARTESIAN_POINT('Ctrl Pts',(0.232672080077057,-9.94227642844191,
10.4324107117509));
#87276=CARTESIAN_POINT('Ctrl Pts',(0.476589776450805,-9.93057028498276,
10.4363197356562));
#87277=CARTESIAN_POINT('Ctrl Pts',(0.720561115200695,-9.91886156710872,
10.4402296192339));
#87278=CARTESIAN_POINT('Ctrl Pts',(0.964082287443854,-9.89815867350911,
10.4441395028116));
#87279=CARTESIAN_POINT('Ctrl Pts',(1.20648189053527,-9.8685239751348,10.4480493863892));
#87280=CARTESIAN_POINT('Ctrl Pts',(1.37943806862752,-9.84737912132989,10.4508391538301));
#87281=CARTESIAN_POINT('Ctrl Pts',(1.55182330419681,-9.82168811958619,10.453628921271));
#87282=CARTESIAN_POINT('Ctrl Pts',(1.72339585979075,-9.79148970843845,10.4564186887118));
#87283=CARTESIAN_POINT('Ctrl Pts',(1.96385589641953,-9.74916644161072,10.4603285656656));
#87284=CARTESIAN_POINT('Ctrl Pts',(2.2027929078169,-9.69797457103325,10.4642384426194));
#87285=CARTESIAN_POINT('Ctrl Pts',(2.43954643095548,-9.6380484129938,10.4681483195732));
#87286=CARTESIAN_POINT('Ctrl Pts',(2.67625896989115,-9.57813262872109,10.4720575196914));
#87287=CARTESIAN_POINT('Ctrl Pts',(2.91078850349805,-9.50948564399854,10.4759667198097));
#87288=CARTESIAN_POINT('Ctrl Pts',(3.14248686696847,-9.43229241971063,10.479875919928));
#87289=CARTESIAN_POINT('Ctrl Pts',(3.37416000667388,-9.35510759903732,10.4837846944725));
#87290=CARTESIAN_POINT('Ctrl Pts',(3.60300232580942,-9.26937848504128,10.4876934690169));
#87291=CARTESIAN_POINT('Ctrl Pts',(3.82838187488862,-9.17533956973933,10.4916022435614));
#87292=CARTESIAN_POINT('Ctrl Pts',(4.05377891456901,-9.08129335653847,10.4955113214468));
#87293=CARTESIAN_POINT('Ctrl Pts',(4.27571238733031,-8.97893615854595,10.4994203993321));
#87294=CARTESIAN_POINT('Ctrl Pts',(4.49357015286368,-8.86855068662815,10.5033294772174));
#87295=CARTESIAN_POINT('Ctrl Pts',(4.71142491001955,-8.75816673901301,10.5072385011226));
#87296=CARTESIAN_POINT('Ctrl Pts',(4.92520382337884,-8.63975486773634,10.5111475250278));
#87297=CARTESIAN_POINT('Ctrl Pts',(5.13431854831178,-8.51364416947652,10.5150565489331));
#87298=CARTESIAN_POINT('Ctrl Pts',(5.34347926175107,-8.38750573695433,10.5189664325108));
#87299=CARTESIAN_POINT('Ctrl Pts',(5.54797349649055,-8.25366523825415,10.5228763160884));
#87300=CARTESIAN_POINT('Ctrl Pts',(5.74723996198683,-8.11249633709265,10.5267861996661));
#87301=CARTESIAN_POINT('Ctrl Pts',(5.88941992373083,-8.01176996089786,10.529575967107));
#87302=CARTESIAN_POINT('Ctrl Pts',(6.02893896155573,-7.90731358197614,10.5323657345479));
#87303=CARTESIAN_POINT('Ctrl Pts',(6.16560271410765,-7.79927606716087,10.5351555019887));
#87304=CARTESIAN_POINT('Ctrl Pts',(6.35713783946976,-7.64786079751144,10.5390653789425));
#87305=CARTESIAN_POINT('Ctrl Pts',(6.5431218798354,-7.48936335350043,10.5429752558963));
#87306=CARTESIAN_POINT('Ctrl Pts',(6.72303733110427,-7.32421552417584,10.5468851328501));
#87307=CARTESIAN_POINT('Ctrl Pts',(6.90292163736157,-7.15909628345229,10.5507943329684));
#87308=CARTESIAN_POINT('Ctrl Pts',(7.0767392452124,-6.98732914501542,10.5547035330866));
#87309=CARTESIAN_POINT('Ctrl Pts',(7.2440075194695,-6.80938463136496,10.5586127332049));
#87310=CARTESIAN_POINT('Ctrl Pts',(7.41125758412091,-6.63145948958549,10.5625215077494));
#87311=CARTESIAN_POINT('Ctrl Pts',(7.57195954687699,-6.44735851951732,10.5664302822939));
#87312=CARTESIAN_POINT('Ctrl Pts',(7.72566856026041,-6.25758813737401,10.5703390568384));
#87313=CARTESIAN_POINT('Ctrl Pts',(7.87938950224671,-6.06780302808179,10.5742481347237));
#87314=CARTESIAN_POINT('Ctrl Pts',(8.02611623163984,-5.87234784346272,10.5781572126091));
#87315=CARTESIAN_POINT('Ctrl Pts',(8.1654442285848,-5.67176203219698,10.5820662904944));
#87316=CARTESIAN_POINT('Ctrl Pts',(8.30477030156209,-5.4711789908025,10.5859753143996));
#87317=CARTESIAN_POINT('Ctrl Pts',(8.43669768819625,-5.26546569586995,10.5898843383048));
#87318=CARTESIAN_POINT('Ctrl Pts',(8.560864834489,-5.05519112256002,10.5937933622101));
#87319=CARTESIAN_POINT('Ctrl Pts',(8.68505928761892,-4.84487030566871,10.5977032457878));
#87320=CARTESIAN_POINT('Ctrl Pts',(8.80148994681545,-4.62998644696003,10.6016131293655));
#87321=CARTESIAN_POINT('Ctrl Pts',(8.90984022814631,-4.41113490032959,10.6055230129432));
#87322=CARTESIAN_POINT('Ctrl Pts',(8.98714996923117,-4.25498065505952,10.6083127803841));
#87323=CARTESIAN_POINT('Ctrl Pts',(9.06034688051059,-4.09680698723904,10.6111025478249));
#87324=CARTESIAN_POINT('Ctrl Pts',(9.12933058355592,-3.93683719451928,10.6138923152658));
#87325=CARTESIAN_POINT('Ctrl Pts',(9.22601168563367,-3.71263850444416,10.6178021922195));
#87326=CARTESIAN_POINT('Ctrl Pts',(9.31444476382986,-3.48484233742335,10.6217120691733));
#87327=CARTESIAN_POINT('Ctrl Pts',(9.39437936772289,-3.25407441453056,10.6256219461271));
#87328=CARTESIAN_POINT('Ctrl Pts',(9.47430013420437,-3.02334643967738,10.6295311462454));
#87329=CARTESIAN_POINT('Ctrl Pts',(9.54572527145567,-2.7896480006273,10.6334403463637));
#87330=CARTESIAN_POINT('Ctrl Pts',(9.60845340728022,-2.55362235268355,10.6373495464819));
#87331=CARTESIAN_POINT('Ctrl Pts',(9.67117471422747,-2.31762239959221,10.6412583210265));
#87332=CARTESIAN_POINT('Ctrl Pts',(9.72520083822318,-2.07929601426984,10.645167095571));
#87333=CARTESIAN_POINT('Ctrl Pts',(9.77038070587608,-1.83930010119187,10.6490758701155));
#87334=CARTESIAN_POINT('Ctrl Pts',(9.81556407971648,-1.59928556321053,10.6529849480009));
#87335=CARTESIAN_POINT('Ctrl Pts',(9.85189977054961,-1.35760151350027,10.6568940258862));
#87336=CARTESIAN_POINT('Ctrl Pts',(9.87928788070018,-1.11491478160916,10.6608031037715));
#87337=CARTESIAN_POINT('Ctrl Pts',(9.90667561265078,-0.872231400957463,
10.6647121276767));
#87338=CARTESIAN_POINT('Ctrl Pts',(9.92511598164183,-0.628545644608861,
10.6686211515819));
#87339=CARTESIAN_POINT('Ctrl Pts',(9.93456092304684,-0.384529928966166,
10.6725301754871));
#87340=CARTESIAN_POINT('Ctrl Pts',(9.94400794158324,-0.140460549390556,
10.6764400590648));
#87341=CARTESIAN_POINT('Ctrl Pts',(9.94445556775577,0.103938654300622,10.6803499426425));
#87342=CARTESIAN_POINT('Ctrl Pts',(9.93590783939905,0.347993400754234,10.6842598262202));
#87343=CARTESIAN_POINT('Ctrl Pts',(9.92980889200356,0.52213055136565,10.6870495936611));
#87344=CARTESIAN_POINT('Ctrl Pts',(9.91913144379351,0.696092297483225,10.6898393611019));
#87345=CARTESIAN_POINT('Ctrl Pts',(9.90389316948275,0.869634456236079,10.6926291285428));
#87346=CARTESIAN_POINT('Ctrl Pts',(9.88253663034249,1.11285490432005,10.6965390054965));
#87347=CARTESIAN_POINT('Ctrl Pts',(9.85221296102409,1.35532547595203,10.7004488824503));
#87348=CARTESIAN_POINT('Ctrl Pts',(9.81299882147368,1.59637656264312,10.7043587594041));
#87349=CARTESIAN_POINT('Ctrl Pts',(9.7737914702497,1.83738592118506,10.7082679595223));
#87350=CARTESIAN_POINT('Ctrl Pts',(9.7256967660159,2.07697600877312,10.7121771596406));
#87351=CARTESIAN_POINT('Ctrl Pts',(9.66884288755617,2.31448508652667,10.7160863597589));
#87352=CARTESIAN_POINT('Ctrl Pts',(9.61199519847483,2.55196830793424,10.7199951343034));
#87353=CARTESIAN_POINT('Ctrl Pts',(9.54639030435901,2.78737069934648,10.723903908848));
#87354=CARTESIAN_POINT('Ctrl Pts',(9.47220713250522,3.0200423902517,10.7278126833925));
#87355=CARTESIAN_POINT('Ctrl Pts',(9.39801820365983,3.25273213766403,10.7317217612778));
#87356=CARTESIAN_POINT('Ctrl Pts',(9.31524974907448,3.48269049310751,10.7356308391631));
#87357=CARTESIAN_POINT('Ctrl Pts',(9.22413044818883,3.70928314837189,10.7395399170484));
#87358=CARTESIAN_POINT('Ctrl Pts',(9.13301240556115,3.93587267463934,10.7434489409537));
#87359=CARTESIAN_POINT('Ctrl Pts',(9.03354385376521,4.15909633436158,10.7473579648589));
#87360=CARTESIAN_POINT('Ctrl Pts',(8.92600174319003,4.37833951179765,10.7512669887641));
#87361=CARTESIAN_POINT('Ctrl Pts',(8.81843598195587,4.59763090518929,10.7551768723418));
#87362=CARTESIAN_POINT('Ctrl Pts',(8.70279323671164,4.81293981491277,10.7590867559195));
#87363=CARTESIAN_POINT('Ctrl Pts',(8.57939719880746,5.02367472126676,10.7629966394972));
#87364=CARTESIAN_POINT('Ctrl Pts',(8.49135205832294,5.17403760770999,10.765786406938));
#87365=CARTESIAN_POINT('Ctrl Pts',(8.39936064634176,5.32207232368689,10.7685761743789));
#87366=CARTESIAN_POINT('Ctrl Pts',(8.30355445241727,5.46757235487024,10.7713659418197));
#87367=CARTESIAN_POINT('Ctrl Pts',(8.1692814574114,5.67149158138533,10.7752758187735));
#87368=CARTESIAN_POINT('Ctrl Pts',(8.02747249641325,5.87049339446562,10.7791856957273));
#87369=CARTESIAN_POINT('Ctrl Pts',(7.87851295708629,6.06402486678801,10.783095572681));
#87370=CARTESIAN_POINT('Ctrl Pts',(7.72957920401992,6.25752283703997,10.7870047727993));
#87371=CARTESIAN_POINT('Ctrl Pts',(7.57349751450284,6.4455521348702,10.7909139729175));
#87372=CARTESIAN_POINT('Ctrl Pts',(7.4106948817036,6.62759121931129,10.7948231730358));
#87373=CARTESIAN_POINT('Ctrl Pts',(7.24790997235995,6.80961048612674,10.7987319475803));
#87374=CARTESIAN_POINT('Ctrl Pts',(7.07840576744021,6.98564063276964,10.8026407221247));
#87375=CARTESIAN_POINT('Ctrl Pts',(6.90264828910748,7.15519465821033,10.8065494966692));
#87376=CARTESIAN_POINT('Ctrl Pts',(6.72687717109729,7.32476184190886,10.8104585745545));
#87377=CARTESIAN_POINT('Ctrl Pts',(6.54485200959871,7.48785170331687,10.8143676524398));
#87378=CARTESIAN_POINT('Ctrl Pts',(6.35707522504381,7.64401455932249,10.8182767303251));
#87379=CARTESIAN_POINT('Ctrl Pts',(6.16930103348131,7.80017525888955,10.8221857542303));
#87380=CARTESIAN_POINT('Ctrl Pts',(5.97577559456118,7.94940896669972,10.8260947781355));
#87381=CARTESIAN_POINT('Ctrl Pts',(5.77703446244656,8.09130624928415,10.8300038020407));
#87382=CARTESIAN_POINT('Ctrl Pts',(5.57824962318541,8.23323473791665,10.8339136856184));
#87383=CARTESIAN_POINT('Ctrl Pts',(5.37424702639811,8.36782341365887,10.8378235691961));
#87384=CARTESIAN_POINT('Ctrl Pts',(5.16559239747318,8.49470536176313,10.8417334527738));
#87385=CARTESIAN_POINT('Ctrl Pts',(5.01671382382499,8.58523775758293,10.8445232202148));
#87386=CARTESIAN_POINT('Ctrl Pts',(4.86546750307192,8.67184749995188,10.8473129876557));
#87387=CARTESIAN_POINT('Ctrl Pts',(4.71206720910593,8.75441526413207,10.8501027550966));
#87388=CARTESIAN_POINT('Ctrl Pts',(4.49707571365821,8.8701345149753,10.8540126320504));
#87389=CARTESIAN_POINT('Ctrl Pts',(4.27778650126944,8.97794798518531,10.8579225090042));
#87390=CARTESIAN_POINT('Ctrl Pts',(4.05480127339299,9.07755201765821,10.861832385958));
#87391=CARTESIAN_POINT('Ctrl Pts',(3.83185464629978,9.17713880776172,10.8657415860763));
#87392=CARTESIAN_POINT('Ctrl Pts',(3.60521353674429,9.26851888275508,10.8696507861946));
#87393=CARTESIAN_POINT('Ctrl Pts',(3.3755013615719,9.35143596235499,10.8735599863129));
#87394=CARTESIAN_POINT('Ctrl Pts',(3.14581419394019,9.4343440152142,10.8774687608574));
#87395=CARTESIAN_POINT('Ctrl Pts',(2.91305689180085,9.50879081712634,10.8813775354019));
#87396=CARTESIAN_POINT('Ctrl Pts',(2.67787082252882,9.57456901681996,10.8852863099464));
#87397=CARTESIAN_POINT('Ctrl Pts',(2.44266650161963,9.640352321237,10.8891953878318));
#87398=CARTESIAN_POINT('Ctrl Pts',(2.2050333060893,9.69746560073563,10.8931044657171));
#87399=CARTESIAN_POINT('Ctrl Pts',(1.96562691959482,9.74575162893885,10.8970135436024));
#87400=CARTESIAN_POINT('Ctrl Pts',(1.72622383904111,9.79403699036474,10.9009225675077));
#87401=CARTESIAN_POINT('Ctrl Pts',(1.485047891698,9.83349529088018,10.9048315914129));
#87402=CARTESIAN_POINT('Ctrl Pts',(1.24276481244143,9.86402045927306,10.9087406153181));
#87403=CARTESIAN_POINT('Ctrl Pts',(1.00042845029488,9.89455234076035,10.9126504988958));
#87404=CARTESIAN_POINT('Ctrl Pts',(0.75698474781826,9.9161471285221,10.9165603824735));
#87405=CARTESIAN_POINT('Ctrl Pts',(0.513105806476577,9.928750496984,10.9204702660512));
#87406=CARTESIAN_POINT('Ctrl Pts',(0.339094095759849,9.93774321154469,10.923260033492));
#87407=CARTESIAN_POINT('Ctrl Pts',(0.164860935587527,9.94215942126182,10.9260498009328));
#87408=CARTESIAN_POINT('Ctrl Pts',(-0.00934887766062076,9.94199560442905,
10.9288395683737));
#87409=CARTESIAN_POINT('Ctrl Pts',(-0.253505047802842,9.94176601408767,
10.9327494453274));
#87410=CARTESIAN_POINT('Ctrl Pts',(-0.497690115998496,9.93253804037886,
10.9366593222812));
#87411=CARTESIAN_POINT('Ctrl Pts',(-0.741230351836662,9.9143301117885,10.940569199235));
#87412=CARTESIAN_POINT('Ctrl Pts',(-0.984728428630572,9.89612533515725,
10.9444783993532));
#87413=CARTESIAN_POINT('Ctrl Pts',(-1.22758161650558,9.86894372769085,10.9483875994715));
#87414=CARTESIAN_POINT('Ctrl Pts',(-1.46911956700822,9.83285572444921,10.9522967995898));
#87415=CARTESIAN_POINT('Ctrl Pts',(-1.71063122256193,9.79677164991608,10.9562055741343));
#87416=CARTESIAN_POINT('Ctrl Pts',(-1.95082764950584,9.75178315697482,10.9601143486788));
#87417=CARTESIAN_POINT('Ctrl Pts',(-2.18904593176416,9.69801226585256,10.9640231232233));
#87418=CARTESIAN_POINT('Ctrl Pts',(-2.42728270097545,9.64423720183507,10.9679322011086));
#87419=CARTESIAN_POINT('Ctrl Pts',(-2.66354074462762,9.58167843648087,10.971841278994));
#87420=CARTESIAN_POINT('Ctrl Pts',(-2.89716834531858,9.51050890220308,10.9757503568793));
#87421=CARTESIAN_POINT('Ctrl Pts',(-3.13079271986601,9.43934035069929,10.9796593807845));
#87422=CARTESIAN_POINT('Ctrl Pts',(-3.36178645653683,9.35956135174315,10.9835684046897));
#87423=CARTESIAN_POINT('Ctrl Pts',(-3.58951327945143,9.27139463169602,10.9874774285949));
#87424=CARTESIAN_POINT('Ctrl Pts',(-3.81729018404561,9.1832085220251,10.9913873121726));
#87425=CARTESIAN_POINT('Ctrl Pts',(-4.04179847740791,9.0866311056931,10.9952971957503));
#87426=CARTESIAN_POINT('Ctrl Pts',(-4.26242084838038,8.98193367328508,10.999207079328));
#87427=CARTESIAN_POINT('Ctrl Pts',(-4.41983860649131,8.90723030110665,11.0019968467689));
#87428=CARTESIAN_POINT('Ctrl Pts',(-4.57527841399815,8.82839399439515,11.0047866142098));
#87429=CARTESIAN_POINT('Ctrl Pts',(-4.72852315291297,8.74553787896239,11.0075763816507));
#87430=CARTESIAN_POINT('Ctrl Pts',(-4.94329663696178,8.62941450198869,11.0114862586044));
#87431=CARTESIAN_POINT('Ctrl Pts',(-5.15382327057579,8.50535790374556,11.0153961355582));
#87432=CARTESIAN_POINT('Ctrl Pts',(-5.3595188513826,8.37370417925511,11.019306012512));
#87433=CARTESIAN_POINT('Ctrl Pts',(-5.56517882440243,8.24207324522889,11.0232152126303));
#87434=CARTESIAN_POINT('Ctrl Pts',(-5.76600917808077,8.10284796129113,11.0271244127486));
#87435=CARTESIAN_POINT('Ctrl Pts',(-5.96145337837669,7.95640858788946,11.0310336128668));
#87436=CARTESIAN_POINT('Ctrl Pts',(-6.15687630170377,7.8099851565622,11.0349423874114));
#87437=CARTESIAN_POINT('Ctrl Pts',(-6.34691401818163,7.65634937189676,11.0388511619559));
#87438=CARTESIAN_POINT('Ctrl Pts',(-6.53104102680931,7.49592336581249,11.0427599365004));
#87439=CARTESIAN_POINT('Ctrl Pts',(-6.71518232463094,7.33548490985282,11.0466690143857));
#87440=CARTESIAN_POINT('Ctrl Pts',(-6.89341178465727,7.16825536135272,11.050578092271));
#87441=CARTESIAN_POINT('Ctrl Pts',(-7.065237934134,6.99469634323564,11.0544871701563));
#87442=CARTESIAN_POINT('Ctrl Pts',(-7.23706171087906,6.82113972177923,11.0583961940615));
#87443=CARTESIAN_POINT('Ctrl Pts',(-7.40248215815815,6.64125400617605,11.0623052179668));
#87444=CARTESIAN_POINT('Ctrl Pts',(-7.56104503468513,6.45553731175519,11.066214241872));
#87445=CARTESIAN_POINT('Ctrl Pts',(-7.71964278235733,6.26977977452191,11.0701241254497));
#87446=CARTESIAN_POINT('Ctrl Pts',(-7.87137976295526,6.07818890873466,11.0740340090274));
#87447=CARTESIAN_POINT('Ctrl Pts',(-8.01584148358511,5.88129656708757,11.0779438926051));
#87448=CARTESIAN_POINT('Ctrl Pts',(-8.11891734163962,5.74081058248799,11.0807336600459));
#87449=CARTESIAN_POINT('Ctrl Pts',(-8.21829015114439,5.59762628955095,11.0835234274868));
#87450=CARTESIAN_POINT('Ctrl Pts',(-8.31382253625083,5.45194633463389,11.0863131949276));
#87451=CARTESIAN_POINT('Ctrl Pts',(-8.44771178644246,5.247774943853,11.0902230718814));
#87452=CARTESIAN_POINT('Ctrl Pts',(-8.57409681002773,5.03863783848452,11.0941329488352));
#87453=CARTESIAN_POINT('Ctrl Pts',(-8.69262302131791,4.82510818627457,11.0980428257889));
#87454=CARTESIAN_POINT('Ctrl Pts',(-8.81112871463591,4.6116154980021,11.1019520259072));
#87455=CARTESIAN_POINT('Ctrl Pts',(-8.9217781754142,4.39373202576283,11.1058612260255));
#87456=CARTESIAN_POINT('Ctrl Pts',(-9.02426213794967,4.17205667094396,11.1097704261438));
#87457=CARTESIAN_POINT('Ctrl Pts',(-9.12673494360241,3.95040544873938,11.1136792006882));
#87458=CARTESIAN_POINT('Ctrl Pts',(-9.22104390834246,3.72496342252571,11.1175879752327));
#87459=CARTESIAN_POINT('Ctrl Pts',(-9.30692695860978,3.49635161090852,11.1214967497772));
#87460=CARTESIAN_POINT('Ctrl Pts',(-9.39281667383949,3.26772205784961,11.1254058276625));
#87461=CARTESIAN_POINT('Ctrl Pts',(-9.47027906653463,3.03592248919001,11.1293149055479));
#87462=CARTESIAN_POINT('Ctrl Pts',(-9.5391007611608,2.80159252362319,11.1332239834332));
#87463=CARTESIAN_POINT('Ctrl Pts',(-9.60792150543459,2.56726579389709,11.1371330073384));
#87464=CARTESIAN_POINT('Ctrl Pts',(-9.66810171325807,2.33040900669727,11.1410420312436));
#87465=CARTESIAN_POINT('Ctrl Pts',(-9.71947810260133,2.09167622089398,11.1449510551489));
#87466=CARTESIAN_POINT('Ctrl Pts',(-9.77086579063905,1.85289093298144,11.1488609387265));
#87467=CARTESIAN_POINT('Ctrl Pts',(-9.81344573148909,1.6122290960173,11.1527708223042));
#87468=CARTESIAN_POINT('Ctrl Pts',(-9.84710564372979,1.37035558933617,11.1566807058819));
#87469=CARTESIAN_POINT('Ctrl Pts',(-9.87112255506911,1.19777478984533,11.1594704733228));
#87470=CARTESIAN_POINT('Ctrl Pts',(-9.89059929140811,1.02457734830841,11.1622602407637));
#87471=CARTESIAN_POINT('Ctrl Pts',(-9.90551116104081,0.85100683810172,11.1650500082046));
#87472=CARTESIAN_POINT('Ctrl Pts',(-9.92783320511444,0.59118371235366,11.1692260983465));
#87473=CARTESIAN_POINT('Ctrl Pts',(-9.93992857739201,0.330476623162821,
11.1734021884884));
#87474=CARTESIAN_POINT('Ctrl Pts',(-9.9417559862999,0.0696556449266178,
11.1775782786304));
#87475=CARTESIAN_POINT('Ctrl Pts',(-9.94191813174516,0.046513077619066,
11.1779488218583));
#87476=CARTESIAN_POINT('Ctrl Pts',(-9.94199947180459,0.0233696156365881,
11.1783193650862));
#87477=CARTESIAN_POINT('Ctrl Pts',(-9.94199999743589,0.000225797940864191,
11.1786899083142));
#87478=CARTESIAN_POINT('Origin',(0.,0.,0.));
#87479=CARTESIAN_POINT('',(-9.94199999835375,-0.000180925794382757,12.3213100916858));
#87480=CARTESIAN_POINT('',(-9.94199999827757,-0.000185064137654065,12.1786899083142));
#87481=CARTESIAN_POINT('',(-9.942,-1.2175438477123E-15,0.));
#87482=CARTESIAN_POINT('Ctrl Pts',(-9.94199999835374,-0.000180925794382757,
12.3213100916858));
#87483=CARTESIAN_POINT('Ctrl Pts',(-9.94200442539233,0.243087966494525,
12.317414885382));
#87484=CARTESIAN_POINT('Ctrl Pts',(-9.93307575954664,0.486394731463211,
12.3135196790782));
#87485=CARTESIAN_POINT('Ctrl Pts',(-9.9152317361037,0.72907038025286,12.3096244727743));
#87486=CARTESIAN_POINT('Ctrl Pts',(-9.8973905132846,0.971707941040203,12.3057298778241));
#87487=CARTESIAN_POINT('Ctrl Pts',(-9.87063674690965,1.21371429979925,12.3018352828739));
#87488=CARTESIAN_POINT('Ctrl Pts',(-9.83504017978952,1.45442382472429,12.2979406879236));
#87489=CARTESIAN_POINT('Ctrl Pts',(-9.79944208775857,1.69514366133356,12.294045926134));
#87490=CARTESIAN_POINT('Ctrl Pts',(-9.75500047577314,1.93456627110119,12.2901511643444));
#87491=CARTESIAN_POINT('Ctrl Pts',(-9.70183671624221,2.17203322520045,12.2862564025547));
#87492=CARTESIAN_POINT('Ctrl Pts',(-9.64867488166776,2.40949158108244,12.2823617817868));
#87493=CARTESIAN_POINT('Ctrl Pts',(-9.58679159441755,2.64499414551934,12.278467161019));
#87494=CARTESIAN_POINT('Ctrl Pts',(-9.51635906541771,2.87789404565945,12.2745725402511));
#87495=CARTESIAN_POINT('Ctrl Pts',(-9.4459094703647,3.11085037827668,12.2706769758027));
#87496=CARTESIAN_POINT('Ctrl Pts',(-9.36690657469958,3.34120251339907,12.2667814113543));
#87497=CARTESIAN_POINT('Ctrl Pts',(-9.27957248525616,3.56831872047282,12.2628858469059));
#87498=CARTESIAN_POINT('Ctrl Pts',(-9.19981206165476,3.77573927066567,12.2593281081976));
#87499=CARTESIAN_POINT('Ctrl Pts',(-9.11310339949484,3.98046083360219,12.2557703694892));
#87500=CARTESIAN_POINT('Ctrl Pts',(-9.01965091992122,4.18201641349771,12.2522126307809));
#87501=CARTESIAN_POINT('Ctrl Pts',(-8.91694869074934,4.40352158330965,12.2483027538271));
#87502=CARTESIAN_POINT('Ctrl Pts',(-8.8060671984233,4.62127556763162,12.2443928768734));
#87503=CARTESIAN_POINT('Ctrl Pts',(-8.68730599303533,4.83467460987526,12.2404829999196));
#87504=CARTESIAN_POINT('Ctrl Pts',(-8.56856534629907,5.04803671079138,12.2365737998013));
#87505=CARTESIAN_POINT('Ctrl Pts',(-8.44194784569837,5.25704512973018,12.232664599683));
#87506=CARTESIAN_POINT('Ctrl Pts',(-8.30779882393879,5.4611210113823,12.2287553995648));
#87507=CARTESIAN_POINT('Ctrl Pts',(-8.17366440626839,5.66517467638062,12.2248466250203));
#87508=CARTESIAN_POINT('Ctrl Pts',(-8.03200025846291,5.8642966421205,12.2209378504758));
#87509=CARTESIAN_POINT('Ctrl Pts',(-7.88319541304502,6.05793645392108,12.2170290759313));
#87510=CARTESIAN_POINT('Ctrl Pts',(-7.73437901961274,6.25159129315795,12.213119998046));
#87511=CARTESIAN_POINT('Ctrl Pts',(-7.57842098963884,6.4397629041926,12.2092109201607));
#87512=CARTESIAN_POINT('Ctrl Pts',(-7.41575186360424,6.62193236883693,12.2053018422754));
#87513=CARTESIAN_POINT('Ctrl Pts',(-7.25308498385263,6.80409931791989,12.2013928183701));
#87514=CARTESIAN_POINT('Ctrl Pts',(-7.08370738163779,6.98026407865271,12.1974837944649));
#87515=CARTESIAN_POINT('Ctrl Pts',(-6.90808830936432,7.14994265082064,12.1935747705597));
#87516=CARTESIAN_POINT('Ctrl Pts',(-6.73243061494724,7.31965853869747,12.189664886982));
#87517=CARTESIAN_POINT('Ctrl Pts',(-6.55052890870874,7.48288519216336,12.1857550034043));
#87518=CARTESIAN_POINT('Ctrl Pts',(-6.36288855985471,7.63917621048697,12.1818451198266));
#87519=CARTESIAN_POINT('Ctrl Pts',(-6.22900402712456,7.75069247064087,12.1790553523857));
#87520=CARTESIAN_POINT('Ctrl Pts',(-6.09219867152078,7.85867854238801,12.1762655849448));
#87521=CARTESIAN_POINT('Ctrl Pts',(-5.9526663120779,7.9629848534989,12.173475817504));
#87522=CARTESIAN_POINT('Ctrl Pts',(-5.75711081576817,8.10917081723498,12.1695659405502));
#87523=CARTESIAN_POINT('Ctrl Pts',(-5.5561377292358,8.24817197377081,12.1656560635964));
#87524=CARTESIAN_POINT('Ctrl Pts',(-5.35029734095619,8.37959917677195,12.1617461866427));
#87525=CARTESIAN_POINT('Ctrl Pts',(-5.14449258553204,8.51100362852117,12.1578369865244));
#87526=CARTESIAN_POINT('Ctrl Pts',(-4.93382244647279,8.63483659325366,12.1539277864061));
#87527=CARTESIAN_POINT('Ctrl Pts',(-4.71886568293697,8.75075257714443,12.1500185862878));
#87528=CARTESIAN_POINT('Ctrl Pts',(-4.50393232059929,8.86665594187931,12.1461098117434));
#87529=CARTESIAN_POINT('Ctrl Pts',(-4.28471351218789,8.9746439136719,12.1422010371989));
#87530=CARTESIAN_POINT('Ctrl Pts',(-4.06181299303673,9.07441674211616,12.1382922626544));
#87531=CARTESIAN_POINT('Ctrl Pts',(-3.83889517566848,9.17419731344074,12.1343831847691));
#87532=CARTESIAN_POINT('Ctrl Pts',(-3.61229533124862,9.26576135016725,12.1304741068838));
#87533=CARTESIAN_POINT('Ctrl Pts',(-3.38263875336924,9.34885656453262,12.1265650289985));
#87534=CARTESIAN_POINT('Ctrl Pts',(-3.15298534679653,9.43195063144378,12.1226560050932));
#87535=CARTESIAN_POINT('Ctrl Pts',(-2.92027555549027,9.50657601644278,12.118746981188));
#87536=CARTESIAN_POINT('Ctrl Pts',(-2.68515216503208,9.57252954294859,12.1148379572828));
#87537=CARTESIAN_POINT('Ctrl Pts',(-2.4499770662418,9.63849757395284,12.1109280737051));
#87538=CARTESIAN_POINT('Ctrl Pts',(-2.21238757740481,9.69578985901981,12.1070181901274));
#87539=CARTESIAN_POINT('Ctrl Pts',(-1.97304041898176,9.74425346063331,12.1031083065497));
#87540=CARTESIAN_POINT('Ctrl Pts',(-1.80226221130059,9.77883305236884,12.1003185391088));
#87541=CARTESIAN_POINT('Ctrl Pts',(-1.63058945480415,9.80891895754833,12.0975287716679));
#87542=CARTESIAN_POINT('Ctrl Pts',(-1.45826374455853,9.8344715593318,12.094739004227));
#87543=CARTESIAN_POINT('Ctrl Pts',(-1.21674815686027,9.87028369455039,12.0908291272733));
#87544=CARTESIAN_POINT('Ctrl Pts',(-0.973875761408798,9.8972002796991,12.0869192503195));
#87545=CARTESIAN_POINT('Ctrl Pts',(-0.730315628791058,9.9151400939343,12.0830093733658));
#87546=CARTESIAN_POINT('Ctrl Pts',(-0.486797658661161,9.93307680262349,
12.0791001732475));
#87547=CARTESIAN_POINT('Ctrl Pts',(-0.24259246843857,9.942039821876,12.0751909731292));
#87548=CARTESIAN_POINT('Ctrl Pts',(0.00162653965630068,9.94199986694673,
12.0712817730109));
#87549=CARTESIAN_POINT('Ctrl Pts',(0.245818960931708,9.94195991636714,12.0673729984664));
#87550=CARTESIAN_POINT('Ctrl Pts',(0.490024916872339,9.93291894860618,12.0634642239218));
#87551=CARTESIAN_POINT('Ctrl Pts',(0.733570741879149,9.91489979609773,12.0595554493773));
#87552=CARTESIAN_POINT('Ctrl Pts',(0.977135467280196,9.89687924521144,12.055646371492));
#87553=CARTESIAN_POINT('Ctrl Pts',(1.22003967959193,9.86987913495575,12.0517372936067));
#87554=CARTESIAN_POINT('Ctrl Pts',(1.46161327421379,9.83397430526652,12.0478282157213));
#87555=CARTESIAN_POINT('Ctrl Pts',(1.70318353296792,9.79806997138381,12.0439191918161));
#87556=CARTESIAN_POINT('Ctrl Pts',(1.94342293380041,9.7532612072464,12.0400101679109));
#87557=CARTESIAN_POINT('Ctrl Pts',(2.18166929454196,9.6996743805786,12.0361011440057));
#87558=CARTESIAN_POINT('Ctrl Pts',(2.4199680504199,9.64607576909661,12.032191260428));
#87559=CARTESIAN_POINT('Ctrl Pts',(2.65627261658128,9.58369529823059,12.0282813768503));
#87560=CARTESIAN_POINT('Ctrl Pts',(2.88993239941065,9.51271016728864,12.0243714932726));
#87561=CARTESIAN_POINT('Ctrl Pts',(3.05665256931344,9.46206108704081,12.0215817258317));
#87562=CARTESIAN_POINT('Ctrl Pts',(3.22202650588926,9.40703238440347,12.0187919583909));
#87563=CARTESIAN_POINT('Ctrl Pts',(3.38582277126201,9.34770389783522,12.01600219095));
#87564=CARTESIAN_POINT('Ctrl Pts',(3.61538428729282,9.26455464355015,12.0120923139963));
#87565=CARTESIAN_POINT('Ctrl Pts',(3.8419164732703,9.1729322022759,12.0081824370425));
#87566=CARTESIAN_POINT('Ctrl Pts',(4.0647919160909,9.07308275498918,12.0042725600887));
#87567=CARTESIAN_POINT('Ctrl Pts',(4.28762877713359,8.97325059255516,12.0003633599704));
#87568=CARTESIAN_POINT('Ctrl Pts',(4.50680990297581,8.8651943816225,11.9964541598521));
#87569=CARTESIAN_POINT('Ctrl Pts',(4.72172872663316,8.74920806885327,11.9925449597338));
#87570=CARTESIAN_POINT('Ctrl Pts',(4.93662415322192,8.63323438289666,11.9886361851893));
#87571=CARTESIAN_POINT('Ctrl Pts',(5.14725795752613,8.50933245192701,11.9847274106448));
#87572=CARTESIAN_POINT('Ctrl Pts',(5.35304808513623,8.377842216121,11.9808186361003));
#87573=CARTESIAN_POINT('Ctrl Pts',(5.55885418310928,8.24634177600242,11.976909558215));
#87574=CARTESIAN_POINT('Ctrl Pts',(5.75981561540428,8.10725200268,11.9730004803296));
#87575=CARTESIAN_POINT('Ctrl Pts',(5.95537815395821,7.96095691756697,11.9690914024443));
#87576=CARTESIAN_POINT('Ctrl Pts',(6.15093799200599,7.81466385263008,11.9651823785391));
#87577=CARTESIAN_POINT('Ctrl Pts',(6.34109886218146,7.66116584446778,11.9612733546339));
#87578=CARTESIAN_POINT('Ctrl Pts',(6.52533797351644,7.50088850279647,11.9573643307287));
#87579=CARTESIAN_POINT('Ctrl Pts',(6.70961760271482,7.3405759129339,11.953454447151));
#87580=CARTESIAN_POINT('Ctrl Pts',(6.8879726586008,7.17348119376462,11.9495445635733));
#87581=CARTESIAN_POINT('Ctrl Pts',(7.05991468331884,7.00006918996227,11.9456346799956));
#87582=CARTESIAN_POINT('Ctrl Pts',(7.18259819875828,6.87633681981741,11.9428449125547));
#87583=CARTESIAN_POINT('Ctrl Pts',(7.30201751837408,6.74938910177999,11.9400551451139));
#87584=CARTESIAN_POINT('Ctrl Pts',(7.41800685906114,6.61940618476626,11.937265377673));
#87585=CARTESIAN_POINT('Ctrl Pts',(7.58056666365085,6.43723429324081,11.9333555007193));
#87586=CARTESIAN_POINT('Ctrl Pts',(7.73643741773675,6.2490434033201,11.9294456237655));
#87587=CARTESIAN_POINT('Ctrl Pts',(7.88518381604907,6.05534806490245,11.9255357468117));
#87588=CARTESIAN_POINT('Ctrl Pts',(8.03390446499868,5.86168625692037,11.9216265466935));
#87589=CARTESIAN_POINT('Ctrl Pts',(8.17550304945856,5.66252212479608,11.9177173465752));
#87590=CARTESIAN_POINT('Ctrl Pts',(8.30958528924128,5.45840235974089,11.9138081464569));
#87591=CARTESIAN_POINT('Ctrl Pts',(8.44365293220342,5.25430481611929,11.9098993719124));
#87592=CARTESIAN_POINT('Ctrl Pts',(8.57020571045967,5.0452529509567,11.905990597368));
#87593=CARTESIAN_POINT('Ctrl Pts',(8.68889275436497,4.83182229631264,11.9020818228235));
#87594=CARTESIAN_POINT('Ctrl Pts',(8.80758900899101,4.6183750783598,11.8981727449382));
#87595=CARTESIAN_POINT('Ctrl Pts',(8.91841817060669,4.4005486354097,11.8942636670529));
#87596=CARTESIAN_POINT('Ctrl Pts',(9.02107478865042,4.17894408404513,11.8903545891676));
#87597=CARTESIAN_POINT('Ctrl Pts',(9.1237299891183,3.95734259279755,11.8864455652624));
#87598=CARTESIAN_POINT('Ctrl Pts',(9.21821275575972,3.73196335270697,11.8825365413571));
#87599=CARTESIAN_POINT('Ctrl Pts',(9.30426505132221,3.50342915651852,11.8786275174519));
#87600=CARTESIAN_POINT('Ctrl Pts',(9.39033627150416,3.27484470109331,11.8747176338742));
#87601=CARTESIAN_POINT('Ctrl Pts',(9.46797321618458,3.04310416524609,11.8708077502965));
#87602=CARTESIAN_POINT('Ctrl Pts',(9.53696669288317,2.80884857171706,11.8668978667188));
#87603=CARTESIAN_POINT('Ctrl Pts',(9.58619469446056,2.64170328089288,11.8641080992779));
#87604=CARTESIAN_POINT('Ctrl Pts',(9.6310232746454,2.47327794012498,11.861318331837));
#87605=CARTESIAN_POINT('Ctrl Pts',(9.67139205901706,2.30380981002811,11.8585285643961));
#87606=CARTESIAN_POINT('Ctrl Pts',(9.7279691691198,2.06629913923054,11.8546186874423));
#87607=CARTESIAN_POINT('Ctrl Pts',(9.77580150726998,1.82666698267465,11.8507088104885));
#87608=CARTESIAN_POINT('Ctrl Pts',(9.81475025993748,1.58557287283091,11.8467989335348));
#87609=CARTESIAN_POINT('Ctrl Pts',(9.85369227021962,1.34452049858287,11.8428897334165));
#87610=CARTESIAN_POINT('Ctrl Pts',(9.88375372019248,1.10200695283348,11.8389805332982));
#87611=CARTESIAN_POINT('Ctrl Pts',(9.90484716277328,0.85870057767661,11.8350713331799));
#87612=CARTESIAN_POINT('Ctrl Pts',(9.92593830902312,0.615420689991385,11.8311625586354));
#87613=CARTESIAN_POINT('Ctrl Pts',(9.9380633730338,0.371348424390499,11.8272537840909));
#87614=CARTESIAN_POINT('Ctrl Pts',(9.94118680661349,0.127156895266496,11.8233450095465));
#87615=CARTESIAN_POINT('Ctrl Pts',(9.94431048258757,-0.117053584366446,
11.8194359316612));
#87616=CARTESIAN_POINT('Ctrl Pts',(9.9384311255953,-0.361383065752061,11.8155268537758));
#87617=CARTESIAN_POINT('Ctrl Pts',(9.92356530800884,-0.605157481721497,
11.8116177758905));
#87618=CARTESIAN_POINT('Ctrl Pts',(9.9086996957031,-0.84892853143216,11.8077087519853));
#87619=CARTESIAN_POINT('Ctrl Pts',(9.88484789010907,-1.09214425137222,11.8037997280801));
#87620=CARTESIAN_POINT('Ctrl Pts',(9.85207848366101,-1.33413400818049,11.7998907041749));
#87621=CARTESIAN_POINT('Ctrl Pts',(9.81930187056549,-1.57617698337315,11.7959808205972));
#87622=CARTESIAN_POINT('Ctrl Pts',(9.77760377452297,-1.8169931786777,11.7920709370195));
#87623=CARTESIAN_POINT('Ctrl Pts',(9.72710443168097,-2.05591910715679,11.7881610534418));
#87624=CARTESIAN_POINT('Ctrl Pts',(9.69107230447155,-2.22639676021308,11.7853712860009));
#87625=CARTESIAN_POINT('Ctrl Pts',(9.65056048832801,-2.39591221604449,11.78258151856));
#87626=CARTESIAN_POINT('Ctrl Pts',(9.60562849498159,-2.56422799618084,11.7797917511191));
#87627=CARTESIAN_POINT('Ctrl Pts',(9.54265601824462,-2.80012364112552,11.7758818741654));
#87628=CARTESIAN_POINT('Ctrl Pts',(9.4709799982601,-3.03373453810527,11.7719719972116));
#87629=CARTESIAN_POINT('Ctrl Pts',(9.39079139998933,-3.26441432448249,11.7680621202578));
#87630=CARTESIAN_POINT('Ctrl Pts',(9.310616683099,-3.49505417807695,11.7641529201396));
#87631=CARTESIAN_POINT('Ctrl Pts',(9.22193242156492,-3.72276366931889,11.7602437200213));
#87632=CARTESIAN_POINT('Ctrl Pts',(9.12497897075788,-3.94691307013804,11.756334519903));
#87633=CARTESIAN_POINT('Ctrl Pts',(9.02803607475598,-4.17103806900728,11.7524257453585));
#87634=CARTESIAN_POINT('Ctrl Pts',(8.92282589817382,-4.39160349412523,11.748516970814));
#87635=CARTESIAN_POINT('Ctrl Pts',(8.80963673854157,-4.60800005804456,11.7446081962695));
#87636=CARTESIAN_POINT('Ctrl Pts',(8.69643879485385,-4.82441341543975,11.7406991183842));
#87637=CARTESIAN_POINT('Ctrl Pts',(8.57526075802538,-5.03665701535093,11.7367900404989));
#87638=CARTESIAN_POINT('Ctrl Pts',(8.44643724939473,-5.24414547777206,11.7328809626135));
#87639=CARTESIAN_POINT('Ctrl Pts',(8.31761551967681,-5.4516310750029,11.7289719387083));
#87640=CARTESIAN_POINT('Ctrl Pts',(8.18114867892451,-5.65436142899711,11.7250629148031));
#87641=CARTESIAN_POINT('Ctrl Pts',(8.03741550115518,-5.8517788801176,11.7211538908979));
#87642=CARTESIAN_POINT('Ctrl Pts',(7.89365071358688,-6.0492397472819,11.7172440073202));
#87643=CARTESIAN_POINT('Ctrl Pts',(7.74261656014366,-6.24138514958947,11.7133341237425));
#87644=CARTESIAN_POINT('Ctrl Pts',(7.58473387360734,-6.42768823657102,11.7094242401648));
#87645=CARTESIAN_POINT('Ctrl Pts',(7.47208193151584,-6.5606186105502,11.7066344727239));
#87646=CARTESIAN_POINT('Ctrl Pts',(7.3559442387082,-6.69057526995139,11.703844705283));
#87647=CARTESIAN_POINT('Ctrl Pts',(7.23648592246849,-6.81737746453248,11.7010549378421));
#87648=CARTESIAN_POINT('Ctrl Pts',(7.06906432640483,-6.9950915531736,11.6971450608884));
#87649=CARTESIAN_POINT('Ctrl Pts',(6.89506747952659,-7.16666253062821,11.6932351839346));
#87650=CARTESIAN_POINT('Ctrl Pts',(6.71497033289678,-7.33161219844013,11.6893253069808));
#87651=CARTESIAN_POINT('Ctrl Pts',(6.53490436273144,-7.49653331195481,11.6854161068626));
#87652=CARTESIAN_POINT('Ctrl Pts',(6.34874040747457,-7.6548352146869,11.6815069067443));
#87653=CARTESIAN_POINT('Ctrl Pts',(6.15698898900126,-7.80607779805693,11.677597706626));
#87654=CARTESIAN_POINT('Ctrl Pts',(5.96525844548466,-7.95730391645159,11.6736889320816));
#87655=CARTESIAN_POINT('Ctrl Pts',(5.76794187329016,-8.10147207642406,11.6697801575371));
#87656=CARTESIAN_POINT('Ctrl Pts',(5.56558228344404,-8.23818292138587,11.6658713829927));
#87657=CARTESIAN_POINT('Ctrl Pts',(5.36320698946049,-8.3749043758073,11.6619623051073));
#87658=CARTESIAN_POINT('Ctrl Pts',(5.15578812637295,-8.50416719934206,11.658053227222));
#87659=CARTESIAN_POINT('Ctrl Pts',(4.94389812405574,-8.62561507018243,11.6541441493367));
#87660=CARTESIAN_POINT('Ctrl Pts',(4.73201104770847,-8.74706126396009,11.6502351254315));
#87661=CARTESIAN_POINT('Ctrl Pts',(4.51565319985091,-8.86069258326205,11.6463261015263));
#87662=CARTESIAN_POINT('Ctrl Pts',(4.29542270807355,-8.96619806601249,11.6424170776211));
#87663=CARTESIAN_POINT('Ctrl Pts',(4.07514378320925,-9.07172675152735,11.6385071940434));
#87664=CARTESIAN_POINT('Ctrl Pts',(3.85099076510653,-9.16912590763106,11.6345973104657));
#87665=CARTESIAN_POINT('Ctrl Pts',(3.62358416970183,-9.25813165628391,11.630687426888));
#87666=CARTESIAN_POINT('Ctrl Pts',(3.46132575379055,-9.32163874919698,11.627897659447));
#87667=CARTESIAN_POINT('Ctrl Pts',(3.29741139000283,-9.3808736912374,11.6251078920061));
#87668=CARTESIAN_POINT('Ctrl Pts',(3.13207222452451,-9.43575580334517,11.6223181245651));
#87669=CARTESIAN_POINT('Ctrl Pts',(2.90034832411118,-9.51267343531544,11.6184082476114));
#87670=CARTESIAN_POINT('Ctrl Pts',(2.66575417575317,-9.58106267851279,11.6144983706576));
#87671=CARTESIAN_POINT('Ctrl Pts',(2.42893482585738,-9.64072816812803,11.6105884937038));
#87672=CARTESIAN_POINT('Ctrl Pts',(2.19215647155919,-9.70038332910076,11.6066792935855));
#87673=CARTESIAN_POINT('Ctrl Pts',(1.95315395635757,-9.75131768266608,11.6027700934672));
#87674=CARTESIAN_POINT('Ctrl Pts',(1.71258554818117,-9.79338627544942,11.5988608933489));
#87675=CARTESIAN_POINT('Ctrl Pts',(1.47204332940585,-9.83545028844916,11.5949521188044));
#87676=CARTESIAN_POINT('Ctrl Pts',(1.22993583404512,-9.86865041952879,11.59104334426));
#87677=CARTESIAN_POINT('Ctrl Pts',(0.986930575443621,-9.89289300656054,
11.5871345697155));
#87678=CARTESIAN_POINT('Ctrl Pts',(0.743906458394857,-9.91713747494068,
11.5832254918301));
#87679=CARTESIAN_POINT('Ctrl Pts',(0.499984717526834,-9.93242297934666,
11.5793164139448));
#87680=CARTESIAN_POINT('Ctrl Pts',(0.255838325587391,-9.93870770025765,
11.5754073360595));
#87681=CARTESIAN_POINT('Ctrl Pts',(0.0116953050447619,-9.94499233438346,
11.5714983121543));
#87682=CARTESIAN_POINT('Ctrl Pts',(-0.23267208007543,-9.94227642844193,
11.5675892882491));
#87683=CARTESIAN_POINT('Ctrl Pts',(-0.47658977644844,-9.93057028498287,
11.5636802643439));
#87684=CARTESIAN_POINT('Ctrl Pts',(-0.720561115199568,-9.91886156710883,
11.5597703807662));
#87685=CARTESIAN_POINT('Ctrl Pts',(-0.964082287443942,-9.89815867350913,
11.5558604971884));
#87686=CARTESIAN_POINT('Ctrl Pts',(-1.20648189053658,-9.86852397513464,
11.5519506136107));
#87687=CARTESIAN_POINT('Ctrl Pts',(-1.37943806862841,-9.84737912132976,
11.5491608461699));
#87688=CARTESIAN_POINT('Ctrl Pts',(-1.55182330419729,-9.82168811958611,
11.546371078729));
#87689=CARTESIAN_POINT('Ctrl Pts',(-1.72339585979082,-9.79148970843844,
11.5435813112882));
#87690=CARTESIAN_POINT('Ctrl Pts',(-1.96385589641977,-9.74916644161068,
11.5396714343344));
#87691=CARTESIAN_POINT('Ctrl Pts',(-2.20279290781731,-9.69797457103316,
11.5357615573806));
#87692=CARTESIAN_POINT('Ctrl Pts',(-2.43954643095606,-9.63804841299366,
11.5318516804268));
#87693=CARTESIAN_POINT('Ctrl Pts',(-2.67625896989279,-9.57813262872066,
11.5279424803086));
#87694=CARTESIAN_POINT('Ctrl Pts',(-2.91078850350073,-9.50948564399775,
11.5240332801903));
#87695=CARTESIAN_POINT('Ctrl Pts',(-3.14248686697217,-9.4322924197094,11.520124080072));
#87696=CARTESIAN_POINT('Ctrl Pts',(-3.37416000667744,-9.35510759903604,
11.5162153055275));
#87697=CARTESIAN_POINT('Ctrl Pts',(-3.60300232581281,-9.26937848503996,
11.512306530983));
#87698=CARTESIAN_POINT('Ctrl Pts',(-3.82838187489187,-9.17533956973797,
11.5083977564385));
#87699=CARTESIAN_POINT('Ctrl Pts',(-4.05377891457193,-9.08129335653716,
11.5044886785532));
#87700=CARTESIAN_POINT('Ctrl Pts',(-4.27571238733293,-8.97893615854469,
11.5005796006679));
#87701=CARTESIAN_POINT('Ctrl Pts',(-4.493570152866,-8.86855068662698,11.4966705227826));
#87702=CARTESIAN_POINT('Ctrl Pts',(-4.71142491002214,-8.75816673901163,
11.4927614988773));
#87703=CARTESIAN_POINT('Ctrl Pts',(-4.92520382338169,-8.63975486773473,
11.4888524749721));
#87704=CARTESIAN_POINT('Ctrl Pts',(-5.13431854831489,-8.51364416947465,
11.4849434510669));
#87705=CARTESIAN_POINT('Ctrl Pts',(-5.34347926175485,-8.38750573695195,
11.4810335674892));
#87706=CARTESIAN_POINT('Ctrl Pts',(-5.54797349649497,-8.25366523825121,
11.4771236839115));
#87707=CARTESIAN_POINT('Ctrl Pts',(-5.74723996199185,-8.11249633708909,
11.4732138003338));
#87708=CARTESIAN_POINT('Ctrl Pts',(-5.88941992373415,-8.01176996089537,
11.4704240328929));
#87709=CARTESIAN_POINT('Ctrl Pts',(-6.02893896155739,-7.90731358197483,
11.4676342654521));
#87710=CARTESIAN_POINT('Ctrl Pts',(-6.16560271410774,-7.7992760671608,11.4648444980112));
#87711=CARTESIAN_POINT('Ctrl Pts',(-6.35713783946964,-7.64786079751152,
11.4609346210575));
#87712=CARTESIAN_POINT('Ctrl Pts',(-6.5431218798351,-7.48936335350068,11.4570247441037));
#87713=CARTESIAN_POINT('Ctrl Pts',(-6.72303733110379,-7.32421552417628,
11.4531148671499));
#87714=CARTESIAN_POINT('Ctrl Pts',(-6.90292163736225,-7.15909628345168,
11.4492056670316));
#87715=CARTESIAN_POINT('Ctrl Pts',(-7.07673924521416,-6.98732914501369,
11.4452964669133));
#87716=CARTESIAN_POINT('Ctrl Pts',(-7.24400751947226,-6.80938463136203,
11.441387266795));
#87717=CARTESIAN_POINT('Ctrl Pts',(-7.41125758412094,-6.63145948958531,
11.4374784922506));
#87718=CARTESIAN_POINT('Ctrl Pts',(-7.57195954687448,-6.44735851952012,
11.4335697177061));
#87719=CARTESIAN_POINT('Ctrl Pts',(-7.7256685602556,-6.25758813737994,11.4296609431617));
#87720=CARTESIAN_POINT('Ctrl Pts',(-7.87938950224148,-6.06780302808854,
11.4257518652764));
#87721=CARTESIAN_POINT('Ctrl Pts',(-8.02611623163426,-5.87234784347031,
11.4218427873911));
#87722=CARTESIAN_POINT('Ctrl Pts',(-8.16544422857891,-5.67176203220546,
11.4179337095058));
#87723=CARTESIAN_POINT('Ctrl Pts',(-8.30477030155618,-5.47117899081146,
11.4140246856006));
#87724=CARTESIAN_POINT('Ctrl Pts',(-8.43669768819032,-5.26546569587943,
11.4101156616953));
#87725=CARTESIAN_POINT('Ctrl Pts',(-8.56086483448311,-5.05519112256999,
11.4062066377901));
#87726=CARTESIAN_POINT('Ctrl Pts',(-8.68505928761271,-4.84487030567978,
11.4022967542124));
#87727=CARTESIAN_POINT('Ctrl Pts',(-8.80148994680901,-4.62998644697222,
11.3983868706347));
#87728=CARTESIAN_POINT('Ctrl Pts',(-8.9098402281397,-4.41113490034294,11.394476987057));
#87729=CARTESIAN_POINT('Ctrl Pts',(-8.98714996922696,-4.2549806550686,11.3916872196161));
#87730=CARTESIAN_POINT('Ctrl Pts',(-9.06034688050858,-4.09680698724369,
11.3888974521752));
#87731=CARTESIAN_POINT('Ctrl Pts',(-9.12933058355585,-3.93683719451945,
11.3861076847342));
#87732=CARTESIAN_POINT('Ctrl Pts',(-9.22562982053677,-3.71352403070184,
11.382213250773));
#87733=CARTESIAN_POINT('Ctrl Pts',(-9.31374835312292,-3.48663634832032,
11.3783188168118));
#87734=CARTESIAN_POINT('Ctrl Pts',(-9.39343666062907,-3.25679469766667,
11.3744243828506));
#87735=CARTESIAN_POINT('Ctrl Pts',(-9.47311002949082,-3.02699613391994,
11.3705306789534));
#87736=CARTESIAN_POINT('Ctrl Pts',(-9.5443562345871,-2.79424497617588,11.3666369750562));
#87737=CARTESIAN_POINT('Ctrl Pts',(-9.60697480470969,-2.55917938051893,
11.362743271159));
#87738=CARTESIAN_POINT('Ctrl Pts',(-9.6695917581785,-2.32411985366366,11.3588496677875));
#87739=CARTESIAN_POINT('Ctrl Pts',(-9.72358144507331,-2.0867462825211,11.3549560644159));
#87740=CARTESIAN_POINT('Ctrl Pts',(-9.76879364488237,-1.84771067099419,
11.3510624610443));
#87741=CARTESIAN_POINT('Ctrl Pts',(-9.81400323699699,-1.60868884627345,
11.3471690822433));
#87742=CARTESIAN_POINT('Ctrl Pts',(-9.85043630164515,-1.36800545269013,
11.3432757034422));
#87743=CARTESIAN_POINT('Ctrl Pts',(-9.87799384897245,-1.12632212073742,
11.3393823246412));
#87744=CARTESIAN_POINT('Ctrl Pts',(-9.90555545351527,-0.884603206468445,
11.3354883726296));
#87745=CARTESIAN_POINT('Ctrl Pts',(-9.92423889681383,-0.641884342588685,
11.331594420618));
#87746=CARTESIAN_POINT('Ctrl Pts',(-9.93399699326778,-0.398832969733717,
11.3277004686064));
#87747=CARTESIAN_POINT('Ctrl Pts',(-9.93933500753949,-0.265875511977494,
11.3255703429709));
#87748=CARTESIAN_POINT('Ctrl Pts',(-9.94200305127928,-0.132818623544602,
11.3234402173353));
#87749=CARTESIAN_POINT('Ctrl Pts',(-9.94199999738095,0.000228204292474588,
11.3213100916997));
#87750=CARTESIAN_POINT('Ctrl Pts',(-9.94199999743591,0.000225797020946319,
11.1786899083289));
#87751=CARTESIAN_POINT('Ctrl Pts',(-9.94200552108102,-0.242984141546804,
11.1825838119575));
#87752=CARTESIAN_POINT('Ctrl Pts',(-9.93308227899852,-0.486228017217286,
11.1864777155862));
#87753=CARTESIAN_POINT('Ctrl Pts',(-9.91524887911624,-0.728837200741169,
11.1903716192148));
#87754=CARTESIAN_POINT('Ctrl Pts',(-9.89741786708007,-0.971413899522894,
11.1942650014598));
#87755=CARTESIAN_POINT('Ctrl Pts',(-9.87067909983736,-1.21335579191454,
11.1981583837048));
#87756=CARTESIAN_POINT('Ctrl Pts',(-9.83510318760652,-1.45399769227194,
11.2020517659498));
#87757=CARTESIAN_POINT('Ctrl Pts',(-9.7995252600358,-1.69465322475247,11.205945368751));
#87758=CARTESIAN_POINT('Ctrl Pts',(-9.75510922572029,-1.93400833586019,
11.2098389715522));
#87759=CARTESIAN_POINT('Ctrl Pts',(-9.7019773071014,-2.17140515162176,11.2137325743534));
#87760=CARTESIAN_POINT('Ctrl Pts',(-9.6488460243958,-2.408799126082,11.2176261305538));
#87761=CARTESIAN_POINT('Ctrl Pts',(-9.58699913029883,-2.64423457461387,
11.2215196867541));
#87762=CARTESIAN_POINT('Ctrl Pts',(-9.51660966073042,-2.87706526955722,
11.2254132429544));
#87763=CARTESIAN_POINT('Ctrl Pts',(-9.44620464128667,-3.10994739958461,
11.2293076592879));
#87764=CARTESIAN_POINT('Ctrl Pts',(-9.36725335772919,-3.34022335347587,
11.2332020756213));
#87765=CARTESIAN_POINT('Ctrl Pts',(-9.27997867577238,-3.56726222434095,
11.2370964919548));
#87766=CARTESIAN_POINT('Ctrl Pts',(-9.23000144926437,-3.69727442055797,
11.239326601797));
#87767=CARTESIAN_POINT('Ctrl Pts',(-9.17729572185186,-3.82622542439781,
11.2415567116393));
#87768=CARTESIAN_POINT('Ctrl Pts',(-9.12191049700363,-3.95399960605144,
11.2437868214816));
#87769=CARTESIAN_POINT('Ctrl Pts',(-9.0248079193148,-4.17801607316244,11.2476966984354));
#87770=CARTESIAN_POINT('Ctrl Pts',(-8.91943438172299,-4.39848811357653,
11.2516065753892));
#87771=CARTESIAN_POINT('Ctrl Pts',(-8.80607416515553,-4.61480463267736,
11.2555164523429));
#87772=CARTESIAN_POINT('Ctrl Pts',(-8.69273357227901,-4.83108370540904,
11.2594256524612));
#87773=CARTESIAN_POINT('Ctrl Pts',(-8.57140919039189,-5.04320844466865,
11.2633348525795));
#87774=CARTESIAN_POINT('Ctrl Pts',(-8.44243169442939,-5.25059149857366,
11.2672440526978));
#87775=CARTESIAN_POINT('Ctrl Pts',(-8.31346823956048,-5.45795197578927,
11.2711528272423));
#87776=CARTESIAN_POINT('Ctrl Pts',(-8.17685348213692,-5.6605715603991,11.2750616017868));
#87777=CARTESIAN_POINT('Ctrl Pts',(-8.03296249691464,-5.8578901938465,11.2789703763313));
#87778=CARTESIAN_POINT('Ctrl Pts',(-7.88906034501808,-6.05522414022614,
11.2828794542166));
#87779=CARTESIAN_POINT('Ctrl Pts',(-7.7378809996901,-6.24725608511839,11.2867885321019));
#87780=CARTESIAN_POINT('Ctrl Pts',(-7.57984182315619,-6.43345645325529,
11.2906976099872));
#87781=CARTESIAN_POINT('Ctrl Pts',(-7.42180482897088,-6.61965425016828,
11.2946066338925));
#87782=CARTESIAN_POINT('Ctrl Pts',(-7.25690837600449,-6.80002041898957,
11.2985156577977));
#87783=CARTESIAN_POINT('Ctrl Pts',(-7.08560940378933,-6.97405931842655,
11.3024246817029));
#87784=CARTESIAN_POINT('Ctrl Pts',(-6.91427275950652,-7.14813649249594,
11.3063345652806));
#87785=CARTESIAN_POINT('Ctrl Pts',(-6.73653097846217,-7.31588341618062,
11.3102444488583));
#87786=CARTESIAN_POINT('Ctrl Pts',(-6.55287805058865,-7.4768411280509,11.314154332436));
#87787=CARTESIAN_POINT('Ctrl Pts',(-6.42183860953779,-7.59168715223645,
11.3169440998769));
#87788=CARTESIAN_POINT('Ctrl Pts',(-6.28779054217615,-7.70307751379853,
11.3197338673177));
#87789=CARTESIAN_POINT('Ctrl Pts',(-6.15092384703237,-7.81085781639946,
11.3225236347586));
#87790=CARTESIAN_POINT('Ctrl Pts',(-5.95910429632489,-7.96191260148291,
11.3264335117123));
#87791=CARTESIAN_POINT('Ctrl Pts',(-5.76168828718676,-8.10592101222499,
11.3303433886661));
#87792=CARTESIAN_POINT('Ctrl Pts',(-5.55921615363541,-8.24248019452635,
11.3342532656199));
#87793=CARTESIAN_POINT('Ctrl Pts',(-5.35677906986329,-8.37901573718354,
11.3381624657381));
#87794=CARTESIAN_POINT('Ctrl Pts',(-5.14928784117645,-8.50810446892983,
11.3420716658564));
#87795=CARTESIAN_POINT('Ctrl Pts',(-4.93731236042359,-8.62938645881667,
11.3459808659747));
#87796=CARTESIAN_POINT('Ctrl Pts',(-4.72535995631246,-8.75065524537915,
11.3498896405192));
#87797=CARTESIAN_POINT('Ctrl Pts',(-4.50892451807544,-8.86411884786254,
11.3537984150637));
#87798=CARTESIAN_POINT('Ctrl Pts',(-4.28860205654056,-8.96946243654747,
11.3577071896082));
#87799=CARTESIAN_POINT('Ctrl Pts',(-4.06826249685949,-9.07481420043191,
11.3616162674935));
#87800=CARTESIAN_POINT('Ctrl Pts',(-3.84403556270164,-9.17204456765768,
11.3655253453788));
#87801=CARTESIAN_POINT('Ctrl Pts',(-3.61654000924706,-9.26088561431979,
11.3694344232641));
#87802=CARTESIAN_POINT('Ctrl Pts',(-3.38904759725678,-9.34972543418441,
11.3733434471694));
#87803=CARTESIAN_POINT('Ctrl Pts',(-3.15828691811552,-9.43017606512519,
11.3772524710746));
#87804=CARTESIAN_POINT('Ctrl Pts',(-2.92489544780486,-9.50201823926951,
11.3811614949798));
#87805=CARTESIAN_POINT('Ctrl Pts',(-2.69145265004682,-9.5738762129433,11.3850713785575));
#87806=CARTESIAN_POINT('Ctrl Pts',(-2.45537817276924,-9.63712186348263,
11.3889812621352));
#87807=CARTESIAN_POINT('Ctrl Pts',(-2.21732468511605,-9.69158579597658,
11.3928911457129));
#87808=CARTESIAN_POINT('Ctrl Pts',(-2.04746953320517,-9.7304467243277,11.3956809131538));
#87809=CARTESIAN_POINT('Ctrl Pts',(-1.87660717283218,-9.76483786884063,
11.3984706805947));
#87810=CARTESIAN_POINT('Ctrl Pts',(-1.70497812703265,-9.79471355305198,
11.4012604480355));
#87811=CARTESIAN_POINT('Ctrl Pts',(-1.46443891901957,-9.83658451600917,
11.4051703249893));
#87812=CARTESIAN_POINT('Ctrl Pts',(-1.22231975523809,-9.86959684035222,
11.4090802019431));
#87813=CARTESIAN_POINT('Ctrl Pts',(-0.979287453550639,-9.89365251478534,
11.4129900788969));
#87814=CARTESIAN_POINT('Ctrl Pts',(-0.736297222978803,-9.91770402496106,
11.4168992790151));
#87815=CARTESIAN_POINT('Ctrl Pts',(-0.49239444885965,-9.93280195273437,
11.4208084791334));
#87816=CARTESIAN_POINT('Ctrl Pts',(-0.248251584658489,-9.93890009763226,
11.4247176792517));
#87817=CARTESIAN_POINT('Ctrl Pts',(-0.00413529899127343,-9.94499757865758,
11.4286264537962));
#87818=CARTESIAN_POINT('Ctrl Pts',(0.240220744454,-9.94209722607196,11.4325352283407));
#87819=CARTESIAN_POINT('Ctrl Pts',(0.484142519027582,-9.93020493349808,
11.4364440028852));
#87820=CARTESIAN_POINT('Ctrl Pts',(0.728083223174456,-9.91831171802167,
11.4403530807705));
#87821=CARTESIAN_POINT('Ctrl Pts',(0.971589310963972,-9.89742517876413,
11.4442621586558));
#87822=CARTESIAN_POINT('Ctrl Pts',(1.21398900848753,-9.86760328992159,11.4481712365411));
#87823=CARTESIAN_POINT('Ctrl Pts',(1.45638535873538,-9.83778181288685,11.4520802604463));
#87824=CARTESIAN_POINT('Ctrl Pts',(1.69767507129333,-9.79902526931674,11.4559892843515));
#87825=CARTESIAN_POINT('Ctrl Pts',(1.93719299710581,-9.75144334403704,11.4598983082567));
#87826=CARTESIAN_POINT('Ctrl Pts',(2.17676359769762,-9.7038509545409,11.4638081918344));
#87827=CARTESIAN_POINT('Ctrl Pts',(2.41456135770987,-9.64742935878678,11.4677180754121));
#87828=CARTESIAN_POINT('Ctrl Pts',(2.64993143540265,-9.582339348388,11.4716279589898));
#87829=CARTESIAN_POINT('Ctrl Pts',(2.81787192934708,-9.53589653541714,11.4744177264307));
#87830=CARTESIAN_POINT('Ctrl Pts',(2.9845766906324,-9.48504164796354,11.4772074938716));
#87831=CARTESIAN_POINT('Ctrl Pts',(3.14981234787031,-9.42984868241287,11.4799972613124));
#87832=CARTESIAN_POINT('Ctrl Pts',(3.3813911808257,-9.35249538734794,11.4839071382662));
#87833=CARTESIAN_POINT('Ctrl Pts',(3.61015460183397,-9.26659544417435,11.48781701522));
#87834=CARTESIAN_POINT('Ctrl Pts',(3.83546920859124,-9.17237918699115,11.4917268921738));
#87835=CARTESIAN_POINT('Ctrl Pts',(4.06074481132754,-9.07817923950453,11.495636092292));
#87836=CARTESIAN_POINT('Ctrl Pts',(4.28257253311811,-8.9756659599215,11.4995452924103));
#87837=CARTESIAN_POINT('Ctrl Pts',(4.50033861067237,-8.86511795687409,11.5034544925286));
#87838=CARTESIAN_POINT('Ctrl Pts',(4.71808098119441,-8.75458198859858,11.5073632670731));
#87839=CARTESIAN_POINT('Ctrl Pts',(4.93176234049709,-8.63601317018384,11.5112720416176));
#87840=CARTESIAN_POINT('Ctrl Pts',(5.14079227414159,-8.50973670533502,11.5151808161621));
#87841=CARTESIAN_POINT('Ctrl Pts',(5.34983842957387,-8.3834504407892,11.5190898940474));
#87842=CARTESIAN_POINT('Ctrl Pts',(5.55423219652298,-8.24945547691004,11.5229989719327));
#87843=CARTESIAN_POINT('Ctrl Pts',(5.75340987018901,-8.10812178408858,11.526908049818));
#87844=CARTESIAN_POINT('Ctrl Pts',(5.95258479342843,-7.96679004293138,11.5308170737233));
#87845=CARTESIAN_POINT('Ctrl Pts',(6.14654354001359,-7.8181199394174,11.5347260976285));
#87846=CARTESIAN_POINT('Ctrl Pts',(6.33475278704742,-7.66252380922858,11.5386351215337));
#87847=CARTESIAN_POINT('Ctrl Pts',(6.52300342505649,-7.50689346034078,11.5425450051114));
#87848=CARTESIAN_POINT('Ctrl Pts',(6.7055018201997,-7.34433421912601,11.5464548886891));
#87849=CARTESIAN_POINT('Ctrl Pts',(6.88174798573371,-7.17529850674173,11.5503647722668));
#87850=CARTESIAN_POINT('Ctrl Pts',(7.00750257776134,-7.05468869384408,11.5531545397077));
#87851=CARTESIAN_POINT('Ctrl Pts',(7.13007481817725,-6.93078250799029,11.5559443071486));
#87852=CARTESIAN_POINT('Ctrl Pts',(7.24929444846749,-6.80375587447245,11.5587340745895));
#87853=CARTESIAN_POINT('Ctrl Pts',(7.41638152464323,-6.6257272332221,11.5626439515432));
#87854=CARTESIAN_POINT('Ctrl Pts',(7.57693294207971,-6.44151337547033,11.566553828497));
#87855=CARTESIAN_POINT('Ctrl Pts',(7.73050060056057,-6.25161774780998,11.5704637054508));
#87856=CARTESIAN_POINT('Ctrl Pts',(7.88404167507424,-6.06175499282076,11.5743729055691));
#87857=CARTESIAN_POINT('Ctrl Pts',(8.03060122779979,-5.86621264919469,11.5782821056874));
#87858=CARTESIAN_POINT('Ctrl Pts',(8.16977136281862,-5.66552732578961,11.5821913058056));
#87859=CARTESIAN_POINT('Ctrl Pts',(8.30892634712674,-5.46486384992587,11.5861000803502));
#87860=CARTESIAN_POINT('Ctrl Pts',(8.44069336027182,-5.25905874245552,11.5900088548947));
#87861=CARTESIAN_POINT('Ctrl Pts',(8.56470717829184,-5.04867853503431,11.5939176294392));
#87862=CARTESIAN_POINT('Ctrl Pts',(8.6887306204162,-4.83828200103678,11.5978267073245));
#87863=CARTESIAN_POINT('Ctrl Pts',(8.80499952013151,-4.62330989756236,11.6017357852098));
#87864=CARTESIAN_POINT('Ctrl Pts',(8.91319341518193,-4.40435547425017,11.6056448630952));
#87865=CARTESIAN_POINT('Ctrl Pts',(9.02138581619239,-4.18540407446033,11.6095538870004));
#87866=CARTESIAN_POINT('Ctrl Pts',(9.12150331321155,-3.96247071704888,11.6134629109056));
#87867=CARTESIAN_POINT('Ctrl Pts',(9.21327229751636,-3.73617151263396,11.6173719348108));
#87868=CARTESIAN_POINT('Ctrl Pts',(9.30506146365513,-3.50982254050067,11.6212818183885));
#87869=CARTESIAN_POINT('Ctrl Pts',(9.3884983421169,-3.28010650177633,11.6251917019663));
#87870=CARTESIAN_POINT('Ctrl Pts',(9.46335769533672,-3.04765895895708,11.629101585544));
#87871=CARTESIAN_POINT('Ctrl Pts',(9.51677109808978,-2.88180374261414,11.6318913529848));
#87872=CARTESIAN_POINT('Ctrl Pts',(9.56581864139675,-2.71455830767632,11.6346811204256));
#87873=CARTESIAN_POINT('Ctrl Pts',(9.61043400671094,-2.5461583223857,11.6374708878664));
#87874=CARTESIAN_POINT('Ctrl Pts',(9.6729627272319,-2.31014466337345,11.6413807648202));
#87875=CARTESIAN_POINT('Ctrl Pts',(9.72680275868779,-2.07179040173455,11.645290641774));
#87876=CARTESIAN_POINT('Ctrl Pts',(9.77179875501628,-1.83175137272019,11.6492005187277));
#87877=CARTESIAN_POINT('Ctrl Pts',(9.81678696212597,-1.59175389665878,11.653109718846));
#87878=CARTESIAN_POINT('Ctrl Pts',(9.85293413867704,-1.35007251079478,11.6570189189643));
#87879=CARTESIAN_POINT('Ctrl Pts',(9.88013606741105,-1.1073731482402,11.6609281190826));
#87880=CARTESIAN_POINT('Ctrl Pts',(9.90733503481589,-0.864700207073136,
11.664836893627));
#87881=CARTESIAN_POINT('Ctrl Pts',(9.92559066760065,-0.621009788950606,
11.6687456681715));
#87882=CARTESIAN_POINT('Ctrl Pts',(9.93485051105835,-0.376973902178435,
11.672654442716));
#87883=CARTESIAN_POINT('Ctrl Pts',(9.94411107312712,-0.132919076977237,
11.6765635206013));
#87884=CARTESIAN_POINT('Ctrl Pts',(9.94437443719738,0.111480990436544,11.6804725984866));
#87885=CARTESIAN_POINT('Ctrl Pts',(9.93564022871477,0.355552029307629,11.6843816763719));
#87886=CARTESIAN_POINT('Ctrl Pts',(9.92690614084202,0.599619697824516,11.6882907002771));
#87887=CARTESIAN_POINT('Ctrl Pts',(9.90917474099365,0.843358066809444,11.6921997241823));
#87888=CARTESIAN_POINT('Ctrl Pts',(9.88249774454809,1.08609499078209,11.6961087480876));
#87889=CARTESIAN_POINT('Ctrl Pts',(9.85581488129786,1.32888529745553,11.7000186316653));
#87890=CARTESIAN_POINT('Ctrl Pts',(9.82018252005589,1.5706734401891,11.703928515243));
#87891=CARTESIAN_POINT('Ctrl Pts',(9.77570418321469,1.81079311967955,11.7078383988207));
#87892=CARTESIAN_POINT('Ctrl Pts',(9.7439681446654,1.98212253408547,11.7106281662616));
#87893=CARTESIAN_POINT('Ctrl Pts',(9.70772964888463,2.15260264564454,11.7134179337025));
#87894=CARTESIAN_POINT('Ctrl Pts',(9.66704222013039,2.32199455516511,11.7162077011434));
#87895=CARTESIAN_POINT('Ctrl Pts',(9.61001852788217,2.55939840233825,11.7201175780971));
#87896=CARTESIAN_POINT('Ctrl Pts',(9.54423661801645,2.79473697410858,11.7240274550509));
#87897=CARTESIAN_POINT('Ctrl Pts',(9.46987114979066,3.02735931239793,11.7279373320047));
#87898=CARTESIAN_POINT('Ctrl Pts',(9.39551855490818,3.25994138163106,11.7318465321229));
#87899=CARTESIAN_POINT('Ctrl Pts',(9.312585453156,3.48980788915068,11.7357557322412));
#87900=CARTESIAN_POINT('Ctrl Pts',(9.22129629668423,3.71632326483553,11.7396649323595));
#87901=CARTESIAN_POINT('Ctrl Pts',(9.13001707837692,3.94281398099733,11.7435737069039));
#87902=CARTESIAN_POINT('Ctrl Pts',(9.03038372642572,4.16595403386053,11.7474824814484));
#87903=CARTESIAN_POINT('Ctrl Pts',(8.92266913374048,4.38512708251367,11.7513912559929));
#87904=CARTESIAN_POINT('Ctrl Pts',(8.81494618185332,4.60431714011355,11.7553003338782));
#87905=CARTESIAN_POINT('Ctrl Pts',(8.6991408569652,4.81953932540157,11.7592094117635));
#87906=CARTESIAN_POINT('Ctrl Pts',(8.57557296203935,5.0302000330742,11.7631184896488));
#87907=CARTESIAN_POINT('Ctrl Pts',(8.45200677345155,5.24085783175187,11.767027513554));
#87908=CARTESIAN_POINT('Ctrl Pts',(8.32067837282204,5.44695403803358,11.7709365374592));
#87909=CARTESIAN_POINT('Ctrl Pts',(8.18195239855599,5.64792164851496,11.7748455613645));
#87910=CARTESIAN_POINT('Ctrl Pts',(8.04319591567539,5.84893345579076,11.7787554449422));
#87911=CARTESIAN_POINT('Ctrl Pts',(7.8970387668655,6.04481418221851,11.7826653285198));
#87912=CARTESIAN_POINT('Ctrl Pts',(7.74388841035309,6.23502656674365,11.7865752120975));
#87913=CARTESIAN_POINT('Ctrl Pts',(7.6346130650195,6.37074629002112,11.7893649795385));
#87914=CARTESIAN_POINT('Ctrl Pts',(7.52177833014649,6.50358084734934,11.7921547469794));
#87915=CARTESIAN_POINT('Ctrl Pts',(7.40554473796219,6.63334539535222,11.7949445144204));
#87916=CARTESIAN_POINT('Ctrl Pts',(7.24264261333854,6.81521124130301,11.7988543913741));
#87917=CARTESIAN_POINT('Ctrl Pts',(7.07301291689818,6.99110117596129,11.8027642683279));
#87918=CARTESIAN_POINT('Ctrl Pts',(6.89711843085032,7.16052521473284,11.8066741452817));
#87919=CARTESIAN_POINT('Ctrl Pts',(6.72125439374738,7.32991992465311,11.8105833454));
#87920=CARTESIAN_POINT('Ctrl Pts',(6.53912793371752,7.49285077870811,11.8144925455183));
#87921=CARTESIAN_POINT('Ctrl Pts',(6.35123834987866,7.64886497612755,11.8184017456366));
#87922=CARTESIAN_POINT('Ctrl Pts',(6.16336922057874,7.80486218911169,11.822310520181));
#87923=CARTESIAN_POINT('Ctrl Pts',(5.96973843576041,7.95394406991516,11.8262192947255));
#87924=CARTESIAN_POINT('Ctrl Pts',(5.77087879767107,8.09569774031803,11.83012806927));
#87925=CARTESIAN_POINT('Ctrl Pts',(5.57200372705975,8.23746241152859,11.8340371471553));
#87926=CARTESIAN_POINT('Ctrl Pts',(5.36789921882674,8.37189757073825,11.8379462250406));
#87927=CARTESIAN_POINT('Ctrl Pts',(5.15912856639042,8.49863262151355,11.841855302926));
#87928=CARTESIAN_POINT('Ctrl Pts',(4.95036079684898,8.62536592221611,11.8457643268312));
#87929=CARTESIAN_POINT('Ctrl Pts',(4.73692725267336,8.74439918343619,11.8496733507364));
#87930=CARTESIAN_POINT('Ctrl Pts',(4.51941805693071,8.85540650826876,11.8535823746416));
#87931=CARTESIAN_POINT('Ctrl Pts',(4.30186102656903,8.96643824583052,11.8574922582193));
#87932=CARTESIAN_POINT('Ctrl Pts',(4.08022680296493,9.06944039173825,11.861402141797));
#87933=CARTESIAN_POINT('Ctrl Pts',(3.85512907384744,9.16413355555102,11.8653120253747));
#87934=CARTESIAN_POINT('Ctrl Pts',(3.69451807271944,9.23169871446921,11.8681017928156));
#87935=CARTESIAN_POINT('Ctrl Pts',(3.53214427256707,9.29503469190088,11.8708915602565));
#87936=CARTESIAN_POINT('Ctrl Pts',(3.36823671880771,9.35405502475132,11.8736813276974));
#87937=CARTESIAN_POINT('Ctrl Pts',(3.13851923139242,9.43677239962426,11.8775912046511));
#87938=CARTESIAN_POINT('Ctrl Pts',(2.90571805417042,9.51103621929828,11.8815010816049));
#87939=CARTESIAN_POINT('Ctrl Pts',(2.67047311957186,9.57663496838238,11.8854109585587));
#87940=CARTESIAN_POINT('Ctrl Pts',(2.43526890802444,9.64222236172265,11.8893201586769));
#87941=CARTESIAN_POINT('Ctrl Pts',(2.1976220534538,9.69914760356212,11.8932293587952));
#87942=CARTESIAN_POINT('Ctrl Pts',(1.95818697265278,9.74724924171599,11.8971385589135));
#87943=CARTESIAN_POINT('Ctrl Pts',(1.71877795787394,9.79534564330067,11.901047333458));
#87944=CARTESIAN_POINT('Ctrl Pts',(1.47758138028183,9.83462030397606,11.9049561080025));
#87945=CARTESIAN_POINT('Ctrl Pts',(1.235262188295,9.86496281423142,11.908864882547));
#87946=CARTESIAN_POINT('Ctrl Pts',(0.992924191103593,9.89530767922025,11.9127739604323));
#87947=CARTESIAN_POINT('Ctrl Pts',(0.749463683207167,9.91671897080718,11.9166830383176));
#87948=CARTESIAN_POINT('Ctrl Pts',(0.505552373690955,9.92913796849734,11.9205921162029));
#87949=CARTESIAN_POINT('Ctrl Pts',(0.26164443232356,9.9415567946947,11.9245011401081));
#87950=CARTESIAN_POINT('Ctrl Pts',(0.0172859818579282,9.9449835631453,11.9284101640133));
#87951=CARTESIAN_POINT('Ctrl Pts',(-0.226848878373291,9.93941163180099,
11.9323191879186));
#87952=CARTESIAN_POINT('Ctrl Pts',(-0.471037428739418,9.93383847507761,
11.9362290714963));
#87953=CARTESIAN_POINT('Ctrl Pts',(-0.715002010243568,9.91926266958761,
11.940138955074));
#87954=CARTESIAN_POINT('Ctrl Pts',(-0.95806986473244,9.89572969185656,11.9440488386517));
#87955=CARTESIAN_POINT('Ctrl Pts',(-1.13150285139464,9.87893851796179,11.9468386060925));
#87956=CARTESIAN_POINT('Ctrl Pts',(-1.30447933666542,9.85758828243919,11.9496283735334));
#87957=CARTESIAN_POINT('Ctrl Pts',(-1.4767566858202,9.83171163586917,11.9524181409743));
#87958=CARTESIAN_POINT('Ctrl Pts',(-1.71820449514073,9.79544534980461,11.9563280179281));
#87959=CARTESIAN_POINT('Ctrl Pts',(-1.95835265971994,9.75027498254813,11.9602378948819));
#87960=CARTESIAN_POINT('Ctrl Pts',(-2.1965375493256,9.69631820818617,11.9641477718357));
#87961=CARTESIAN_POINT('Ctrl Pts',(-2.43468120694782,9.64237077423548,11.968056971954));
#87962=CARTESIAN_POINT('Ctrl Pts',(-2.67086199478642,9.57964003135387,11.9719661720723));
#87963=CARTESIAN_POINT('Ctrl Pts',(-2.90442730406609,9.50829459132369,11.9758753721906));
#87964=CARTESIAN_POINT('Ctrl Pts',(-3.13796718633633,9.43695691829103,11.9797841467351));
#87965=CARTESIAN_POINT('Ctrl Pts',(-3.36889189058786,9.35700650252349,11.9836929212796));
#87966=CARTESIAN_POINT('Ctrl Pts',(-3.59656377335176,9.26866187883741,11.9876016958242));
#87967=CARTESIAN_POINT('Ctrl Pts',(-3.82425332461187,9.18031039915914,11.9915107737095));
#87968=CARTESIAN_POINT('Ctrl Pts',(-4.04868928751855,9.08356350842259,11.9954198515948));
#87969=CARTESIAN_POINT('Ctrl Pts',(-4.26925260961267,8.97868844293616,11.9993289294802));
#87970=CARTESIAN_POINT('Ctrl Pts',(-4.48981288596899,8.87381482565947,12.0032379533854));
#87971=CARTESIAN_POINT('Ctrl Pts',(-4.70650037618384,8.76081338035352,12.0071469772906));
#87972=CARTESIAN_POINT('Ctrl Pts',(-4.91871865012074,8.63999831255507,12.0110560011959));
#87973=CARTESIAN_POINT('Ctrl Pts',(-5.13098359509581,8.51915667510954,12.0149658847736));
#87974=CARTESIAN_POINT('Ctrl Pts',(-5.33877711565538,8.39049811943732,12.0188757683513));
#87975=CARTESIAN_POINT('Ctrl Pts',(-5.54152870707573,8.25438208399972,12.022785651929));
#87976=CARTESIAN_POINT('Ctrl Pts',(-5.68619536455216,8.15726101216125,12.0255754193697));
#87977=CARTESIAN_POINT('Ctrl Pts',(-5.82829568684554,8.05634423746679,12.0283651868105));
#87978=CARTESIAN_POINT('Ctrl Pts',(-5.96763163245033,7.951775694735,12.0311549542513));
#87979=CARTESIAN_POINT('Ctrl Pts',(-6.162911853515,7.80522221169484,12.035064831205));
#87980=CARTESIAN_POINT('Ctrl Pts',(-6.352820743239,7.65144927313826,12.0389747081588));
#87981=CARTESIAN_POINT('Ctrl Pts',(-6.53683010861459,7.49087552500439,12.0428845851126));
#87982=CARTESIAN_POINT('Ctrl Pts',(-6.72080762028672,7.33032957365437,12.0467937852309));
#87983=CARTESIAN_POINT('Ctrl Pts',(-6.89888743518115,7.1629853470611,12.0507029853492));
#87984=CARTESIAN_POINT('Ctrl Pts',(-7.07057524467959,6.98930108875875,12.0546121854675));
#87985=CARTESIAN_POINT('Ctrl Pts',(-7.24224436343932,6.81563573853785,12.058520960012));
#87986=CARTESIAN_POINT('Ctrl Pts',(-7.4075226692328,6.63563193400119,12.0624297345565));
#87987=CARTESIAN_POINT('Ctrl Pts',(-7.56595272707869,6.44978475079677,12.066338509101));
#87988=CARTESIAN_POINT('Ctrl Pts',(-7.7243950799046,6.26392314490366,12.0702475869863));
#87989=CARTESIAN_POINT('Ctrl Pts',(-7.87598793863131,6.07221746555143,12.0741566648717));
#87990=CARTESIAN_POINT('Ctrl Pts',(-8.02031335293776,5.87519682399563,12.078065742757));
#87991=CARTESIAN_POINT('Ctrl Pts',(-8.16463677426606,5.67817890308216,12.0819747666622));
#87992=CARTESIAN_POINT('Ctrl Pts',(-8.30169278788719,5.47584639411476,12.0858837905673));
#87993=CARTESIAN_POINT('Ctrl Pts',(-8.43110565365917,5.26875900538603,12.0897928144725));
#87994=CARTESIAN_POINT('Ctrl Pts',(-8.56054697990804,5.06162607399965,12.0937026980502));
#87995=CARTESIAN_POINT('Ctrl Pts',(-8.6823416501597,4.8497364106546,12.0976125816279));
#87996=CARTESIAN_POINT('Ctrl Pts',(-8.79615821714132,4.63367722430223,12.1015224652056));
#87997=CARTESIAN_POINT('Ctrl Pts',(-8.8773682446238,4.47951537487349,12.1043122326465));
#87998=CARTESIAN_POINT('Ctrl Pts',(-8.9545174967614,4.32323137086869,12.1071020000874));
#87999=CARTESIAN_POINT('Ctrl Pts',(-9.02750001457516,4.16504591653506,12.1098917675283));
#88000=CARTESIAN_POINT('Ctrl Pts',(-9.12940431381605,3.9441741467353,12.1137870743034));
#88001=CARTESIAN_POINT('Ctrl Pts',(-9.22321658138155,3.71952196105995,12.1176823810786));
#88002=CARTESIAN_POINT('Ctrl Pts',(-9.30867171303844,3.49170373011198,12.1215776878538));
#88003=CARTESIAN_POINT('Ctrl Pts',(-9.39411098950818,3.26392776813745,12.1254722719009));
#88004=CARTESIAN_POINT('Ctrl Pts',(-9.47119612523989,3.03298719968502,12.129366855948));
#88005=CARTESIAN_POINT('Ctrl Pts',(-9.53971060835845,2.79951522745873,12.1332614399952));
#88006=CARTESIAN_POINT('Ctrl Pts',(-9.60822488072106,2.56604397341062,12.1371560120623));
#88007=CARTESIAN_POINT('Ctrl Pts',(-9.66816846912883,2.3300416029902,12.1410505841294));
#88008=CARTESIAN_POINT('Ctrl Pts',(-9.71937473864423,2.09215646876718,12.1449451561965));
#88009=CARTESIAN_POINT('Ctrl Pts',(-9.77057792428616,1.85428566106437,12.1488394937148));
#88010=CARTESIAN_POINT('Ctrl Pts',(-9.81304478356313,1.61453259450658,12.1527338312331));
#88011=CARTESIAN_POINT('Ctrl Pts',(-9.84665965976869,1.37355653130258,12.1566281687514));
#88012=CARTESIAN_POINT('Ctrl Pts',(-9.88028121308345,1.13253260168737,12.1605232798236));
#88013=CARTESIAN_POINT('Ctrl Pts',(-9.90504722845266,0.890285471654712,
12.1644183908958));
#88014=CARTESIAN_POINT('Ctrl Pts',(-9.92089368692205,0.647481623515401,
12.1683135019679));
#88015=CARTESIAN_POINT('Ctrl Pts',(-9.93496511211645,0.431875329364309,
12.1717723040834));
#88016=CARTESIAN_POINT('Ctrl Pts',(-9.94200401926865,0.215830279218862,
12.1752311061988));
#88017=CARTESIAN_POINT('Ctrl Pts',(-9.94199999827757,-0.000185064137654065,
12.1786899083142));
#88018=CARTESIAN_POINT('Origin',(0.,0.,0.));
#88019=CARTESIAN_POINT('',(-9.94195875194945,-0.000111575420876506,13.3213100922243));
#88020=CARTESIAN_POINT('',(-9.94195498619804,-0.000106503573575908,13.1786899087943));
#88021=CARTESIAN_POINT('',(-9.942,-1.2175438477123E-15,0.));
#88022=CARTESIAN_POINT('Ctrl Pts',(-9.94125749983017,-0.000111533904790795,
13.3213100916858));
#88023=CARTESIAN_POINT('Ctrl Pts',(-9.94087740012148,0.947889144334461,
13.3061371289177));
#88024=CARTESIAN_POINT('Ctrl Pts',(-9.57342153214947,3.5359933036782,13.2647185617242));
#88025=CARTESIAN_POINT('Ctrl Pts',(-7.35748914925443,7.28899342376248,13.1970543901046));
#88026=CARTESIAN_POINT('Ctrl Pts',(-3.01465202171707,9.90827658581459,13.1183175768277));
#88027=CARTESIAN_POINT('Ctrl Pts',(2.05108274737684,10.1516073247769,13.0395807635506));
#88028=CARTESIAN_POINT('Ctrl Pts',(6.62497870056853,7.96063621389991,12.9608439502738));
#88029=CARTESIAN_POINT('Ctrl Pts',(9.61023973221781,3.86074656023302,12.8821071369967));
#88030=CARTESIAN_POINT('Ctrl Pts',(10.2910160050407,-1.16492973910139,12.8033703237197));
#88031=CARTESIAN_POINT('Ctrl Pts',(8.50406096238505,-5.91126203623941,12.7246335104427));
#88032=CARTESIAN_POINT('Ctrl Pts',(4.67787699079448,-9.24010490048894,12.6458966971659));
#88033=CARTESIAN_POINT('Ctrl Pts',(-0.270037190378026,-10.3532193847547,
12.5671598838888));
#88034=CARTESIAN_POINT('Ctrl Pts',(-5.15319787872579,-8.98368651143514,
12.4884230706118));
#88035=CARTESIAN_POINT('Ctrl Pts',(-8.80064891761229,-5.45991303428693,
12.4096862573348));
#88036=CARTESIAN_POINT('Ctrl Pts',(-9.88811005993012,-2.04066390104026,
12.3539819310262));
#88037=CARTESIAN_POINT('Ctrl Pts',(-9.94269391643093,-0.200861641353821,
12.3245232091432));
#88038=CARTESIAN_POINT('Ctrl Pts',(-9.94252421102867,-0.000180935334070931,
12.3213100916858));
#88039=CARTESIAN_POINT('Ctrl Pts',(-9.94250794012056,-0.000185073592678929,
12.1786899083142));
#88040=CARTESIAN_POINT('Ctrl Pts',(-9.94268579522292,-0.207098276547491,
12.1820027991445));
#88041=CARTESIAN_POINT('Ctrl Pts',(-9.8862140376245,-2.05313606585478,12.2115612944009));
#88042=CARTESIAN_POINT('Ctrl Pts',(-8.79036500190181,-5.47645461378649,
12.2673653940818));
#88043=CARTESIAN_POINT('Ctrl Pts',(-5.13629330883765,-8.99336216601434,
12.3461022073594));
#88044=CARTESIAN_POINT('Ctrl Pts',(-0.250565592938094,-10.3537089435215,
12.4248390206361));
#88045=CARTESIAN_POINT('Ctrl Pts',(4.6952464295034,-9.2312909698346,12.5035758339132));
#88046=CARTESIAN_POINT('Ctrl Pts',(8.51516314264787,-5.89525815020917,12.5823126471901));
#88047=CARTESIAN_POINT('Ctrl Pts',(10.2931886826346,-1.14557354508644,12.661049460467));
#88048=CARTESIAN_POINT('Ctrl Pts',(9.60296191052419,3.87881354908099,12.7397862737441));
#88049=CARTESIAN_POINT('Ctrl Pts',(6.60999556281344,7.97308162902553,12.8185230870211));
#88050=CARTESIAN_POINT('Ctrl Pts',(2.03198717090202,10.1554468213272,12.8972599002979));
#88051=CARTESIAN_POINT('Ctrl Pts',(-3.0332810184704,9.90258947278456,12.975996713575));
#88052=CARTESIAN_POINT('Ctrl Pts',(-7.37118443120105,7.27514344083582,13.054733526852));
#88053=CARTESIAN_POINT('Ctrl Pts',(-9.57679763346346,3.52352256269792,13.1222979250984));
#88054=CARTESIAN_POINT('Ctrl Pts',(-9.94088989120619,0.941662455610846,
13.1636167189191));
#88055=CARTESIAN_POINT('Ctrl Pts',(-9.94124998359704,-0.000106466024951112,
13.1786899083142));
#88056=CARTESIAN_POINT('Origin',(0.,0.,0.));
#88057=CARTESIAN_POINT('',(-9.94199999708082,0.000240925445847458,14.3213100916727));
#88058=CARTESIAN_POINT('',(-9.9419999970495,0.000242214229021048,14.178689908302));
#88059=CARTESIAN_POINT('',(-9.942,-1.2175438477123E-15,0.));
#88060=CARTESIAN_POINT('Ctrl Pts',(-9.94199999708082,0.00024092544577925,
14.3213100916727));
#88061=CARTESIAN_POINT('Ctrl Pts',(-9.94199381537137,0.255334591941568,
14.3172267605938));
#88062=CARTESIAN_POINT('Ctrl Pts',(-9.93216543361595,0.510380829635011,
14.3131434295148));
#88063=CARTESIAN_POINT('Ctrl Pts',(-9.91255176743128,0.764644661261096,
14.3090600984358));
#88064=CARTESIAN_POINT('Ctrl Pts',(-9.89703643234913,0.965779345098612,
14.3058299909513));
#88065=CARTESIAN_POINT('Ctrl Pts',(-9.87539892454686,1.16642442817123,14.3025998834667));
#88066=CARTESIAN_POINT('Ctrl Pts',(-9.84768052877541,1.36621821213805,14.2993697759822));
#88067=CARTESIAN_POINT('Ctrl Pts',(-9.81412885368643,1.60805818656242,14.2954598990284));
#88068=CARTESIAN_POINT('Ctrl Pts',(-9.77165905958109,1.84869862293535,14.2915500220746));
#88069=CARTESIAN_POINT('Ctrl Pts',(-9.72038135817929,2.08747461099783,14.2876401451208));
#88070=CARTESIAN_POINT('Ctrl Pts',(-9.66911253341697,2.32620926475113,14.2837309450025));
#88071=CARTESIAN_POINT('Ctrl Pts',(-9.60903890388906,2.56307984055476,14.2798217448842));
#88072=CARTESIAN_POINT('Ctrl Pts',(-9.54032173960764,2.79743187669866,14.2759125447659));
#88073=CARTESIAN_POINT('Ctrl Pts',(-9.47161205619742,3.03175840018625,14.2720037702214));
#88074=CARTESIAN_POINT('Ctrl Pts',(-9.39426079570019,3.26356666258029,14.2680949956769));
#88075=CARTESIAN_POINT('Ctrl Pts',(-9.3084793161259,3.49221660571855,14.2641862211323));
#88076=CARTESIAN_POINT('Ctrl Pts',(-9.22269117947215,3.72088429325624,14.260277143247));
#88077=CARTESIAN_POINT('Ctrl Pts',(-9.12847161206279,3.9463929082363,14.2563680653617));
#88078=CARTESIAN_POINT('Ctrl Pts',(-9.02608087917035,4.16812043524122,14.2524589874764));
#88079=CARTESIAN_POINT('Ctrl Pts',(-8.92369156018213,4.38984490043109,14.2485499635712));
#88080=CARTESIAN_POINT('Ctrl Pts',(-8.81313142077705,4.60778812843122,14.2446409396659));
#88081=CARTESIAN_POINT('Ctrl Pts',(-8.69470794662194,4.82135019708683,14.2407319157607));
#88082=CARTESIAN_POINT('Ctrl Pts',(-8.57625842877817,5.03495923230939,14.236822032183));
#88083=CARTESIAN_POINT('Ctrl Pts',(-8.44994225585272,5.24418493721204,14.2329121486053));
#88084=CARTESIAN_POINT('Ctrl Pts',(-8.31611243481795,5.44845280528943,14.2290022650276));
#88085=CARTESIAN_POINT('Ctrl Pts',(-8.22062261525989,5.59420135156561,14.2262124975868));
#88086=CARTESIAN_POINT('Ctrl Pts',(-8.1213085032248,5.73742636391226,14.2234227301461));
#88087=CARTESIAN_POINT('Ctrl Pts',(-8.01831179973473,5.87792819641707,14.2206329627053));
#88088=CARTESIAN_POINT('Ctrl Pts',(-7.87396125947005,6.07484241544545,14.2167230857515));
#88089=CARTESIAN_POINT('Ctrl Pts',(-7.72233137996095,6.26646674236815,14.2128132087978));
#88090=CARTESIAN_POINT('Ctrl Pts',(-7.56383484723363,6.45226831461419,14.208903331844));
#88091=CARTESIAN_POINT('Ctrl Pts',(-7.40536575170677,6.63803772290751,14.2049941317257));
#88092=CARTESIAN_POINT('Ctrl Pts',(-7.24003255766611,6.81798617551003,14.2010849316075));
#88093=CARTESIAN_POINT('Ctrl Pts',(-7.06828792687721,6.99161424727952,14.1971757314892));
#88094=CARTESIAN_POINT('Ctrl Pts',(-6.89656199301152,7.1652234170856,14.1932669569447));
#88095=CARTESIAN_POINT('Ctrl Pts',(-6.71842621308652,7.33251338069326,14.1893581824002));
#88096=CARTESIAN_POINT('Ctrl Pts',(-6.53437049288043,7.49302117051417,14.1854494078557));
#88097=CARTESIAN_POINT('Ctrl Pts',(-6.35030048901242,7.65354141655759,14.1815403299704));
#88098=CARTESIAN_POINT('Ctrl Pts',(-6.16030983611704,7.80727825054629,14.1776312520851));
#88099=CARTESIAN_POINT('Ctrl Pts',(-5.96492291698645,7.95380780471907,14.1737221741998));
#88100=CARTESIAN_POINT('Ctrl Pts',(-5.76953869593587,8.10033533547869,14.1698131502946));
#88101=CARTESIAN_POINT('Ctrl Pts',(-5.5687585831884,8.23965561892998,14.1659041263894));
#88102=CARTESIAN_POINT('Ctrl Pts',(-5.3631380308139,8.37138665111328,14.1619951024842));
#88103=CARTESIAN_POINT('Ctrl Pts',(-5.15747225837047,8.50314665358329,14.1580852189065));
#88104=CARTESIAN_POINT('Ctrl Pts',(-4.94696415481059,8.62731391766556,14.1541753353288));
#88105=CARTESIAN_POINT('Ctrl Pts',(-4.73219716869498,8.743550420544,14.1502654517511));
#88106=CARTESIAN_POINT('Ctrl Pts',(-4.57895732578351,8.82648711283471,14.1474756843102));
#88107=CARTESIAN_POINT('Ctrl Pts',(-4.42354984516734,8.90538712539718,14.1446859168692));
#88108=CARTESIAN_POINT('Ctrl Pts',(-4.26619422686921,8.9801420266401,14.1418961494283));
#88109=CARTESIAN_POINT('Ctrl Pts',(-4.04565931900939,9.08491149998959,14.1379862724745));
#88110=CARTESIAN_POINT('Ctrl Pts',(-3.82122939880282,9.18156921538258,14.1340763955208));
#88111=CARTESIAN_POINT('Ctrl Pts',(-3.59352066665134,9.26984213556788,14.130166518567));
#88112=CARTESIAN_POINT('Ctrl Pts',(-3.36585135296519,9.3580997749029,14.1262573184487));
#88113=CARTESIAN_POINT('Ctrl Pts',(-3.13490462160746,9.43797541525384,14.1223481183304));
#88114=CARTESIAN_POINT('Ctrl Pts',(-2.90131598019526,9.50924442755909,14.1184389182121));
#88115=CARTESIAN_POINT('Ctrl Pts',(-2.6677527683341,9.58050568118663,14.1145301436676));
#88116=CARTESIAN_POINT('Ctrl Pts',(-2.43154848869088,9.64316209580029,14.1106213691231));
#88117=CARTESIAN_POINT('Ctrl Pts',(-2.19335411799256,9.69703881156949,14.1067125945786));
#88118=CARTESIAN_POINT('Ctrl Pts',(-1.95514126219735,9.75091970844636,14.1028035166932));
#88119=CARTESIAN_POINT('Ctrl Pts',(-1.71493827948673,9.79601948017485,14.0988944388079));
#88120=CARTESIAN_POINT('Ctrl Pts',(-1.47340792594698,9.83221404790176,14.0949853609226));
#88121=CARTESIAN_POINT('Ctrl Pts',(-1.23188090767788,9.86840811582118,14.0910763370174));
#88122=CARTESIAN_POINT('Ctrl Pts',(-0.989026832777744,9.89569718617364,
14.0871673131121));
#88123=CARTESIAN_POINT('Ctrl Pts',(-0.745515925245146,9.9140087757277,14.0832582892069));
#88124=CARTESIAN_POINT('Ctrl Pts',(-0.501951464797451,9.93232439236626,
14.0793484056292));
#88125=CARTESIAN_POINT('Ctrl Pts',(-0.257730162639278,9.9416585611352,14.0754385220515));
#88126=CARTESIAN_POINT('Ctrl Pts',(-0.0135260010347294,9.94199079899474,
14.0715286384738));
#88127=CARTESIAN_POINT('Ctrl Pts',(0.160717759787237,9.94222785627399,14.068738871033));
#88128=CARTESIAN_POINT('Ctrl Pts',(0.334952715461797,9.93788306251751,14.0659491035921));
#88129=CARTESIAN_POINT('Ctrl Pts',(0.508934201912364,9.92896520177827,14.0631593361513));
#88130=CARTESIAN_POINT('Ctrl Pts',(0.752770370585048,9.91646676277895,14.0592494591976));
#88131=CARTESIAN_POINT('Ctrl Pts',(0.996183221306394,9.89497985671135,14.0553395822438));
#88132=CARTESIAN_POINT('Ctrl Pts',(1.23850080090258,9.86455674453564,14.05142970529));
#88133=CARTESIAN_POINT('Ctrl Pts',(1.48077643310792,9.8341388988791,14.0475205051717));
#88134=CARTESIAN_POINT('Ctrl Pts',(1.72195689468522,9.79478797005619,14.0436113050534));
#88135=CARTESIAN_POINT('Ctrl Pts',(1.9613762235378,9.74660798994915,14.0397021049352));
#88136=CARTESIAN_POINT('Ctrl Pts',(2.20076948808366,9.69843325493985,14.0357933303907));
#88137=CARTESIAN_POINT('Ctrl Pts',(2.43840172802136,9.64143144307507,14.0318845558462));
#88138=CARTESIAN_POINT('Ctrl Pts',(2.6736169964581,9.57575773274629,14.0279757813017));
#88139=CARTESIAN_POINT('Ctrl Pts',(2.90885051879817,9.51007892580296,14.0240667034164));
#88140=CARTESIAN_POINT('Ctrl Pts',(3.14166642401248,9.43572694807593,14.020157625531));
#88141=CARTESIAN_POINT('Ctrl Pts',(3.37142250813172,9.35290726307402,14.0162485476457));
#88142=CARTESIAN_POINT('Ctrl Pts',(3.60117541957035,9.27008872172152,14.0123395237405));
#88143=CARTESIAN_POINT('Ctrl Pts',(3.82786833139906,9.17880280395386,14.0084304998353));
#88144=CARTESIAN_POINT('Ctrl Pts',(4.05087696386757,9.07930392836406,14.00452147593));
#88145=CARTESIAN_POINT('Ctrl Pts',(4.27393464039106,8.97978317098309,14.0006115923523));
#88146=CARTESIAN_POINT('Ctrl Pts',(4.4933061620441,8.87204596004006,13.9967017087747));
#88147=CARTESIAN_POINT('Ctrl Pts',(4.70838863024847,8.75639426399628,13.992791825197));
#88148=CARTESIAN_POINT('Ctrl Pts',(4.86185357491384,8.67387484118144,13.9900020577561));
#88149=CARTESIAN_POINT('Ctrl Pts',(5.01313538300763,8.58732709971537,13.9872122903152));
#88150=CARTESIAN_POINT('Ctrl Pts',(5.16202289555344,8.49687493292576,13.9844225228743));
#88151=CARTESIAN_POINT('Ctrl Pts',(5.37068969891424,8.3701056412752,13.9805126459206));
#88152=CARTESIAN_POINT('Ctrl Pts',(5.57471636343581,8.23562656040066,13.9766027689668));
#88153=CARTESIAN_POINT('Ctrl Pts',(5.77353631399643,8.0938027175713,13.972692892013));
#88154=CARTESIAN_POINT('Ctrl Pts',(5.97232184700406,7.95200342574706,13.9687836918947));
#88155=CARTESIAN_POINT('Ctrl Pts',(6.16590223721962,7.80286207276289,13.9648744917764));
#88156=CARTESIAN_POINT('Ctrl Pts',(6.3537407622623,7.64678640514866,13.9609652916581));
#88157=CARTESIAN_POINT('Ctrl Pts',(6.54155883832555,7.49072772866082,13.9570565171137));
#88158=CARTESIAN_POINT('Ctrl Pts',(6.72363608179566,7.32773642391084,13.9531477425692));
#88159=CARTESIAN_POINT('Ctrl Pts',(6.89946886821635,7.15826049655315,13.9492389680247));
#88160=CARTESIAN_POINT('Ctrl Pts',(7.07531530015708,6.98877141700007,13.9453298901393));
#88161=CARTESIAN_POINT('Ctrl Pts',(7.24491610275595,6.81279690159931,13.941420812254));
#88162=CARTESIAN_POINT('Ctrl Pts',(7.40780362128244,6.63082268715691,13.9375117343687));
#88163=CARTESIAN_POINT('Ctrl Pts',(7.57068889050987,6.44885098558002,13.9336027104635));
#88164=CARTESIAN_POINT('Ctrl Pts',(7.72686087564029,6.26087996090791,13.9296936865583));
#88165=CARTESIAN_POINT('Ctrl Pts',(7.87589094016046,6.06742992532245,13.9257846626531));
#88166=CARTESIAN_POINT('Ctrl Pts',(8.02495377937031,5.8739373462079,13.9218747790754));
#88167=CARTESIAN_POINT('Ctrl Pts',(8.16687138760884,5.67496357003133,13.9179648954977));
#88168=CARTESIAN_POINT('Ctrl Pts',(8.30125652188029,5.47106060631209,13.91405501192));
#88169=CARTESIAN_POINT('Ctrl Pts',(8.39714256674027,5.32557242540382,13.9112652444791));
#88170=CARTESIAN_POINT('Ctrl Pts',(8.48919464823038,5.17757542777753,13.9084754770382));
#88171=CARTESIAN_POINT('Ctrl Pts',(8.57728574728231,5.02727890706968,13.9056857095974));
#88172=CARTESIAN_POINT('Ctrl Pts',(8.70074598736159,4.81663736973645,13.9017758326436));
#88173=CARTESIAN_POINT('Ctrl Pts',(8.81646194851377,4.60141348778228,13.8978659556898));
#88174=CARTESIAN_POINT('Ctrl Pts',(8.92410829539268,4.38219752317299,13.893956078736));
#88175=CARTESIAN_POINT('Ctrl Pts',(9.03173600770384,4.1630195068533,13.8900468786177));
#88176=CARTESIAN_POINT('Ctrl Pts',(9.13129677082437,3.93985103889019,13.8861376784995));
#88177=CARTESIAN_POINT('Ctrl Pts',(9.22251180528306,3.71330580499569,13.8822284783812));
#88178=CARTESIAN_POINT('Ctrl Pts',(9.31371690964677,3.48678523387418,13.8783197038367));
#88179=CARTESIAN_POINT('Ctrl Pts',(9.39657799478445,3.25688889074633,13.8744109292922));
#88180=CARTESIAN_POINT('Ctrl Pts',(9.47086452516248,3.02425017913844,13.8705021547477));
#88181=CARTESIAN_POINT('Ctrl Pts',(9.54515682055384,2.79159341358098,13.8665930768624));
#88182=CARTESIAN_POINT('Ctrl Pts',(9.61087314333497,2.55619412039391,13.8626839989771));
#88183=CARTESIAN_POINT('Ctrl Pts',(9.66783252914998,2.31870183255837,13.8587749210917));
#88184=CARTESIAN_POINT('Ctrl Pts',(9.72479112841801,2.08121282423224,13.8548658971865));
#88185=CARTESIAN_POINT('Ctrl Pts',(9.77299296919136,1.84163115214076,13.8509568732813));
#88186=CARTESIAN_POINT('Ctrl Pts',(9.81230784296712,1.60061825394001,13.8470478493761));
#88187=CARTESIAN_POINT('Ctrl Pts',(9.85163136286934,1.35955235218624,13.8431379657984));
#88188=CARTESIAN_POINT('Ctrl Pts',(9.88206396436919,1.11705487199269,13.8392280822207));
#88189=CARTESIAN_POINT('Ctrl Pts',(9.90352691887965,0.87379549496791,13.835318198643));
#88190=CARTESIAN_POINT('Ctrl Pts',(9.918841096524,0.700225853770615,13.8325284312021));
#88191=CARTESIAN_POINT('Ctrl Pts',(9.92958984817828,0.526268498794397,13.8297386637613));
#88192=CARTESIAN_POINT('Ctrl Pts',(9.93576075318437,0.352167936475196,13.8269488963204));
#88193=CARTESIAN_POINT('Ctrl Pts',(9.94440931611256,0.108164882212393,13.8230390193667));
#88194=CARTESIAN_POINT('Ctrl Pts',(9.94406649723332,-0.136194250016732,
13.8191291424129));
#88195=CARTESIAN_POINT('Ctrl Pts',(9.9347262146747,-0.380235505253301,13.8152192654591));
#88196=CARTESIAN_POINT('Ctrl Pts',(9.92538754900448,-0.624234514715135,
13.8113100653409));
#88197=CARTESIAN_POINT('Ctrl Pts',(9.90705453957857,-0.867915477063908,
13.8074008652226));
#88198=CARTESIAN_POINT('Ctrl Pts',(9.87977319968096,-1.11060592599979,13.8034916651043));
#88199=CARTESIAN_POINT('Ctrl Pts',(9.85249482975749,-1.35326995451939,13.7995828905598));
#88200=CARTESIAN_POINT('Ctrl Pts',(9.81627010574047,-1.59494340648189,13.7956741160153));
#88201=CARTESIAN_POINT('Ctrl Pts',(9.77119686222301,-1.83495936731123,13.7917653414708));
#88202=CARTESIAN_POINT('Ctrl Pts',(9.72612012079218,-2.07499395460216,13.7878562635855));
#88203=CARTESIAN_POINT('Ctrl Pts',(9.6721935364453,-2.31337051765586,13.7839471857002));
#88204=CARTESIAN_POINT('Ctrl Pts',(9.60956622949839,-2.54943148189631,13.7800381078149));
#88205=CARTESIAN_POINT('Ctrl Pts',(9.54693978736628,-2.78548918639237,13.7761290839096));
#88206=CARTESIAN_POINT('Ctrl Pts',(9.47561293680516,-3.01923108559936,13.7722200600044));
#88207=CARTESIAN_POINT('Ctrl Pts',(9.39578512063412,-3.25001322564547,13.7683110360992));
#88208=CARTESIAN_POINT('Ctrl Pts',(9.31593974873091,-3.48084611929645,13.7644011525215));
#88209=CARTESIAN_POINT('Ctrl Pts',(9.2275897662953,-3.70871768781189,13.7604912689438));
#88210=CARTESIAN_POINT('Ctrl Pts',(9.13098383784858,-3.93300116360878,13.7565813853661));
#88211=CARTESIAN_POINT('Ctrl Pts',(9.06205388931622,-4.09303118135107,13.7537916179252));
#88212=CARTESIAN_POINT('Ctrl Pts',(8.98892181722655,-4.2512348382156,13.7510018504843));
#88213=CARTESIAN_POINT('Ctrl Pts',(8.91169277773993,-4.40739104631959,13.7482120830434));
#88214=CARTESIAN_POINT('Ctrl Pts',(8.80345578377937,-4.62624497310424,13.7443022060896));
#88215=CARTESIAN_POINT('Ctrl Pts',(8.68713639102615,-4.84114332558387,13.7403923291359));
#88216=CARTESIAN_POINT('Ctrl Pts',(8.56304922948336,-5.0514900666481,13.7364824521821));
#88217=CARTESIAN_POINT('Ctrl Pts',(8.43898354856387,-5.26180039476637,13.7325732520638));
#88218=CARTESIAN_POINT('Ctrl Pts',(8.30715292547827,-5.46756044303394,13.7286640519455));
#88219=CARTESIAN_POINT('Ctrl Pts',(8.16791713252317,-5.66820021843217,13.7247548518272));
#88220=CARTESIAN_POINT('Ctrl Pts',(8.02869649742703,-5.86881815124701,13.7208460772827));
#88221=CARTESIAN_POINT('Ctrl Pts',(7.88207246185683,-6.06431669397078,13.7169373027382));
#88222=CARTESIAN_POINT('Ctrl Pts',(7.72844777031341,-6.25415534357259,13.7130285281937));
#88223=CARTESIAN_POINT('Ctrl Pts',(7.57481115671128,-6.44400872562077,13.7091194503083));
#88224=CARTESIAN_POINT('Ctrl Pts',(7.41417297550338,-6.62820111702483,13.705210372423));
#88225=CARTESIAN_POINT('Ctrl Pts',(7.24697667341301,-6.80622458452612,13.7013012945377));
#88226=CARTESIAN_POINT('Ctrl Pts',(7.07978268012128,-6.98424559371742,13.6973922706325));
#88227=CARTESIAN_POINT('Ctrl Pts',(6.90603094048115,-7.15609764644923,13.6934832467273));
#88228=CARTESIAN_POINT('Ctrl Pts',(6.72620272329846,-7.32130868937326,13.689574222822));
#88229=CARTESIAN_POINT('Ctrl Pts',(6.54633495829673,-7.48655606550757,13.6856643392443));
#88230=CARTESIAN_POINT('Ctrl Pts',(6.36038825134543,-7.64515932306672,13.6817544556666));
#88231=CARTESIAN_POINT('Ctrl Pts',(6.16887903163457,-7.79668490405117,13.6778445720889));
#88232=CARTESIAN_POINT('Ctrl Pts',(6.03223399473014,-7.90480094481853,13.6750548046481));
#88233=CARTESIAN_POINT('Ctrl Pts',(5.89275778374903,-8.0093145017494,13.6722650372073));
#88234=CARTESIAN_POINT('Ctrl Pts',(5.75064791577785,-8.11008092122143,13.6694752697664));
#88235=CARTESIAN_POINT('Ctrl Pts',(5.55148002473702,-8.25130570413412,13.6655653928127));
#88236=CARTESIAN_POINT('Ctrl Pts',(5.34707683448481,-8.38521178630878,13.6616555158589));
#88237=CARTESIAN_POINT('Ctrl Pts',(5.13799824028541,-8.51142397503638,13.6577456389051));
#88238=CARTESIAN_POINT('Ctrl Pts',(4.928955839504,-8.6376143152791,13.6538364387868));
#88239=CARTESIAN_POINT('Ctrl Pts',(4.71523989028925,-8.75611327602244,13.6499272386685));
#88240=CARTESIAN_POINT('Ctrl Pts',(4.49743765245278,-8.86659001884603,13.6460180385503));
#88241=CARTESIAN_POINT('Ctrl Pts',(4.27965912558583,-8.97705473465507,13.6421092640058));
#88242=CARTESIAN_POINT('Ctrl Pts',(4.0577954482182,-9.07949884955958,13.6382004894613));
#88243=CARTESIAN_POINT('Ctrl Pts',(3.83245769875314,-9.17363788184752,13.6342917149168));
#88244=CARTESIAN_POINT('Ctrl Pts',(3.6071024619304,-9.26778421980409,13.6303826370314));
#88245=CARTESIAN_POINT('Ctrl Pts',(3.37827287176535,-9.35362407638387,13.6264735591461));
#88246=CARTESIAN_POINT('Ctrl Pts',(3.14660036520514,-9.43092095935974,13.6225644812608));
#88247=CARTESIAN_POINT('Ctrl Pts',(2.91493105778971,-9.50821677494992,13.6186554573556));
#88248=CARTESIAN_POINT('Ctrl Pts',(2.68041917906492,-9.57696976610555,13.6147464334504));
#88249=CARTESIAN_POINT('Ctrl Pts',(2.44371241810416,-9.63699297590299,13.6108374095452));
#88250=CARTESIAN_POINT('Ctrl Pts',(2.20695360059577,-9.6970293860039,13.6069275259675));
#88251=CARTESIAN_POINT('Ctrl Pts',(1.96799920791167,-9.74833210865252,13.6030176423898));
#88252=CARTESIAN_POINT('Ctrl Pts',(1.72750959691687,-9.79076476035249,13.5991077588121));
#88253=CARTESIAN_POINT('Ctrl Pts',(1.55591623018638,-9.82104116827872,13.5963179913712));
#88254=CARTESIAN_POINT('Ctrl Pts',(1.38354153945845,-9.84680282601728,13.5935282239303));
#88255=CARTESIAN_POINT('Ctrl Pts',(1.21062803919123,-9.86801620138131,13.5907384564895));
#88256=CARTESIAN_POINT('Ctrl Pts',(0.96828866000674,-9.89774688295436,13.5868285795357));
#88257=CARTESIAN_POINT('Ctrl Pts',(0.724816478307781,-9.91855072316058,
13.5829187025819));
#88258=CARTESIAN_POINT('Ctrl Pts',(0.48088239469076,-9.93036334292338,13.5790088256282));
#88259=CARTESIAN_POINT('Ctrl Pts',(0.236990538295991,-9.9421739178136,13.5750996255099));
#88260=CARTESIAN_POINT('Ctrl Pts',(-0.00736278055499909,-9.94499636575971,
13.5711904253916));
#88261=CARTESIAN_POINT('Ctrl Pts',(-0.251503636338526,-9.93881833624644,
13.5672812252733));
#88262=CARTESIAN_POINT('Ctrl Pts',(-0.49561791380746,-9.93264097930234,
13.5633724507288));
#88263=CARTESIAN_POINT('Ctrl Pts',(-0.739519494277679,-9.91746510839929,
13.5594636761843));
#88264=CARTESIAN_POINT('Ctrl Pts',(-0.982535498819007,-9.89333048035698,
13.5555549016399));
#88265=CARTESIAN_POINT('Ctrl Pts',(-1.22557036264081,-9.86919397934454,
13.5516458237545));
#88266=CARTESIAN_POINT('Ctrl Pts',(-1.46771923394983,-9.83609735660985,
13.5477367458692));
#88267=CARTESIAN_POINT('Ctrl Pts',(-1.70831410082192,-9.79413227054511,
13.5438276679839));
#88268=CARTESIAN_POINT('Ctrl Pts',(-1.94890564534161,-9.75216776397237,
13.5399186440787));
#88269=CARTESIAN_POINT('Ctrl Pts',(-2.18794295253656,-9.70133508919492,
13.5360096201735));
#88270=CARTESIAN_POINT('Ctrl Pts',(-2.42476722548671,-9.64177721699716,
13.5321005962683));
#88271=CARTESIAN_POINT('Ctrl Pts',(-2.66164358082723,-9.58220624683308,
13.5281907126906));
#88272=CARTESIAN_POINT('Ctrl Pts',(-2.89630565723214,-9.51390631248867,
13.5242808291129));
#88273=CARTESIAN_POINT('Ctrl Pts',(-3.12810752025186,-9.43707090901323,
13.5203709455352));
#88274=CARTESIAN_POINT('Ctrl Pts',(-3.29350203324386,-9.3822475612937,13.5175811780943));
#88275=CARTESIAN_POINT('Ctrl Pts',(-3.45744066278369,-9.32307981029869,
13.5147914106534));
#88276=CARTESIAN_POINT('Ctrl Pts',(-3.61969405072859,-9.25965328611823,
13.5120016432125));
#88277=CARTESIAN_POINT('Ctrl Pts',(-3.84709321415005,-9.17076060584786,
13.5080917662588));
#88278=CARTESIAN_POINT('Ctrl Pts',(-4.07125104332576,-9.07347355302008,
13.504181889305));
#88279=CARTESIAN_POINT('Ctrl Pts',(-4.29154651074866,-8.96805399995345,
13.5002720123512));
#88280=CARTESIAN_POINT('Ctrl Pts',(-4.51180384301016,-8.86265269597618,
13.4963628122329));
#88281=CARTESIAN_POINT('Ctrl Pts',(-4.72819989548968,-8.74912182300618,
13.4924536121146));
#88282=CARTESIAN_POINT('Ctrl Pts',(-4.94013568073457,-8.62777048002166,
13.4885444119964));
#88283=CARTESIAN_POINT('Ctrl Pts',(-5.15204839365958,-8.50643234791137,
13.4846356374519));
#88284=CARTESIAN_POINT('Ctrl Pts',(-5.359501565704,-8.37727558493515,13.4807268629074));
#88285=CARTESIAN_POINT('Ctrl Pts',(-5.5619218702263,-8.24065465296892,13.4768180883629));
#88286=CARTESIAN_POINT('Ctrl Pts',(-5.76435788359565,-8.10402311852223,
13.4729090104775));
#88287=CARTESIAN_POINT('Ctrl Pts',(-5.96176001492486,-7.9599264118996,13.4689999325922));
#88288=CARTESIAN_POINT('Ctrl Pts',(-6.15358386304595,-7.80876236291389,
13.4650908547069));
#88289=CARTESIAN_POINT('Ctrl Pts',(-6.34540506228902,-7.65760040133873,
13.4611818308017));
#88290=CARTESIAN_POINT('Ctrl Pts',(-6.53164791347946,-7.49937146771238,
13.4572728068964));
#88291=CARTESIAN_POINT('Ctrl Pts',(-6.71180048787439,-7.33451417688786,
13.4533637829912));
#88292=CARTESIAN_POINT('Ctrl Pts',(-6.89199268142085,-7.16962063065036,
13.4494538994135));
#88293=CARTESIAN_POINT('Ctrl Pts',(-7.06609171432072,-6.99809600303789,
13.4455440158358));
#88294=CARTESIAN_POINT('Ctrl Pts',(-7.23362096621123,-6.82041726855397,
13.4416341322581));
#88295=CARTESIAN_POINT('Ctrl Pts',(-7.35315589430491,-6.69364051458034,
13.4388443648172));
#88296=CARTESIAN_POINT('Ctrl Pts',(-7.46934684466363,-6.56373146921644,
13.4360545973764));
#88297=CARTESIAN_POINT('Ctrl Pts',(-7.58203261433193,-6.43087439118561,
13.4332648299355));
#88298=CARTESIAN_POINT('Ctrl Pts',(-7.73996244295911,-6.24467434456856,
13.4293549529818));
#88299=CARTESIAN_POINT('Ctrl Pts',(-7.89105405542264,-6.05262532043193,
13.425445076028));
#88300=CARTESIAN_POINT('Ctrl Pts',(-8.03488521642281,-5.85525264688982,
13.4215351990742));
#88301=CARTESIAN_POINT('Ctrl Pts',(-8.17869147893296,-5.65791414036345,
13.4176259989559));
#88302=CARTESIAN_POINT('Ctrl Pts',(-8.3152396339323,-5.45525405052717,13.4137167988376));
#88303=CARTESIAN_POINT('Ctrl Pts',(-8.44414926606862,-5.24782880554929,
13.4098075987193));
#88304=CARTESIAN_POINT('Ctrl Pts',(-8.57304486449993,-5.04042614185295,
13.4058988241748));
#88305=CARTESIAN_POINT('Ctrl Pts',(-8.69430345253167,-4.82825959679366,
13.4019900496303));
#88306=CARTESIAN_POINT('Ctrl Pts',(-8.80758873651319,-4.61191333921682,
13.3980812750858));
#88307=CARTESIAN_POINT('Ctrl Pts',(-8.92088281200999,-4.39555029206798,
13.3941721972005));
#88308=CARTESIAN_POINT('Ctrl Pts',(-9.02620221428049,-4.17500713117138,
13.3902631193152));
#88309=CARTESIAN_POINT('Ctrl Pts',(-9.12325669743927,-3.95089246027141,
13.3863540414298));
#88310=CARTESIAN_POINT('Ctrl Pts',(-9.22030984038136,-3.72678088415093,
13.3824450175246));
#88311=CARTESIAN_POINT('Ctrl Pts',(-9.3090981829599,-3.49909815472667,13.3785359936194));
#88312=CARTESIAN_POINT('Ctrl Pts',(-9.38937942241948,-3.26847335339386,
13.3746269697142));
#88313=CARTESIAN_POINT('Ctrl Pts',(-9.46967831732807,-3.03779783305806,
13.3707170861365));
#88314=CARTESIAN_POINT('Ctrl Pts',(-9.54146627763864,-2.80417921246332,
13.3668072025588));
#88315=CARTESIAN_POINT('Ctrl Pts',(-9.60455028812226,-2.56826356959923,
13.3628973189811));
#88316=CARTESIAN_POINT('Ctrl Pts',(-9.6495617865438,-2.39993380576549,13.3601075515403));
#88317=CARTESIAN_POINT('Ctrl Pts',(-9.69014308115675,-2.23043496936777,
13.3573177840994));
#88318=CARTESIAN_POINT('Ctrl Pts',(-9.72623977981077,-2.06000576349351,
13.3545280166586));
#88319=CARTESIAN_POINT('Ctrl Pts',(-9.77790824323873,-1.81605505555838,
13.350534770673));
#88320=CARTESIAN_POINT('Ctrl Pts',(-9.82039913593903,-1.57013722047607,
13.3465415246875));
#88321=CARTESIAN_POINT('Ctrl Pts',(-9.85358736138807,-1.3229437295264,13.342548278702));
#88322=CARTESIAN_POINT('Ctrl Pts',(-9.88676782727094,-1.07580803359969,
13.3385559663566));
#88323=CARTESIAN_POINT('Ctrl Pts',(-9.91064993630569,-0.827397529053514,
13.3345636540111));
#88324=CARTESIAN_POINT('Ctrl Pts',(-9.92516018494209,-0.57841101583585,
13.3305713416656));
#88325=CARTESIAN_POINT('Ctrl Pts',(-9.93638033506975,-0.385880472213324,
13.3274842585291));
#88326=CARTESIAN_POINT('Ctrl Pts',(-9.94199783454639,-0.19300570929332,
13.3243971753925));
#88327=CARTESIAN_POINT('Ctrl Pts',(-9.94199999937389,-0.000111577862839334,
13.321310092256));
#88328=CARTESIAN_POINT('Ctrl Pts',(-9.94199999942951,-0.000106505970992509,
13.1786899088249));
#88329=CARTESIAN_POINT('Ctrl Pts',(-9.94199732858428,-0.249421572746613,
13.1826799425284));
#88330=CARTESIAN_POINT('Ctrl Pts',(-9.93261222415611,-0.498704725276454,
13.1866699762318));
#88331=CARTESIAN_POINT('Ctrl Pts',(-9.91387787977736,-0.747254564965084,
13.1906600099353));
#88332=CARTESIAN_POINT('Ctrl Pts',(-9.89513752219156,-0.995884182286508,
13.1946513243293));
#88333=CARTESIAN_POINT('Ctrl Pts',(-9.86704194641944,-1.24377976230886,
13.1986426387234));
#88334=CARTESIAN_POINT('Ctrl Pts',(-9.82967631540366,-1.49024411905982,
13.2026339531174));
#88335=CARTESIAN_POINT('Ctrl Pts',(-9.79980239131882,-1.6872930456546,13.2058250198802));
#88336=CARTESIAN_POINT('Ctrl Pts',(-9.76400401434294,-1.8834271732374,13.209016086643));
#88337=CARTESIAN_POINT('Ctrl Pts',(-9.72234836197068,-2.07829409095199,
13.2122071534058));
#88338=CARTESIAN_POINT('Ctrl Pts',(-9.6713094814617,-2.31705614992799,13.2161170303596));
#88339=CARTESIAN_POINT('Ctrl Pts',(-9.61146324235827,-2.55397371089278,
13.2200269073133));
#88340=CARTESIAN_POINT('Ctrl Pts',(-9.54296788786523,-2.7883916315993,13.2239367842671));
#88341=CARTESIAN_POINT('Ctrl Pts',(-9.47448439054498,-3.0227689724182,13.2278459843854));
#88342=CARTESIAN_POINT('Ctrl Pts',(-9.39735484524539,-3.25464726783933,
13.2317551845036));
#88343=CARTESIAN_POINT('Ctrl Pts',(-9.31178765908832,-3.48338550724012,
13.2356643846219));
#88344=CARTESIAN_POINT('Ctrl Pts',(-9.22622978817491,-3.71209884512747,
13.2395731591664));
#88345=CARTESIAN_POINT('Ctrl Pts',(-9.13223620864876,-3.93767254709915,
13.2434819337109));
#88346=CARTESIAN_POINT('Ctrl Pts',(-9.03006423638719,-4.15948360818035,
13.2473907082554));
#88347=CARTESIAN_POINT('Ctrl Pts',(-8.92788433505995,-4.38131188293015,
13.2512997861407));
#88348=CARTESIAN_POINT('Ctrl Pts',(-8.81752488726968,-4.59937667741979,
13.255208864026));
#88349=CARTESIAN_POINT('Ctrl Pts',(-8.69929067555455,-4.81307653608476,
13.2591179419113));
#88350=CARTESIAN_POINT('Ctrl Pts',(-8.58105809652494,-5.02677344378773,
13.2630269658165));
#88351=CARTESIAN_POINT('Ctrl Pts',(-8.45495110856853,-5.23610529192399,
13.2669359897218));
#88352=CARTESIAN_POINT('Ctrl Pts',(-8.32131998410183,-5.44049609155154,
13.270845013627));
#88353=CARTESIAN_POINT('Ctrl Pts',(-8.18765947148013,-5.64493184080084,
13.2747548972047));
#88354=CARTESIAN_POINT('Ctrl Pts',(-8.04647166857423,-5.84442413499898,
13.2786647807824));
#88355=CARTESIAN_POINT('Ctrl Pts',(-7.89815040162596,-6.03842564194473,
13.2825746643601));
#88356=CARTESIAN_POINT('Ctrl Pts',(-7.79232069260521,-6.17684896755466,
13.285364431801));
#88357=CARTESIAN_POINT('Ctrl Pts',(-7.68286020402429,-6.31247749867597,
13.2881541992419));
#88358=CARTESIAN_POINT('Ctrl Pts',(-7.56992477163206,-6.44512241558152,
13.2909439666829));
#88359=CARTESIAN_POINT('Ctrl Pts',(-7.41164503910113,-6.6310251170161,13.2948538436367));
#88360=CARTESIAN_POINT('Ctrl Pts',(-7.24648966419361,-6.81112288259956,
13.2987637205905));
#88361=CARTESIAN_POINT('Ctrl Pts',(-7.07490896788178,-6.98491425116916,
13.3026735975443));
#88362=CARTESIAN_POINT('Ctrl Pts',(-6.90335797375851,-7.15867553486259,
13.3065827976626));
#88363=CARTESIAN_POINT('Ctrl Pts',(-6.72538407543683,-7.32613240143615,
13.3104919977809));
#88364=CARTESIAN_POINT('Ctrl Pts',(-6.54147503382302,-7.48681964400573,
13.3144011978992));
#88365=CARTESIAN_POINT('Ctrl Pts',(-6.35758601340758,-7.64748939341059,
13.3183099724437));
#88366=CARTESIAN_POINT('Ctrl Pts',(-6.167763350815,-7.80139080594464,13.3222187469882));
#88367=CARTESIAN_POINT('Ctrl Pts',(-5.97252930289241,-7.94809774261059,
13.3261275215327));
#88368=CARTESIAN_POINT('Ctrl Pts',(-5.77728010381255,-8.09481606448262,
13.330036599418));
#88369=CARTESIAN_POINT('Ctrl Pts',(-5.5766189025228,-8.23433862398428,13.3339456773033));
#88370=CARTESIAN_POINT('Ctrl Pts',(-5.37109950009994,-8.36628078419714,
13.3378547551886));
#88371=CARTESIAN_POINT('Ctrl Pts',(-5.16558293567578,-8.49822112243272,
13.3417637790938));
#88372=CARTESIAN_POINT('Ctrl Pts',(-4.95520854130392,-8.62258112102101,
13.3456728029991));
#88373=CARTESIAN_POINT('Ctrl Pts',(-4.74055806269171,-8.73902015412762,
13.3495818269043));
#88374=CARTESIAN_POINT('Ctrl Pts',(-4.52586037814926,-8.85548479450474,
13.353491710482));
#88375=CARTESIAN_POINT('Ctrl Pts',(-4.30688497630831,-8.96402485403609,
13.3574015940597));
#88376=CARTESIAN_POINT('Ctrl Pts',(-4.08423832896597,-9.06434560639682,
13.3613114776374));
#88377=CARTESIAN_POINT('Ctrl Pts',(-3.92537621575494,-9.1359261440298,13.3641012450782));
#88378=CARTESIAN_POINT('Ctrl Pts',(-3.76464556609823,-9.20332314153561,
13.366891012519));
#88379=CARTESIAN_POINT('Ctrl Pts',(-3.60227317993511,-9.26644440641178,
13.3696807799599));
#88380=CARTESIAN_POINT('Ctrl Pts',(-3.37470723974289,-9.3549092638121,13.3735906569136));
#88381=CARTESIAN_POINT('Ctrl Pts',(-3.14384611613994,-9.4350007404964,13.3775005338674));
#88382=CARTESIAN_POINT('Ctrl Pts',(-2.91032422327388,-9.50649130412611,
13.3814104108212));
#88383=CARTESIAN_POINT('Ctrl Pts',(-2.67684275518445,-9.57796949208503,
13.3853196109395));
#88384=CARTESIAN_POINT('Ctrl Pts',(-2.44070170520027,-9.64084965714869,
13.3892288110578));
#88385=CARTESIAN_POINT('Ctrl Pts',(-2.20255122552143,-9.69495395032664,
13.393138011176));
#88386=CARTESIAN_POINT('Ctrl Pts',(-1.96442667201731,-9.74905235345825,
13.3970467857205));
#88387=CARTESIAN_POINT('Ctrl Pts',(-1.72429339884424,-9.79437673021801,
13.400955560265));
#88388=CARTESIAN_POINT('Ctrl Pts',(-1.48281336938402,-9.83079999346828,
13.4048643348095));
#88389=CARTESIAN_POINT('Ctrl Pts',(-1.24131459984261,-9.86722608334945,
13.4087734126948));
#88390=CARTESIAN_POINT('Ctrl Pts',(-0.998469141906446,-9.89474963458269,
13.4126824905802));
#88391=CARTESIAN_POINT('Ctrl Pts',(-0.754947016616046,-9.91329506279837,
13.4165915684655));
#88392=CARTESIAN_POINT('Ctrl Pts',(-0.511428254100723,-9.9318402349219,
13.4205005923707));
#88393=CARTESIAN_POINT('Ctrl Pts',(-0.267233122595606,-9.94140751275124,
13.4244096162759));
#88394=CARTESIAN_POINT('Ctrl Pts',(-0.0230353415490897,-9.94197331383663,
13.4283186401811));
#88395=CARTESIAN_POINT('Ctrl Pts',(0.221216143469949,-9.94253923935299,
13.4322285237588));
#88396=CARTESIAN_POINT('Ctrl Pts',(0.465469998774068,-9.93409973088492,
13.4361384073365));
#88397=CARTESIAN_POINT('Ctrl Pts',(0.709052535746479,-9.9166833418009,13.4400482909142));
#88398=CARTESIAN_POINT('Ctrl Pts',(0.882852756982974,-9.90425645638634,
13.4428380583551));
#88399=CARTESIAN_POINT('Ctrl Pts',(1.05631120637462,-9.88726047604474,13.445627825796));
#88400=CARTESIAN_POINT('Ctrl Pts',(1.22918450521996,-9.86572194277374,13.4484175932369));
#88401=CARTESIAN_POINT('Ctrl Pts',(1.47146754185372,-9.83553555030947,13.4523274701906));
#88402=CARTESIAN_POINT('Ctrl Pts',(1.71267513534455,-9.79641522475994,13.4562373471444));
#88403=CARTESIAN_POINT('Ctrl Pts',(1.95214090753327,-9.74846192366443,13.4601472240982));
#88404=CARTESIAN_POINT('Ctrl Pts',(2.1915652260052,-9.70051692372421,13.4640564242164));
#88405=CARTESIAN_POINT('Ctrl Pts',(2.42924805036886,-9.64374205561775,13.4679656243347));
#88406=CARTESIAN_POINT('Ctrl Pts',(2.66453274019601,-9.57828947549736,13.471874824453));
#88407=CARTESIAN_POINT('Ctrl Pts',(2.89979181583238,-9.51284402085069,13.4757835989975));
#88408=CARTESIAN_POINT('Ctrl Pts',(3.13265300825618,-9.43872281554012,13.479692373542));
#88409=CARTESIAN_POINT('Ctrl Pts',(3.36247338287568,-9.35612829911244,13.4836011480865));
#88410=CARTESIAN_POINT('Ctrl Pts',(3.59231159272715,-9.27352737292947,13.4875102259718));
#88411=CARTESIAN_POINT('Ctrl Pts',(3.81910824838988,-9.18245191359552,13.4914193038571));
#88412=CARTESIAN_POINT('Ctrl Pts',(4.04223777636832,-9.08315351402259,13.4953283817424));
#88413=CARTESIAN_POINT('Ctrl Pts',(4.26536422317144,-8.98385648565221,13.4992374056476));
#88414=CARTESIAN_POINT('Ctrl Pts',(4.48482338829301,-8.87633686000137,13.5031464295529));
#88415=CARTESIAN_POINT('Ctrl Pts',(4.700011132911,-8.76089375295196,13.5070554534581));
#88416=CARTESIAN_POINT('Ctrl Pts',(4.91524620161468,-8.64542525765611,13.5109653370358));
#88417=CARTESIAN_POINT('Ctrl Pts',(5.12620772520819,-8.52202993077017,13.5148752206135));
#88418=CARTESIAN_POINT('Ctrl Pts',(5.33231634522919,-8.3910527584089,13.5187851041911));
#88419=CARTESIAN_POINT('Ctrl Pts',(5.479378298863,-8.29759835147086,13.521574871632));
#88420=CARTESIAN_POINT('Ctrl Pts',(5.62397012744568,-8.20028493965103,13.5243646390729));
#88421=CARTESIAN_POINT('Ctrl Pts',(5.76589023444149,-8.0992514348162,13.5271544065137));
#88422=CARTESIAN_POINT('Ctrl Pts',(5.96479217425593,-7.95765233005725,13.5310642834675));
#88423=CARTESIAN_POINT('Ctrl Pts',(6.1585059299626,-7.80870104983866,13.5349741604213));
#88424=CARTESIAN_POINT('Ctrl Pts',(6.34649295335573,-7.65280283249256,13.5388840373751));
#88425=CARTESIAN_POINT('Ctrl Pts',(6.53444743447464,-7.49693160255467,13.5427932374934));
#88426=CARTESIAN_POINT('Ctrl Pts',(6.71667694657671,-7.33411601495616,13.5467024376116));
#88427=CARTESIAN_POINT('Ctrl Pts',(6.89267581991407,-7.16480174474995,13.5506116377299));
#88428=CARTESIAN_POINT('Ctrl Pts',(7.06865553319191,-6.99550590688613,13.5545204122744));
#88429=CARTESIAN_POINT('Ctrl Pts',(7.23840576011248,-6.81971299327947,13.558429186819));
#88430=CARTESIAN_POINT('Ctrl Pts',(7.40145676719534,-6.63790642622645,13.5623379613635));
#88431=CARTESIAN_POINT('Ctrl Pts',(7.564520427867,-6.45608575005762,13.5662470392488));
#88432=CARTESIAN_POINT('Ctrl Pts',(7.72088364040559,-6.26825069455036,13.5701561171341));
#88433=CARTESIAN_POINT('Ctrl Pts',(7.87011528808262,-6.07491969924609,13.5740651950194));
#88434=CARTESIAN_POINT('Ctrl Pts',(8.01934487503333,-5.88159137363204,13.5779742189247));
#88435=CARTESIAN_POINT('Ctrl Pts',(8.16144292442014,-5.68276748317503,13.5818832428299));
#88436=CARTESIAN_POINT('Ctrl Pts',(8.29601974734786,-5.47899811567903,13.5857922667351));
#88437=CARTESIAN_POINT('Ctrl Pts',(8.43062616640853,-5.27518393522667,13.5897021503128));
#88438=CARTESIAN_POINT('Ctrl Pts',(8.55770789852269,-5.06642233795103,13.5936120338905));
#88439=CARTESIAN_POINT('Ctrl Pts',(8.67691884248351,-4.85329201686387,13.5975219174682));
#88440=CARTESIAN_POINT('Ctrl Pts',(8.76197784832004,-4.70121996187494,13.6003116849091));
#88441=CARTESIAN_POINT('Ctrl Pts',(8.84303069884756,-4.54692436104982,13.6031014523499));
#88442=CARTESIAN_POINT('Ctrl Pts',(8.91996592148114,-4.39062318579209,13.6058912197908));
#88443=CARTESIAN_POINT('Ctrl Pts',(9.02779112923973,-4.17156608660955,13.6098010967445));
#88444=CARTESIAN_POINT('Ctrl Pts',(9.1275595110882,-3.94850158245876,13.6137109736983));
#88445=CARTESIAN_POINT('Ctrl Pts',(9.21898948979115,-3.72204201845175,13.6176208506521));
#88446=CARTESIAN_POINT('Ctrl Pts',(9.310403641128,-3.49562165666787,13.6215300507704));
#88447=CARTESIAN_POINT('Ctrl Pts',(9.39348216588967,-3.26580766803928,13.6254392508887));
#88448=CARTESIAN_POINT('Ctrl Pts',(9.46799162194494,-3.03323237599435,13.629348451007));
#88449=CARTESIAN_POINT('Ctrl Pts',(9.54249296655266,-2.80068240318251,13.6332572255515));
#88450=CARTESIAN_POINT('Ctrl Pts',(9.60842701960371,-2.56537199401636,13.637166000096));
#88451=CARTESIAN_POINT('Ctrl Pts',(9.66560988833804,-2.32794963142717,13.6410747746405));
#88452=CARTESIAN_POINT('Ctrl Pts',(9.72279719475438,-2.09050884365275,13.6449838525258));
#88453=CARTESIAN_POINT('Ctrl Pts',(9.77123189118644,-1.8509560467701,13.6488929304111));
#88454=CARTESIAN_POINT('Ctrl Pts',(9.81078069718854,-1.60995220788467,13.6528020082964));
#88455=CARTESIAN_POINT('Ctrl Pts',(9.85032895706476,-1.36895169699941,13.6567110322016));
#88456=CARTESIAN_POINT('Ctrl Pts',(9.88099152855776,-1.12650046114897,13.6606200561068));
#88457=CARTESIAN_POINT('Ctrl Pts',(9.90268661803924,-0.883267651907685,
13.6645290800121));
#88458=CARTESIAN_POINT('Ctrl Pts',(9.92438647870449,-0.639981350910512,
13.6684389635898));
#88459=CARTESIAN_POINT('Ctrl Pts',(9.93711489079659,-0.395913412295458,
13.6723488471675));
#88460=CARTESIAN_POINT('Ctrl Pts',(9.94084200360668,-0.151737468441802,
13.6762587307452));
#88461=CARTESIAN_POINT('Ctrl Pts',(9.94350136104263,0.0224861585459037,
13.679048498186));
#88462=CARTESIAN_POINT('Ctrl Pts',(9.94157918780769,0.196764677770003,13.6818382656269));
#88463=CARTESIAN_POINT('Ctrl Pts',(9.93508086580521,0.370853326682132,13.6846280330678));
#88464=CARTESIAN_POINT('Ctrl Pts',(9.92597342585754,0.614839684226999,13.6885379100215));
#88465=CARTESIAN_POINT('Ctrl Pts',(9.90787250252161,0.858527721690995,13.6924477869753));
#88466=CARTESIAN_POINT('Ctrl Pts',(9.88082101026709,1.10124482430766,13.6963576639291));
#88467=CARTESIAN_POINT('Ctrl Pts',(9.85377420087345,1.34391991037255,13.7002668640474));
#88468=CARTESIAN_POINT('Ctrl Pts',(9.81777994659825,1.58562411866262,13.7041760641657));
#88469=CARTESIAN_POINT('Ctrl Pts',(9.77293301111777,1.82569010519433,13.7080852642839));
#88470=CARTESIAN_POINT('Ctrl Pts',(9.72809095788426,2.06572995702092,13.7119940388284));
#88471=CARTESIAN_POINT('Ctrl Pts',(9.67439819918634,2.3041316677469,13.7159028133729));
#88472=CARTESIAN_POINT('Ctrl Pts',(9.6120007794975,2.54023719659,13.7198115879174));
#88473=CARTESIAN_POINT('Ctrl Pts',(9.54959851745092,2.7763610484253,13.7237206658027));
#88474=CARTESIAN_POINT('Ctrl Pts',(9.47849031324122,3.010188090503,13.7276297436881));
#88475=CARTESIAN_POINT('Ctrl Pts',(9.39887268265288,3.2410733245765,13.7315388215734));
#88476=CARTESIAN_POINT('Ctrl Pts',(9.31925615149717,3.4719553703768,13.7354478454786));
#88477=CARTESIAN_POINT('Ctrl Pts',(9.23113052230889,3.69989542507572,13.7393568693838));
#88478=CARTESIAN_POINT('Ctrl Pts',(9.13474151040695,3.92426573234384,13.743265893289));
#88479=CARTESIAN_POINT('Ctrl Pts',(9.03833130063493,4.14868538312664,13.7471757768667));
#88480=CARTESIAN_POINT('Ctrl Pts',(8.93365418667395,4.36953345974712,13.7510856604444));
#88481=CARTESIAN_POINT('Ctrl Pts',(8.82100372635553,4.58620292394721,13.7549955440221));
#88482=CARTESIAN_POINT('Ctrl Pts',(8.74062573551506,4.74080021684468,13.757785311463));
#88483=CARTESIAN_POINT('Ctrl Pts',(8.6561894655125,4.8932705855102,13.7605750789039));
#88484=CARTESIAN_POINT('Ctrl Pts',(8.56781586218746,5.04340116901768,13.7633648463447));
#88485=CARTESIAN_POINT('Ctrl Pts',(8.44395969055799,5.25381014430122,13.7672747232985));
#88486=CARTESIAN_POINT('Ctrl Pts',(8.31232996790528,5.4596866100354,13.7711846002523));
#88487=CARTESIAN_POINT('Ctrl Pts',(8.17328380974075,5.66045897126989,13.7750944772061));
#88488=CARTESIAN_POINT('Ctrl Pts',(8.0342617217387,5.86119657697125,13.7790036773243));
#88489=CARTESIAN_POINT('Ctrl Pts',(7.88782592060099,6.05683161164373,13.7829128774426));
#88490=CARTESIAN_POINT('Ctrl Pts',(7.73437665198203,6.24682173631321,13.7868220775609));
#88491=CARTESIAN_POINT('Ctrl Pts',(7.58094408856781,6.43679117776955,13.7907308521054));
#88492=CARTESIAN_POINT('Ctrl Pts',(7.42049975823215,6.62111671825914,13.7946396266499));
#88493=CARTESIAN_POINT('Ctrl Pts',(7.25348462198825,6.79928855385473,13.7985484011944));
#88494=CARTESIAN_POINT('Ctrl Pts',(7.08645652451837,6.97747421649305,13.8024574790797));
#88495=CARTESIAN_POINT('Ctrl Pts',(6.91285679168171,7.14950501336379,13.806366556965));
#88496=CARTESIAN_POINT('Ctrl Pts',(6.73316461204516,7.31490658225399,13.8102756348504));
#88497=CARTESIAN_POINT('Ctrl Pts',(6.55347491376161,7.48030586712894,13.8141846587556));
#88498=CARTESIAN_POINT('Ctrl Pts',(6.36769314458791,7.63907591877233,13.8180936826608));
#88499=CARTESIAN_POINT('Ctrl Pts',(6.17633360755374,7.79078090875377,13.822002706566));
#88500=CARTESIAN_POINT('Ctrl Pts',(5.984931986733,7.94251926169437,13.8259125901437));
#88501=CARTESIAN_POINT('Ctrl Pts',(5.78795036609402,8.08718927332352,13.8298224737214));
#88502=CARTESIAN_POINT('Ctrl Pts',(5.58593531839025,8.22439606407428,13.8337323572991));
#88503=CARTESIAN_POINT('Ctrl Pts',(5.44179419719196,8.32229540810648,13.83652212474));
#88504=CARTESIAN_POINT('Ctrl Pts',(5.29509120226131,8.416396036642,13.8393118921808));
#88505=CARTESIAN_POINT('Ctrl Pts',(5.14603384120027,8.50656803330354,13.8421016596217));
#88506=CARTESIAN_POINT('Ctrl Pts',(4.93712899405436,8.63294466472467,13.8460115365754));
#88507=CARTESIAN_POINT('Ctrl Pts',(4.72353458475188,8.75164146899247,13.8499214135292));
#88508=CARTESIAN_POINT('Ctrl Pts',(4.50583629543146,8.86232493642455,13.853831290483));
#88509=CARTESIAN_POINT('Ctrl Pts',(4.28817569167732,8.97298924353544,13.8577404906013));
#88510=CARTESIAN_POINT('Ctrl Pts',(4.06641287580908,9.07564285596153,13.8616496907195));
#88511=CARTESIAN_POINT('Ctrl Pts',(3.84115759866413,9.16999848976132,13.8655588908378));
#88512=CARTESIAN_POINT('Ctrl Pts',(3.61592684386145,9.2643438515658,13.8694676653823));
#88513=CARTESIAN_POINT('Ctrl Pts',(3.38720464537551,9.35039293019713,13.8733764399268));
#88514=CARTESIAN_POINT('Ctrl Pts',(3.15562114063591,9.42790640687378,13.8772852144713));
#88515=CARTESIAN_POINT('Ctrl Pts',(2.92401966383604,9.50542589899128,13.8811942923566));
#88516=CARTESIAN_POINT('Ctrl Pts',(2.68955670193747,9.57440837365301,13.885103370242));
#88517=CARTESIAN_POINT('Ctrl Pts',(2.45287920940057,9.63466385423438,13.8890124481273));
#88518=CARTESIAN_POINT('Ctrl Pts',(2.21620498512208,9.69491850275318,13.8929214720325));
#88519=CARTESIAN_POINT('Ctrl Pts',(1.97731656353752,9.74644633104595,13.8968304959377));
#88520=CARTESIAN_POINT('Ctrl Pts',(1.73687350823564,9.78910794793832,13.9007395198429));
#88521=CARTESIAN_POINT('Ctrl Pts',(1.49637757470016,9.83177894697293,13.9046494034206));
#88522=CARTESIAN_POINT('Ctrl Pts',(1.2543266002188,9.86557978848229,13.9085592869983));
#88523=CARTESIAN_POINT('Ctrl Pts',(1.01138910720584,9.89042244162631,13.912469170576));
#88524=CARTESIAN_POINT('Ctrl Pts',(0.83804913564136,9.90814809087116,13.9152589380169));
#88525=CARTESIAN_POINT('Ctrl Pts',(0.664258019571988,9.92131414527852,13.9180487054578));
#88526=CARTESIAN_POINT('Ctrl Pts',(0.490260069134454,9.9299047862813,13.9208384728987));
#88527=CARTESIAN_POINT('Ctrl Pts',(0.24640082608494,9.94194462472182,13.9247483498524));
#88528=CARTESIAN_POINT('Ctrl Pts',(0.00206054199615485,9.94499890041736,
13.9286582268062));
#88529=CARTESIAN_POINT('Ctrl Pts',(-0.242086977851291,9.93905216281486,
13.93256810376));
#88530=CARTESIAN_POINT('Ctrl Pts',(-0.486192233529097,9.93310645464706,
13.9364773038783));
#88531=CARTESIAN_POINT('Ctrl Pts',(-0.730104511488564,9.91816285043836,
13.9403865039966));
#88532=CARTESIAN_POINT('Ctrl Pts',(-0.973150770741514,9.89425801045259,
13.9442957041149));
#88533=CARTESIAN_POINT('Ctrl Pts',(-1.21617057084281,9.87035577285941,13.9482044786594));
#88534=CARTESIAN_POINT('Ctrl Pts',(-1.45832426162404,9.83749427479848,13.9521132532039));
#88535=CARTESIAN_POINT('Ctrl Pts',(-1.69894363286851,9.79576207001454,13.9560220277484));
#88536=CARTESIAN_POINT('Ctrl Pts',(-1.93958167740217,9.75402662659888,13.9599311056337));
#88537=CARTESIAN_POINT('Ctrl Pts',(-2.17868488774455,9.70341914576131,13.963840183519));
#88538=CARTESIAN_POINT('Ctrl Pts',(-2.41559367980634,9.64407959185736,13.9677492614043));
#88539=CARTESIAN_POINT('Ctrl Pts',(-2.65249920041627,9.58474085736789,13.9716582853095));
#88540=CARTESIAN_POINT('Ctrl Pts',(-2.88721009192215,9.51667036108228,13.9755673092148));
#88541=CARTESIAN_POINT('Ctrl Pts',(-3.11907969004316,9.44005857435007,13.97947633312));
#88542=CARTESIAN_POINT('Ctrl Pts',(-3.35100028092263,9.36342993915489,13.9833862166977));
#88543=CARTESIAN_POINT('Ctrl Pts',(-3.58007806326531,9.27825634717285,13.9872961002754));
#88544=CARTESIAN_POINT('Ctrl Pts',(-3.80568287314214,9.18477772562149,13.9912059838531));
#88545=CARTESIAN_POINT('Ctrl Pts',(-3.9666556848868,9.1180791629563,13.9939957512939));
#88546=CARTESIAN_POINT('Ctrl Pts',(-4.12586072983799,9.04715349288656,13.9967855187348));
#88547=CARTESIAN_POINT('Ctrl Pts',(-4.2830754796054,8.97210278786434,13.9995752861756));
#88548=CARTESIAN_POINT('Ctrl Pts',(-4.50341295931952,8.86691874362021,14.0034851631294));
#88549=CARTESIAN_POINT('Ctrl Pts',(-4.71990760785364,8.75359809155419,14.0073950400832));
#88550=CARTESIAN_POINT('Ctrl Pts',(-4.93195907173468,8.63244714520361,14.0113049170369));
#88551=CARTESIAN_POINT('Ctrl Pts',(-5.14397382756636,8.51131717119078,14.0152141171552));
#88552=CARTESIAN_POINT('Ctrl Pts',(-5.3515466908855,8.38235974775502,14.0191233172735));
#88553=CARTESIAN_POINT('Ctrl Pts',(-5.55410272222934,8.24592668842773,14.0230325173918));
#88554=CARTESIAN_POINT('Ctrl Pts',(-5.75663670237712,8.10950848184078,14.0269412919362));
#88555=CARTESIAN_POINT('Ctrl Pts',(-5.95415470864457,7.96561642085906,14.0308500664807));
#88556=CARTESIAN_POINT('Ctrl Pts',(-6.14611069131068,7.81464569703301,14.0347588410252));
#88557=CARTESIAN_POINT('Ctrl Pts',(-6.33808157073958,7.66366325710919,14.0386679189105));
#88558=CARTESIAN_POINT('Ctrl Pts',(-6.52448934182446,7.50560122753885,14.0425769967958));
#88559=CARTESIAN_POINT('Ctrl Pts',(-6.70481995562998,7.34089595094399,14.0464860746812));
#88560=CARTESIAN_POINT('Ctrl Pts',(-6.88514807926637,7.17619294874941,14.0503950985864));
#88561=CARTESIAN_POINT('Ctrl Pts',(-7.05939900786311,7.00484707357558,14.0543041224916));
#88562=CARTESIAN_POINT('Ctrl Pts',(-7.22709404312832,6.82733298527172,14.0582131463968));
#88563=CARTESIAN_POINT('Ctrl Pts',(-7.39482595788342,6.64977985807195,14.0621230299745));
#88564=CARTESIAN_POINT('Ctrl Pts',(-7.55599890510002,6.46605601035547,14.0660329135522));
#88565=CARTESIAN_POINT('Ctrl Pts',(-7.71017218931807,6.27667179411718,14.0699427971299));
#88566=CARTESIAN_POINT('Ctrl Pts',(-7.82017741070618,6.14154298279056,14.0727325645708));
#88567=CARTESIAN_POINT('Ctrl Pts',(-7.92661985514808,6.00353318953445,14.0755223320117));
#88568=CARTESIAN_POINT('Ctrl Pts',(-8.02935213713319,5.86283790138485,14.0783120994526));
#88569=CARTESIAN_POINT('Ctrl Pts',(-8.17333208895841,5.66565255303689,14.0822219764063));
#88570=CARTESIAN_POINT('Ctrl Pts',(-8.31006682801636,5.46313066739559,14.0861318533601));
#88571=CARTESIAN_POINT('Ctrl Pts',(-8.43917341423532,5.25582686971933,14.0900417303139));
#88572=CARTESIAN_POINT('Ctrl Pts',(-8.56825765092245,5.04855895822799,14.0939509304322));
#88573=CARTESIAN_POINT('Ctrl Pts',(-8.68971622268014,4.83651102498496,14.0978601305505));
#88574=CARTESIAN_POINT('Ctrl Pts',(-8.80321015901934,4.62026567376148,14.1017693306688));
#88575=CARTESIAN_POINT('Ctrl Pts',(-8.91669173987867,4.40404386401669,14.1056781052133));
#88576=CARTESIAN_POINT('Ctrl Pts',(-9.02221028635632,4.18362579678211,14.1095868797578));
#88577=CARTESIAN_POINT('Ctrl Pts',(-9.11947284906762,3.95961853656617,14.1134956543023));
#88578=CARTESIAN_POINT('Ctrl Pts',(-9.21674295984921,3.73559389224583,14.1174047321876));
#88579=CARTESIAN_POINT('Ctrl Pts',(-9.30575569214927,3.507979754281,14.121313810073));
#88580=CARTESIAN_POINT('Ctrl Pts',(-9.38626579840765,3.2774042109027,14.1252228879583));
#88581=CARTESIAN_POINT('Ctrl Pts',(-9.46677479290924,3.04683185152128,14.1291319118635));
#88582=CARTESIAN_POINT('Ctrl Pts',(-9.53878130572673,2.81329843385258,14.1330409357688));
#88583=CARTESIAN_POINT('Ctrl Pts',(-9.60208939388073,2.57744898531923,14.136949959674));
#88584=CARTESIAN_POINT('Ctrl Pts',(-9.66541140474864,2.34154766877827,14.1408598432517));
#88585=CARTESIAN_POINT('Ctrl Pts',(-9.72003109486963,2.10332957419767,14.1447697268294));
#88586=CARTESIAN_POINT('Ctrl Pts',(-9.7658029136977,1.86345309863528,14.1486796104071));
#88587=CARTESIAN_POINT('Ctrl Pts',(-9.79846187331522,1.69229721431242,14.1514693778479));
#88588=CARTESIAN_POINT('Ctrl Pts',(-9.82661738093914,1.5202973177943,14.1542591452887));
#88589=CARTESIAN_POINT('Ctrl Pts',(-9.8502325362061,1.34769543394151,14.1570489127296));
#88590=CARTESIAN_POINT('Ctrl Pts',(-9.88482225034695,1.09488109691296,14.1611351555345));
#88591=CARTESIAN_POINT('Ctrl Pts',(-9.90967623294466,0.840722795474834,
14.1652213983395));
#88592=CARTESIAN_POINT('Ctrl Pts',(-9.92471777929082,0.585953071012211,
14.1693076411444));
#88593=CARTESIAN_POINT('Ctrl Pts',(-9.93622988735837,0.390964036450559,
14.1724350635303));
#88594=CARTESIAN_POINT('Ctrl Pts',(-9.94199523718629,0.195617028572116,
14.1755624859161));
#88595=CARTESIAN_POINT('Ctrl Pts',(-9.9419999970495,0.000242214229054161,
14.178689908302));
#88596=CARTESIAN_POINT('Origin',(0.,0.,0.));
#88597=CARTESIAN_POINT('',(-9.94207718462978,-3.49168275919068E-5,15.3213100916858));
#88598=CARTESIAN_POINT('',(-9.9420751122847,-4.12289121522736E-5,15.1786899083142));
#88599=CARTESIAN_POINT('',(-9.942,-1.2175438477123E-15,0.));
#88600=CARTESIAN_POINT('Ctrl Pts',(-9.94199999993869,-3.49165565174472E-5,
15.3213100916858));
#88601=CARTESIAN_POINT('Ctrl Pts',(-9.94200085662577,0.243894721467326,
15.3174038606442));
#88602=CARTESIAN_POINT('Ctrl Pts',(-9.93302005102662,0.487862969434573,
15.3134976296025));
#88603=CARTESIAN_POINT('Ctrl Pts',(-9.91507511453682,0.731197287394158,
15.3095913985609));
#88604=CARTESIAN_POINT('Ctrl Pts',(-9.89713332233784,0.974488968598745,
15.3056858519645));
#88605=CARTESIAN_POINT('Ctrl Pts',(-9.87023055529752,1.21714666105488,15.3017803053682));
#88606=CARTESIAN_POINT('Ctrl Pts',(-9.8344363552134,1.45850113995739,15.2978747587718));
#88607=CARTESIAN_POINT('Ctrl Pts',(-9.79864602746684,1.69982950831646,15.2939696346906));
#88608=CARTESIAN_POINT('Ctrl Pts',(-9.75396622853532,1.93985466640253,15.2900645106095));
#88609=CARTESIAN_POINT('Ctrl Pts',(-9.70051809299003,2.17791476591096,15.2861593865283));
#88610=CARTESIAN_POINT('Ctrl Pts',(-9.64706588965377,2.41599298352052,15.2822539652389));
#88611=CARTESIAN_POINT('Ctrl Pts',(-9.58484407510101,2.65210556853956,15.2783485439495));
#88612=CARTESIAN_POINT('Ctrl Pts',(-9.51402470257343,2.88560183650179,15.27444312266));
#88613=CARTESIAN_POINT('Ctrl Pts',(-9.44320579862831,3.11909655951593,15.2705377272112));
#88614=CARTESIAN_POINT('Ctrl Pts',(-9.36378953438648,3.34997473150565,15.2666323317623));
#88615=CARTESIAN_POINT('Ctrl Pts',(-9.27599776630388,3.57760107327877,15.2627269363134));
#88616=CARTESIAN_POINT('Ctrl Pts',(-9.18818719966375,3.80527615591877,15.2588207046153));
#88617=CARTESIAN_POINT('Ctrl Pts',(-9.09199764660268,4.02969775428937,15.2549144729171));
#88618=CARTESIAN_POINT('Ctrl Pts',(-8.98769952200388,4.25024955763438,15.251008241219));
#88619=CARTESIAN_POINT('Ctrl Pts',(-8.92720783120775,4.37816702061652,15.2487426725813));
#88620=CARTESIAN_POINT('Ctrl Pts',(-8.86398942047525,4.50478311840303,15.2464771039436));
#88621=CARTESIAN_POINT('Ctrl Pts',(-8.798104277811,4.62998111408283,15.2442115353059));
#88622=CARTESIAN_POINT('Ctrl Pts',(-8.68440090259071,4.84604552715019,15.2403016583521));
#88623=CARTESIAN_POINT('Ctrl Pts',(-8.56271709935375,5.05795247620724,15.2363917813984));
#88624=CARTESIAN_POINT('Ctrl Pts',(-8.43338237923258,5.26511402019458,15.2324819044446));
#88625=CARTESIAN_POINT('Ctrl Pts',(-8.3040700481352,5.47223970262259,15.2285727043263));
#88626=CARTESIAN_POINT('Ctrl Pts',(-8.16710959241722,5.67462138216799,15.224663504208));
#88627=CARTESIAN_POINT('Ctrl Pts',(-8.02287499666421,5.87169828822125,15.2207543040897));
#88628=CARTESIAN_POINT('Ctrl Pts',(-7.87865610296278,6.06875373956228,15.2168455295452));
#88629=CARTESIAN_POINT('Ctrl Pts',(-7.7271648158754,6.26050534438171,15.2129367550007));
#88630=CARTESIAN_POINT('Ctrl Pts',(-7.5688173374294,6.44642289278543,15.2090279804562));
#88631=CARTESIAN_POINT('Ctrl Pts',(-7.41045757041219,6.63235486933829,15.2051189025708));
#88632=CARTESIAN_POINT('Ctrl Pts',(-7.24524072827637,6.81245166938742,15.2012098246855));
#88633=CARTESIAN_POINT('Ctrl Pts',(-7.07362288382047,6.98621666551299,15.1973007468002));
#88634=CARTESIAN_POINT('Ctrl Pts',(-6.90200740922004,7.15997926213325,15.1933917228949));
#88635=CARTESIAN_POINT('Ctrl Pts',(-6.72399130753356,7.32741003169691,15.1894826989897));
#88636=CARTESIAN_POINT('Ctrl Pts',(-6.54006755990517,7.48804916596279,15.1855736750845));
#88637=CARTESIAN_POINT('Ctrl Pts',(-6.35610336376876,7.64872362798484,15.1816637915068));
#88638=CARTESIAN_POINT('Ctrl Pts',(-6.16622913619626,7.80260328498453,15.177753907929));
#88639=CARTESIAN_POINT('Ctrl Pts',(-5.97097204008465,7.94926769561369,15.1738440243513));
#88640=CARTESIAN_POINT('Ctrl Pts',(-5.83165283057599,8.05391520988496,15.1710542569105));
#88641=CARTESIAN_POINT('Ctrl Pts',(-5.6895938845075,8.15489022091912,15.1682644894697));
#88642=CARTESIAN_POINT('Ctrl Pts',(-5.54499629222769,8.25205308509229,15.1654747220289));
#88643=CARTESIAN_POINT('Ctrl Pts',(-5.34234183961776,8.38822746215193,15.1615648450752));
#88644=CARTESIAN_POINT('Ctrl Pts',(-5.13463768644058,8.51695386885005,15.1576549681214));
#88645=CARTESIAN_POINT('Ctrl Pts',(-4.92245298101037,8.63787130314767,15.1537450911676));
#88646=CARTESIAN_POINT('Ctrl Pts',(-4.71030500669503,8.75876780553054,15.1498358910494));
#88647=CARTESIAN_POINT('Ctrl Pts',(-4.49367827187,8.87185789530211,15.1459266909311));
#88648=CARTESIAN_POINT('Ctrl Pts',(-4.27316816597247,8.97682559846851,15.1420174908128));
#88649=CARTESIAN_POINT('Ctrl Pts',(-4.05268206583625,9.08178187435987,15.1381087162683));
#88650=CARTESIAN_POINT('Ctrl Pts',(-3.82831369174776,9.17861740875552,15.1341999417239));
#88651=CARTESIAN_POINT('Ctrl Pts',(-3.60068107910359,9.26706316837138,15.1302911671794));
#88652=CARTESIAN_POINT('Ctrl Pts',(-3.37303080100701,9.35551579182955,15.1263820892941));
#88653=CARTESIAN_POINT('Ctrl Pts',(-3.14211603835447,9.43557723512077,15.1224730114088));
#88654=CARTESIAN_POINT('Ctrl Pts',(-2.90857397250981,9.50702695096835,15.1185639335235));
#88655=CARTESIAN_POINT('Ctrl Pts',(-2.67503513162568,9.57847568017349,15.1146549096182));
#88656=CARTESIAN_POINT('Ctrl Pts',(-2.43886932877706,9.64131283973038,15.110745885713));
#88657=CARTESIAN_POINT('Ctrl Pts',(-2.20072874732272,9.69536781049112,15.1068368618078));
#88658=CARTESIAN_POINT('Ctrl Pts',(-1.96253579399613,9.74943466902002,15.1029269782301));
#88659=CARTESIAN_POINT('Ctrl Pts',(-1.72236746751696,9.79471541647667,15.0990170946524));
#88660=CARTESIAN_POINT('Ctrl Pts',(-1.48088734394482,9.83109030955082,15.0951072110747));
#88661=CARTESIAN_POINT('Ctrl Pts',(-1.30858722989211,9.85704440520316,15.0923174436338));
#88662=CARTESIAN_POINT('Ctrl Pts',(-1.1356195102959,9.87846553942996,15.0895276761929));
#88663=CARTESIAN_POINT('Ctrl Pts',(-0.962227465787131,9.89532628588289,
15.086737908752));
#88664=CARTESIAN_POINT('Ctrl Pts',(-0.719217403783887,9.91895673013168,
15.0828280317982));
#88665=CARTESIAN_POINT('Ctrl Pts',(-0.475299260203229,9.93363468164528,
15.0789181548444));
#88666=CARTESIAN_POINT('Ctrl Pts',(-0.231145341779765,9.93931264378848,
15.0750082778907));
#88667=CARTESIAN_POINT('Ctrl Pts',(0.0129663113656991,9.94498962302446,
15.0710990777724));
#88668=CARTESIAN_POINT('Ctrl Pts',(0.257313377781516,9.94166971645738,15.0671898776541));
#88669=CARTESIAN_POINT('Ctrl Pts',(0.5012218344231,9.9293575156048,15.0632806775358));
#88670=CARTESIAN_POINT('Ctrl Pts',(0.745103738049442,9.91704665511598,15.0593719029914));
#88671=CARTESIAN_POINT('Ctrl Pts',(0.988546847393906,9.8957454691014,15.0554631284469));
#88672=CARTESIAN_POINT('Ctrl Pts',(1.23087949531634,9.86551061364843,15.0515543539024));
#88673=CARTESIAN_POINT('Ctrl Pts',(1.4732309494886,9.83527341181642,15.0476452760171));
#88674=CARTESIAN_POINT('Ctrl Pts',(1.71447149148974,9.79610118686422,15.0437361981318));
#88675=CARTESIAN_POINT('Ctrl Pts',(1.95393562411819,9.74810235773106,15.0398271202465));
#88676=CARTESIAN_POINT('Ctrl Pts',(2.1933964500083,9.70010419140935,15.0359180963413));
#88677=CARTESIAN_POINT('Ctrl Pts',(2.43108064112902,9.6432797217921,15.0320090724361));
#88678=CARTESIAN_POINT('Ctrl Pts',(2.66633320203375,9.57778843239568,15.0281000485309));
#88679=CARTESIAN_POINT('Ctrl Pts',(2.90163749967821,9.51228274015585,15.0241901649532));
#88680=CARTESIAN_POINT('Ctrl Pts',(3.13450882813705,9.43810649385022,15.0202802813755));
#88681=CARTESIAN_POINT('Ctrl Pts',(3.36430632022437,9.35546936202019,15.0163703977978));
#88682=CARTESIAN_POINT('Ctrl Pts',(3.52827068097552,9.29650638391392,15.0135806303569));
#88683=CARTESIAN_POINT('Ctrl Pts',(3.69067042796834,9.23323696641594,15.010790862916));
#88684=CARTESIAN_POINT('Ctrl Pts',(3.85127842770058,9.1657524771471,15.008001095475));
#88685=CARTESIAN_POINT('Ctrl Pts',(4.07637156899041,9.07117253279072,15.0040912185213));
#88686=CARTESIAN_POINT('Ctrl Pts',(4.29801341969897,8.96828233382643,15.0001813415675));
#88687=CARTESIAN_POINT('Ctrl Pts',(4.51558973027739,8.85735927846519,14.9962714646138));
#88688=CARTESIAN_POINT('Ctrl Pts',(4.73312837640567,8.74645542489976,14.9923622644955));
#88689=CARTESIAN_POINT('Ctrl Pts',(4.9466026377054,8.62752161806375,14.9884530643772));
#88690=CARTESIAN_POINT('Ctrl Pts',(5.15542148469268,8.50088191396452,14.9845438642589));
#88691=CARTESIAN_POINT('Ctrl Pts',(5.36421759868521,8.37425599645481,14.9806350897144));
#88692=CARTESIAN_POINT('Ctrl Pts',(5.56835907071416,8.23992600199358,14.9767263151699));
#88693=CARTESIAN_POINT('Ctrl Pts',(5.76728166413054,8.09826069020896,14.9728175406254));
#88694=CARTESIAN_POINT('Ctrl Pts',(5.96621969495306,7.9565843844748,14.96890846274));
#88695=CARTESIAN_POINT('Ctrl Pts',(6.1599378077519,7.80757178404671,14.9649993848547));
#88696=CARTESIAN_POINT('Ctrl Pts',(6.34790177220379,7.6516342757905,14.9610903069694));
#88697=CARTESIAN_POINT('Ctrl Pts',(6.53586314107918,7.4956989208605,14.9571812830642));
#88698=CARTESIAN_POINT('Ctrl Pts',(6.71807030609076,7.33283902992702,14.9532722591589));
#88699=CARTESIAN_POINT('Ctrl Pts',(6.8940225241547,7.16350594586531,14.9493632352537));
#88700=CARTESIAN_POINT('Ctrl Pts',(7.07001343762662,6.99413562207542,14.945453351676));
#88701=CARTESIAN_POINT('Ctrl Pts',(7.23974645274272,6.81828945432251,14.9415434680983));
#88702=CARTESIAN_POINT('Ctrl Pts',(7.40275708775905,6.6364562455902,14.9376335845206));
#88703=CARTESIAN_POINT('Ctrl Pts',(7.51906790700664,6.50671520463325,14.9348438170798));
#88704=CARTESIAN_POINT('Ctrl Pts',(7.63195707931439,6.37392690775254,14.9320540496389));
#88705=CARTESIAN_POINT('Ctrl Pts',(7.74126808372366,6.23827960706488,14.929264282198));
#88706=CARTESIAN_POINT('Ctrl Pts',(7.8944681572043,6.04816904550609,14.9253544052442));
#88707=CARTESIAN_POINT('Ctrl Pts',(8.04068516920822,5.85238322265478,14.9214445282905));
#88708=CARTESIAN_POINT('Ctrl Pts',(8.17951022117169,5.65145791294139,14.9175346513367));
#88709=CARTESIAN_POINT('Ctrl Pts',(8.31831124124791,5.45056738523832,14.9136254512184));
#88710=CARTESIAN_POINT('Ctrl Pts',(8.44972269642412,5.24453937720431,14.9097162511001));
#88711=CARTESIAN_POINT('Ctrl Pts',(8.57337827652759,5.03393970241648,14.9058070509818));
#88712=CARTESIAN_POINT('Ctrl Pts',(8.69702039490751,4.82336295449209,14.9018982764373));
#88713=CARTESIAN_POINT('Ctrl Pts',(8.81290818221483,4.60821577517653,14.8979895018928));
#88714=CARTESIAN_POINT('Ctrl Pts',(8.92072013326175,4.38909060102641,14.8940807273483));
#88715=CARTESIAN_POINT('Ctrl Pts',(9.02854045106496,4.1699484216472,14.8901716494629));
#88716=CARTESIAN_POINT('Ctrl Pts',(9.12828355377994,3.94682788074227,14.8862625715776));
#88717=CARTESIAN_POINT('Ctrl Pts',(9.21967458357322,3.72034468470515,14.8823534936923));
#88718=CARTESIAN_POINT('Ctrl Pts',(9.3110643513558,3.4938646161546,14.8784444697871));
#88719=CARTESIAN_POINT('Ctrl Pts',(9.39410217389248,3.26402224607422,14.8745354458819));
#88720=CARTESIAN_POINT('Ctrl Pts',(9.46856163601043,3.03145254705917,14.8706264219767));
#88721=CARTESIAN_POINT('Ctrl Pts',(9.5430374732524,2.79883170131868,14.866716538399));
#88722=CARTESIAN_POINT('Ctrl Pts',(9.60893109396079,2.56348259491659,14.8628066548213));
#88723=CARTESIAN_POINT('Ctrl Pts',(9.66606578210403,2.32605595290345,14.8588967712436));
#88724=CARTESIAN_POINT('Ctrl Pts',(9.70683233935735,2.15664806586246,14.8561070038027));
#88725=CARTESIAN_POINT('Ctrl Pts',(9.74314070936392,1.9861828222507,14.8533172363619));
#88726=CARTESIAN_POINT('Ctrl Pts',(9.77494251660834,1.81490021681704,14.8505274689211));
#88727=CARTESIAN_POINT('Ctrl Pts',(9.81951295334562,1.57484654719376,14.8466175919673));
#88728=CARTESIAN_POINT('Ctrl Pts',(9.85524305899185,1.33311350729371,14.8427077150135));
#88729=CARTESIAN_POINT('Ctrl Pts',(9.88202733768561,1.09036677188656,14.8387978380597));
#88730=CARTESIAN_POINT('Ctrl Pts',(9.90880697977562,0.847662058160643,14.8348886379414));
#88731=CARTESIAN_POINT('Ctrl Pts',(9.92664385555036,0.603944277707854,14.8309794378232));
#88732=CARTESIAN_POINT('Ctrl Pts',(9.93548421339401,0.359885322566067,14.8270702377049));
#88733=CARTESIAN_POINT('Ctrl Pts',(9.94432360883498,0.115852936822927,14.8231614631604));
#88734=CARTESIAN_POINT('Ctrl Pts',(9.94416843175336,-0.128520269429035,
14.8192526886159));
#88735=CARTESIAN_POINT('Ctrl Pts',(9.93501700366949,-0.372560245863747,
14.8153439140714));
#88736=CARTESIAN_POINT('Ctrl Pts',(9.9258648653882,-0.616619161043476,14.8114348361861));
#88737=CARTESIAN_POINT('Ctrl Pts',(9.9077150884957,-0.860344514487166,14.8075257583008));
#88738=CARTESIAN_POINT('Ctrl Pts',(9.88061809710591,-1.10306392341661,14.8036166804155));
#88739=CARTESIAN_POINT('Ctrl Pts',(9.85352147989596,-1.34577998065622,14.7997076565102));
#88740=CARTESIAN_POINT('Ctrl Pts',(9.817477928441,-1.58748984279357,14.795798632605));
#88741=CARTESIAN_POINT('Ctrl Pts',(9.77258964864251,-1.82752717059015,14.7918896086998));
#88742=CARTESIAN_POINT('Ctrl Pts',(9.72769149701424,-2.06761728739204,14.7879797251221));
#88743=CARTESIAN_POINT('Ctrl Pts',(9.67394478089711,-2.30603385904891,14.7840698415444));
#88744=CARTESIAN_POINT('Ctrl Pts',(9.61150292554344,-2.54212027887545,14.7801599579667));
#88745=CARTESIAN_POINT('Ctrl Pts',(9.56694961556588,-2.71057189493409,14.7773701905259));
#88746=CARTESIAN_POINT('Ctrl Pts',(9.51797062780309,-2.87783741968628,14.774580423085));
#88747=CARTESIAN_POINT('Ctrl Pts',(9.46463733237617,-3.04368266522501,14.7717906556441));
#88748=CARTESIAN_POINT('Ctrl Pts',(9.3898903769119,-3.27611584009292,14.7678807786904));
#88749=CARTESIAN_POINT('Ctrl Pts',(9.30656568547299,-3.50582979009426,14.7639709017366));
#88750=CARTESIAN_POINT('Ctrl Pts',(9.21488646225104,-3.73218856541607,14.7600610247828));
#88751=CARTESIAN_POINT('Ctrl Pts',(9.12322310954175,-3.95850815596207,14.7561518246646));
#88752=CARTESIAN_POINT('Ctrl Pts',(9.02320821725878,-4.18147347157733,14.7522426245463));
#88753=CARTESIAN_POINT('Ctrl Pts',(8.91511348169699,-4.40046765792734,14.748333424428));
#88754=CARTESIAN_POINT('Ctrl Pts',(8.8070305138338,-4.61943800354575,14.7444246498835));
#88755=CARTESIAN_POINT('Ctrl Pts',(8.69086958300992,-4.83443783183178,14.740515875339));
#88756=CARTESIAN_POINT('Ctrl Pts',(8.56694923994434,-5.04487311240005,14.7366071007946));
#88757=CARTESIAN_POINT('Ctrl Pts',(8.44301928002809,-5.25532472381943,14.7326980229092));
#88758=CARTESIAN_POINT('Ctrl Pts',(8.31132884422128,-5.46121083658457,14.7287889450239));
#88759=CARTESIAN_POINT('Ctrl Pts',(8.17224154714889,-5.66196362537357,14.7248798671386));
#88760=CARTESIAN_POINT('Ctrl Pts',(8.03315617072061,-5.86271364198518,14.7209708432334));
#88761=CARTESIAN_POINT('Ctrl Pts',(7.8866742986526,-6.05833024713667,14.7170618193282));
#88762=CARTESIAN_POINT('Ctrl Pts',(7.73320224948501,-6.24827551957818,14.713152795423));
#88763=CARTESIAN_POINT('Ctrl Pts',(7.57969644874574,-6.43826256478231,14.7092429118453));
#88764=CARTESIAN_POINT('Ctrl Pts',(7.4191975746183,-6.62257556632651,14.7053330282676));
#88765=CARTESIAN_POINT('Ctrl Pts',(7.25215240307327,-6.80070948670788,14.7014231446899));
#88766=CARTESIAN_POINT('Ctrl Pts',(7.13296287441414,-6.92781102344842,14.698633377249));
#88767=CARTESIAN_POINT('Ctrl Pts',(7.01044143160265,-7.05176743943949,14.695843609808));
#88768=CARTESIAN_POINT('Ctrl Pts',(6.88476207621809,-7.17240651063987,14.6930538423671));
#88769=CARTESIAN_POINT('Ctrl Pts',(6.70862165391074,-7.34148294234961,14.6891439654134));
#88770=CARTESIAN_POINT('Ctrl Pts',(6.52622298655312,-7.50409360981867,14.6852340884596));
#88771=CARTESIAN_POINT('Ctrl Pts',(6.33806445520289,-7.65978478559899,14.6813242115058));
#88772=CARTESIAN_POINT('Ctrl Pts',(6.1499384958169,-7.81544900981153,14.6774150113875));
#88773=CARTESIAN_POINT('Ctrl Pts',(5.9560548787038,-7.9641959548582,14.6735058112693));
#88774=CARTESIAN_POINT('Ctrl Pts',(5.75694559673185,-8.105611722521,14.669596611151));
#88775=CARTESIAN_POINT('Ctrl Pts',(5.55785799072428,-8.24701209500426,14.6656878366065));
#88776=CARTESIAN_POINT('Ctrl Pts',(5.35354608419496,-8.38108272141112,14.6617790620619));
#88777=CARTESIAN_POINT('Ctrl Pts',(5.1445722702807,-8.50745203664757,14.6578702875174));
#88778=CARTESIAN_POINT('Ctrl Pts',(4.93558223893498,-8.633831158786,14.6539612096321));
#88779=CARTESIAN_POINT('Ctrl Pts',(4.72192981557315,-8.7525076278296,14.6500521317467));
#88780=CARTESIAN_POINT('Ctrl Pts',(4.50420461246357,-8.86315433742761,14.6461430538614));
#88781=CARTESIAN_POINT('Ctrl Pts',(4.28648241590132,-8.97379951911538,14.6422340299562));
#88782=CARTESIAN_POINT('Ctrl Pts',(4.06468780291554,-9.07641503795574,14.638325006051));
#88783=CARTESIAN_POINT('Ctrl Pts',(3.83943377164389,-9.17072038136375,14.6344159821457));
#88784=CARTESIAN_POINT('Ctrl Pts',(3.61413020250926,-9.26504646440137,14.630506098568));
#88785=CARTESIAN_POINT('Ctrl Pts',(3.38536595317184,-9.3510586109826,14.6265962149903));
#88786=CARTESIAN_POINT('Ctrl Pts',(3.15377401580106,-9.42852445811422,14.6226863314126));
#88787=CARTESIAN_POINT('Ctrl Pts',(2.98852928828094,-9.48379763794382,14.6198965639718));
#88788=CARTESIAN_POINT('Ctrl Pts',(2.82184538566737,-9.53472085093505,14.617106796531));
#88789=CARTESIAN_POINT('Ctrl Pts',(2.65395721633758,-9.58122513532845,14.6143170290901));
#88790=CARTESIAN_POINT('Ctrl Pts',(2.41866087067466,-9.64640118804924,14.6104071521364));
#88791=CARTESIAN_POINT('Ctrl Pts',(2.18092646501388,-9.70291539328969,14.6064972751826));
#88792=CARTESIAN_POINT('Ctrl Pts',(1.94140804813212,-9.75060504741361,14.6025873982288));
#88793=CARTESIAN_POINT('Ctrl Pts',(1.70193109407979,-9.79828644602207,14.5986781981105));
#88794=CARTESIAN_POINT('Ctrl Pts',(1.46067102007726,-9.83714628825954,14.5947689979922));
#88795=CARTESIAN_POINT('Ctrl Pts',(1.21829254648454,-9.86707288263243,14.5908597978739));
#88796=CARTESIAN_POINT('Ctrl Pts',(0.975940459346045,-9.89699621905629,
14.5869510233294));
#88797=CARTESIAN_POINT('Ctrl Pts',(0.732470493812973,-9.91798821507807,
14.5830422487849));
#88798=CARTESIAN_POINT('Ctrl Pts',(0.488554026534318,-9.92998887024337,
14.5791334742404));
#88799=CARTESIAN_POINT('Ctrl Pts',(0.244618630095396,-9.94199045672063,
14.5752243963551));
#88800=CARTESIAN_POINT('Ctrl Pts',(0.000236942509269006,-9.94499929121524,
14.5713153184698));
#88801=CARTESIAN_POINT('Ctrl Pts',(-0.243916812221935,-9.93900742472383,
14.5674062405845));
#88802=CARTESIAN_POINT('Ctrl Pts',(-0.48806719545689,-9.93301564097355,
14.5634972166792));
#88803=CARTESIAN_POINT('Ctrl Pts',(-0.731989371937555,-9.91802341375385,
14.559588192774));
#88804=CARTESIAN_POINT('Ctrl Pts',(-0.975010657646331,-9.89407490458184,
14.5556791688688));
#88805=CARTESIAN_POINT('Ctrl Pts',(-1.21808538859319,-9.87012112865399,
14.5517692852911));
#88806=CARTESIAN_POINT('Ctrl Pts',(-1.46025855371254,-9.83720716154928,
14.5478594017134));
#88807=CARTESIAN_POINT('Ctrl Pts',(-1.70086273281695,-9.79542903420338,
14.5439495181357));
#88808=CARTESIAN_POINT('Ctrl Pts',(-1.8725378458111,-9.76561964037036,14.5411597506948));
#88809=CARTESIAN_POINT('Ctrl Pts',(-2.04341428824949,-9.73129853269574,
14.538369983254));
#88810=CARTESIAN_POINT('Ctrl Pts',(-2.21325257474579,-9.69251654836767,
14.5355802158131));
#88811=CARTESIAN_POINT('Ctrl Pts',(-2.45128202211772,-9.63816334869736,
14.5316703388594));
#88812=CARTESIAN_POINT('Ctrl Pts',(-2.68734471051723,-9.57502928361011,
14.5277604619056));
#88813=CARTESIAN_POINT('Ctrl Pts',(-2.92078776089241,-9.50328168875474,
14.5238505849518));
#88814=CARTESIAN_POINT('Ctrl Pts',(-3.15419040013839,-9.43154651406489,
14.5199413848335));
#88815=CARTESIAN_POINT('Ctrl Pts',(-3.38497403880597,-9.35120086845111,
14.5160321847152));
#88816=CARTESIAN_POINT('Ctrl Pts',(-3.61250062547696,-9.26246205017481,
14.5121229845969));
#88817=CARTESIAN_POINT('Ctrl Pts',(-3.84000244254035,-9.173732892421,14.5082142100525));
#88818=CARTESIAN_POINT('Ctrl Pts',(-4.06424765453314,-9.07661248822245,
14.504305435508));
#88819=CARTESIAN_POINT('Ctrl Pts',(-4.28461689387056,-8.97136678955659,
14.5003966609635));
#88820=CARTESIAN_POINT('Ctrl Pts',(-4.5050032349847,-8.86611292328784,14.4964875830782));
#88821=CARTESIAN_POINT('Ctrl Pts',(-4.72151274811587,-8.75273262060444,
14.4925785051928));
#88822=CARTESIAN_POINT('Ctrl Pts',(-4.93354827288488,-8.63153899597949,
14.4886694273075));
#88823=CARTESIAN_POINT('Ctrl Pts',(-5.1455808696755,-8.51034704490577,14.4847604034023));
#88824=CARTESIAN_POINT('Ctrl Pts',(-5.35313935930901,-8.38134212857442,
14.480851379497));
#88825=CARTESIAN_POINT('Ctrl Pts',(-5.5556526779645,-8.24488249290588,14.4769423555918));
#88826=CARTESIAN_POINT('Ctrl Pts',(-5.75821053334468,-8.1083928470372,14.4730324720141));
#88827=CARTESIAN_POINT('Ctrl Pts',(-5.9557207675935,-7.96444536181786,14.4691225884364));
#88828=CARTESIAN_POINT('Ctrl Pts',(-6.14764157634337,-7.81344143440101,
14.4652127048587));
#88829=CARTESIAN_POINT('Ctrl Pts',(-6.2845802889253,-7.70569760219243,14.4624229374179));
#88830=CARTESIAN_POINT('Ctrl Pts',(-6.41867400228556,-7.59436219430257,
14.459633169977));
#88831=CARTESIAN_POINT('Ctrl Pts',(-6.54973608136025,-7.47959365637784,
14.4568434025362));
#88832=CARTESIAN_POINT('Ctrl Pts',(-6.73342042543229,-7.31874481468659,
14.4529335255824));
#88833=CARTESIAN_POINT('Ctrl Pts',(-6.91120480998141,-7.15110169481779,
14.4490236486286));
#88834=CARTESIAN_POINT('Ctrl Pts',(-7.08259408263102,-6.97712154549998,
14.4451137716748));
#88835=CARTESIAN_POINT('Ctrl Pts',(-7.25395368622958,-6.80317151373768,
14.4412045715565));
#88836=CARTESIAN_POINT('Ctrl Pts',(-7.41892019123506,-6.62288684197434,
14.4372953714382));
#88837=CARTESIAN_POINT('Ctrl Pts',(-7.57703521653304,-6.43676171125032,
14.4333861713199));
#88838=CARTESIAN_POINT('Ctrl Pts',(-7.73513302868985,-6.25065684297856,
14.4294773967754));
#88839=CARTESIAN_POINT('Ctrl Pts',(-7.88638066901632,-6.05871299882243,
14.4255686222309));
#88840=CARTESIAN_POINT('Ctrl Pts',(-8.03035930006934,-5.8614583093109,14.4216598476864));
#88841=CARTESIAN_POINT('Ctrl Pts',(-8.17434910459761,-5.66418831183059,
14.4177507698011));
#88842=CARTESIAN_POINT('Ctrl Pts',(-8.31106860489869,-5.46160687005948,
14.4138416919158));
#88843=CARTESIAN_POINT('Ctrl Pts',(-8.44014090012312,-5.25427307874923,
14.4099326140305));
#88844=CARTESIAN_POINT('Ctrl Pts',(-8.5692114129995,-5.04694215049318,14.4060235901253));
#88845=CARTESIAN_POINT('Ctrl Pts',(-8.69063478559525,-4.83485924301839,
14.4021145662201));
#88846=CARTESIAN_POINT('Ctrl Pts',(-8.80407851237586,-4.61861078116804,
14.3982055423149));
#88847=CARTESIAN_POINT('Ctrl Pts',(-8.91754718770018,-4.40231476195727,
14.3942956587372));
#88848=CARTESIAN_POINT('Ctrl Pts',(-9.02303257949188,-4.18185160573104,
14.3903857751595));
#88849=CARTESIAN_POINT('Ctrl Pts',(-9.12024842103068,-3.95783182294138,
14.3864758915818));
#88850=CARTESIAN_POINT('Ctrl Pts',(-9.18961355277154,-3.79798995458123,
14.3836861241409));
#88851=CARTESIAN_POINT('Ctrl Pts',(-9.25476957242055,-3.63633788958992,
14.3808963567001));
#88852=CARTESIAN_POINT('Ctrl Pts',(-9.31562744933931,-3.47310368764251,
14.3781065892592));
#88853=CARTESIAN_POINT('Ctrl Pts',(-9.40073229793138,-3.24483377838614,
14.3742053237587));
#88854=CARTESIAN_POINT('Ctrl Pts',(-9.47745710973565,-3.01339584872495,
14.3703040582581));
#88855=CARTESIAN_POINT('Ctrl Pts',(-9.54558346248208,-2.77942446574622,
14.3664027927576));
#88856=CARTESIAN_POINT('Ctrl Pts',(-9.61370093894827,-2.54548356723466,
14.3625020355585));
#88857=CARTESIAN_POINT('Ctrl Pts',(-9.67322211152418,-2.30901014511221,
14.3586012783594));
#88858=CARTESIAN_POINT('Ctrl Pts',(-9.72397841135791,-2.07065396806064,
14.3547005211603));
#88859=CARTESIAN_POINT('Ctrl Pts',(-9.77472803701372,-1.83232913355255,
14.3508002768896));
#88860=CARTESIAN_POINT('Ctrl Pts',(-9.8167150329033,-1.59212231511132,14.3469000326189));
#88861=CARTESIAN_POINT('Ctrl Pts',(-9.8498217594818,-1.35069437936156,14.3429997883482));
#88862=CARTESIAN_POINT('Ctrl Pts',(-9.88293073090551,-1.1092500732725,14.3390992796164));
#88863=CARTESIAN_POINT('Ctrl Pts',(-9.90715818883622,-0.866584764294565,
14.3351987708845));
#88864=CARTESIAN_POINT('Ctrl Pts',(-9.9224381093107,-0.623366639225106,
14.3312982621526));
#88865=CARTESIAN_POINT('Ctrl Pts',(-9.93548071998098,-0.415760891633932,
14.327968871997));
#88866=CARTESIAN_POINT('Ctrl Pts',(-9.94200503739041,-0.207752580076446,
14.3246394818414));
#88867=CARTESIAN_POINT('Ctrl Pts',(-9.94199999708083,0.000240924627958939,
14.3213100916858));
#88868=CARTESIAN_POINT('Ctrl Pts',(-9.94199999704952,0.000242213467125498,
14.1786899083142));
#88869=CARTESIAN_POINT('Ctrl Pts',(-9.94200593246289,-0.243385362018565,
14.1825897269062));
#88870=CARTESIAN_POINT('Ctrl Pts',(-9.93305242611158,-0.487033811773988,
14.1864895454982));
#88871=CARTESIAN_POINT('Ctrl Pts',(-9.91516094928765,-0.730032430595599,
14.1903893640902));
#88872=CARTESIAN_POINT('Ctrl Pts',(-9.89726842140917,-0.973045324639196,
14.1942894117814));
#88873=CARTESIAN_POINT('Ctrl Pts',(-9.87043689098207,-1.21540802900749,
14.1981894594725));
#88874=CARTESIAN_POINT('Ctrl Pts',(-9.83473984509367,-1.45645328772565,
14.2020895071637));
#88875=CARTESIAN_POINT('Ctrl Pts',(-9.7990438019972,-1.69749177506449,14.2059894452957));
#88876=CARTESIAN_POINT('Ctrl Pts',(-9.75448278445375,-1.93721261106689,
14.2098893834278));
#88877=CARTESIAN_POINT('Ctrl Pts',(-9.70118182189137,-2.17495638085099,
14.2137893215598));
#88878=CARTESIAN_POINT('Ctrl Pts',(-9.6478680282462,-2.41275738243441,14.2176901985198));
#88879=CARTESIAN_POINT('Ctrl Pts',(-9.58581014560736,-2.64858009013482,
14.2215910754797));
#88880=CARTESIAN_POINT('Ctrl Pts',(-9.51518406546778,-2.88177657015045,
14.2254919524396));
#88881=CARTESIAN_POINT('Ctrl Pts',(-9.45306052381708,-3.08689897267394,
14.2289232102953));
#88882=CARTESIAN_POINT('Ctrl Pts',(-9.38430840258609,-3.28998947716511,
14.2323544681509));
#88883=CARTESIAN_POINT('Ctrl Pts',(-9.30907916889128,-3.4906172845665,14.2357857260066));
#88884=CARTESIAN_POINT('Ctrl Pts',(-9.22335636418048,-3.7192302520094,14.2396956029604));
#88885=CARTESIAN_POINT('Ctrl Pts',(-9.12919493734013,-3.94471889634473,
14.2436054799141));
#88886=CARTESIAN_POINT('Ctrl Pts',(-9.02684810190686,-4.16645860955087,
14.2475153568679));
#88887=CARTESIAN_POINT('Ctrl Pts',(-8.92451898364727,-4.38815993758374,
14.2514245569862));
#88888=CARTESIAN_POINT('Ctrl Pts',(-8.81400740279905,-4.6061133756037,14.2553337571045));
#88889=CARTESIAN_POINT('Ctrl Pts',(-8.69561410139372,-4.81971569697246,
14.2592429572228));
#88890=CARTESIAN_POINT('Ctrl Pts',(-8.57723368883644,-5.03329476459433,
14.2631517317673));
#88891=CARTESIAN_POINT('Ctrl Pts',(-8.45097340479063,-5.24252341628112,
14.2670605063118));
#88892=CARTESIAN_POINT('Ctrl Pts',(-8.31717970653641,-5.44682345309437,
14.2709692808563));
#88893=CARTESIAN_POINT('Ctrl Pts',(-8.1833756252098,-5.65113934463098,14.2748783587416));
#88894=CARTESIAN_POINT('Ctrl Pts',(-8.04203711248208,-5.85052562082029,
14.278787436627));
#88895=CARTESIAN_POINT('Ctrl Pts',(-7.89355439149902,-6.04443240250452,
14.2826965145123));
#88896=CARTESIAN_POINT('Ctrl Pts',(-7.74507372090081,-6.23833650654704,
14.2866055384175));
#88897=CARTESIAN_POINT('Ctrl Pts',(-7.58944921142196,-6.4267610460982,14.2905145623227));
#88898=CARTESIAN_POINT('Ctrl Pts',(-7.4271123187362,-6.60918804429689,14.2944235862279));
#88899=CARTESIAN_POINT('Ctrl Pts',(-7.26473972492272,-6.7916551618391,14.2983334698056));
#88900=CARTESIAN_POINT('Ctrl Pts',(-7.09565198389764,-6.96812189232768,
14.3022433533833));
#88901=CARTESIAN_POINT('Ctrl Pts',(-6.92031939813261,-7.13810503059667,
14.306153236961));
#88902=CARTESIAN_POINT('Ctrl Pts',(-6.79521666057857,-7.25939084773495,
14.3089430044018));
#88903=CARTESIAN_POINT('Ctrl Pts',(-6.66693544661198,-7.37737655515681,
14.3117327718427));
#88904=CARTESIAN_POINT('Ctrl Pts',(-6.53565775611927,-7.49189840393462,
14.3145225392835));
#88905=CARTESIAN_POINT('Ctrl Pts',(-6.35167123126275,-7.65240150920476,
14.3184324162373));
#88906=CARTESIAN_POINT('Ctrl Pts',(-6.16174122976717,-7.80614837115737,
14.3223422931911));
#88907=CARTESIAN_POINT('Ctrl Pts',(-5.96638715909887,-7.95270949222591,
14.3262521701448));
#88908=CARTESIAN_POINT('Ctrl Pts',(-5.77106690600795,-8.09924524222316,
14.3301613702631));
#88909=CARTESIAN_POINT('Ctrl Pts',(-5.57032468222568,-8.23859756633971,
14.3340705703814));
#88910=CARTESIAN_POINT('Ctrl Pts',(-5.36471157364484,-8.37037835056463,
14.3379797704996));
#88911=CARTESIAN_POINT('Ctrl Pts',(-5.15912084906745,-8.50214478851782,
14.3418885450441));
#88912=CARTESIAN_POINT('Ctrl Pts',(-4.94866053437317,-8.62634118118867,
14.3457973195886));
#88913=CARTESIAN_POINT('Ctrl Pts',(-4.73391006682754,-8.74262314635538,
14.3497060941331));
#88914=CARTESIAN_POINT('Ctrl Pts',(-4.51914293355178,-8.85891413559488,
14.3536151720184));
#88915=CARTESIAN_POINT('Ctrl Pts',(-4.30008522719908,-8.96728933386437,
14.3575242499037));
#88916=CARTESIAN_POINT('Ctrl Pts',(-4.07734145772508,-9.06745006256535,
14.361433327789));
#88917=CARTESIAN_POINT('Ctrl Pts',(-3.85460076409937,-9.16760940815601,
14.3653423516942));
#88918=CARTESIAN_POINT('Ctrl Pts',(-3.62817436566829,-9.259554397956,14.3692513755994));
#88919=CARTESIAN_POINT('Ctrl Pts',(-3.39868791456105,-9.34303400718507,
14.3731603995047));
#88920=CARTESIAN_POINT('Ctrl Pts',(-3.16915099479696,-9.42653197524853,
14.3770702830823));
#88921=CARTESIAN_POINT('Ctrl Pts',(-2.93655294084078,-9.50156074592832,
14.38098016666));
#88922=CARTESIAN_POINT('Ctrl Pts',(-2.70153708496493,-9.5679183409224,14.3848900502377));
#88923=CARTESIAN_POINT('Ctrl Pts',(-2.53384933421917,-9.61526559674046,
14.3876798176786));
#88924=CARTESIAN_POINT('Ctrl Pts',(-2.36493103553926,-9.65819932922349,
14.3904695851195));
#88925=CARTESIAN_POINT('Ctrl Pts',(-2.19502011278984,-9.69666183304585,
14.3932593525605));
#88926=CARTESIAN_POINT('Ctrl Pts',(-1.95688886524821,-9.75056727873812,
14.3971692295142));
#88927=CARTESIAN_POINT('Ctrl Pts',(-1.71673450088251,-9.79570467238657,
14.401079106468));
#88928=CARTESIAN_POINT('Ctrl Pts',(-1.47521806992016,-9.83194261812899,
14.4049889834218));
#88929=CARTESIAN_POINT('Ctrl Pts',(-1.23374344766249,-9.86817429075132,
14.4088981835401));
#88930=CARTESIAN_POINT('Ctrl Pts',(-0.990907506561842,-9.89550954923249,
14.4128073836584));
#88931=CARTESIAN_POINT('Ctrl Pts',(-0.747379528884163,-9.91386845988007,
14.4167165837767));
#88932=CARTESIAN_POINT('Ctrl Pts',(-0.503878062801711,-9.93222537189074,
14.4206253583212));
#88933=CARTESIAN_POINT('Ctrl Pts',(-0.259684989979209,-9.94160786617101,
14.4245341328657));
#88934=CARTESIAN_POINT('Ctrl Pts',(-0.0154737816699827,-9.94198795825467,
14.4284429074102));
#88935=CARTESIAN_POINT('Ctrl Pts',(0.228756378674564,-9.94236807983541,
14.4323519852955));
#88936=CARTESIAN_POINT('Ctrl Pts',(0.473004396996434,-9.93374439971333,
14.4362610631809));
#88937=CARTESIAN_POINT('Ctrl Pts',(0.716596434826483,-9.91614106140055,
14.4401701410662));
#88938=CARTESIAN_POINT('Ctrl Pts',(0.960185108916133,-9.89853796617067,
14.4440791649714));
#88939=CARTESIAN_POINT('Ctrl Pts',(1.203117541179,-9.87195548300876,14.4479881888767));
#88940=CARTESIAN_POINT('Ctrl Pts',(1.44472391110842,-9.83646973363267,14.4518972127819));
#88941=CARTESIAN_POINT('Ctrl Pts',(1.68638341510737,-9.80097618023107,14.4558070963596));
#88942=CARTESIAN_POINT('Ctrl Pts',(1.92671599645829,-9.75657548794242,14.4597169799373));
#88943=CARTESIAN_POINT('Ctrl Pts',(2.16505956077095,-9.70339533865926,14.463626863515));
#88944=CARTESIAN_POINT('Ctrl Pts',(2.33512168723394,-9.66545041113922,14.4664166309558));
#88945=CARTESIAN_POINT('Ctrl Pts',(2.50417135425363,-9.6230368862643,14.4692063983967));
#88946=CARTESIAN_POINT('Ctrl Pts',(2.67197176687402,-9.57621693974338,14.4719961658375));
#88947=CARTESIAN_POINT('Ctrl Pts',(2.90714512094574,-9.51059848452723,14.4759060427912));
#88948=CARTESIAN_POINT('Ctrl Pts',(3.1399360992914,-9.4363027011379,14.479815919745));
#88949=CARTESIAN_POINT('Ctrl Pts',(3.36970052527757,-9.35352780345171,14.4837257966988));
#88950=CARTESIAN_POINT('Ctrl Pts',(3.59942517693956,-9.27076723485758,14.4876349968171));
#88951=CARTESIAN_POINT('Ctrl Pts',(3.82612405852349,-9.17953057701206,14.4915441969354));
#88952=CARTESIAN_POINT('Ctrl Pts',(4.04917018174472,-9.08006524421876,14.4954533970537));
#88953=CARTESIAN_POINT('Ctrl Pts',(4.27219202312241,-8.9806107396865,14.4993621715982));
#88954=CARTESIAN_POINT('Ctrl Pts',(4.49156164421777,-8.87292946297478,14.5032709461427));
#88955=CARTESIAN_POINT('Ctrl Pts',(4.70667303464128,-8.75731653790022,14.5071797206872));
#88956=CARTESIAN_POINT('Ctrl Pts',(4.92180111880482,-8.64169464067354,14.5110887985725));
#88957=CARTESIAN_POINT('Ctrl Pts',(5.13267006359735,-8.51813999513188,14.5149978764578));
#88958=CARTESIAN_POINT('Ctrl Pts',(5.33869828494419,-8.38699377741119,14.5189069543431));
#88959=CARTESIAN_POINT('Ctrl Pts',(5.54472366126592,-8.25584937067677,14.5228159782484));
#88960=CARTESIAN_POINT('Ctrl Pts',(5.74590821245473,-8.11711375369622,14.5267250021536));
#88961=CARTESIAN_POINT('Ctrl Pts',(5.94169856904823,-7.97117194109939,14.5306340260588));
#88962=CARTESIAN_POINT('Ctrl Pts',(6.13753198385399,-7.82519803298134,14.5345439096365));
#88963=CARTESIAN_POINT('Ctrl Pts',(6.32796860821824,-7.67201492936055,14.5384537932142));
#88964=CARTESIAN_POINT('Ctrl Pts',(6.51248635237282,-7.51204935488031,14.5423636767919));
#88965=CARTESIAN_POINT('Ctrl Pts',(6.64414285433088,-7.39791123734439,14.5451534442327));
#88966=CARTESIAN_POINT('Ctrl Pts',(6.77278667189828,-7.28032099449095,14.5479432116736));
#88967=CARTESIAN_POINT('Ctrl Pts',(6.89823892120813,-7.1594457736566,14.5507329791145));
#88968=CARTESIAN_POINT('Ctrl Pts',(7.07406105289956,-6.99003837671724,14.5546428560682));
#88969=CARTESIAN_POINT('Ctrl Pts',(7.2436665974382,-6.81412515296673,14.558552733022));
#88970=CARTESIAN_POINT('Ctrl Pts',(7.40658272194097,-6.63218639537863,14.5624626099758));
#88971=CARTESIAN_POINT('Ctrl Pts',(7.56947064417157,-6.45027913305461,14.5663718100941));
#88972=CARTESIAN_POINT('Ctrl Pts',(7.72567127109587,-6.26234862782928,14.5702810102123));
#88973=CARTESIAN_POINT('Ctrl Pts',(7.87475025689159,-6.06891031335823,14.5741902103306));
#88974=CARTESIAN_POINT('Ctrl Pts',(8.02381301325228,-5.87549305748602,14.5780989848751));
#88975=CARTESIAN_POINT('Ctrl Pts',(8.16575550545327,-5.67656941152785,14.5820077594196));
#88976=CARTESIAN_POINT('Ctrl Pts',(8.30018450206128,-5.4726868384498,14.5859165339641));
#88977=CARTESIAN_POINT('Ctrl Pts',(8.43462393104462,-5.26878844304489,14.5898256118494));
#88978=CARTESIAN_POINT('Ctrl Pts',(8.56154854244736,-5.05993058388463,14.5937346897347));
#88979=CARTESIAN_POINT('Ctrl Pts',(8.68060846738039,-4.8466896574924,14.5976437676201));
#88980=CARTESIAN_POINT('Ctrl Pts',(8.79966674822597,-4.63345167572433,14.6015527915253));
#88981=CARTESIAN_POINT('Ctrl Pts',(8.91086042494637,-4.41583099354175,14.6054618154305));
#88982=CARTESIAN_POINT('Ctrl Pts',(9.01388527419954,-4.19442919401064,14.6093708393357));
#88983=CARTESIAN_POINT('Ctrl Pts',(9.11693278067592,-3.9729787037993,14.6132807229134));
#88984=CARTESIAN_POINT('Ctrl Pts',(9.21180775077748,-3.74774568849631,14.6171906064911));
#88985=CARTESIAN_POINT('Ctrl Pts',(9.29825329372859,-3.51935358917877,14.6211004900688));
#88986=CARTESIAN_POINT('Ctrl Pts',(9.35993363697699,-3.35639199971779,14.6238902575097));
#88987=CARTESIAN_POINT('Ctrl Pts',(9.41732349670136,-3.1918225584054,14.6266800249506));
#88988=CARTESIAN_POINT('Ctrl Pts',(9.47034479553094,-3.0258773031569,14.6294697923914));
#88989=CARTESIAN_POINT('Ctrl Pts',(9.5446544857636,-2.79330396404026,14.6333796693452));
#88990=CARTESIAN_POINT('Ctrl Pts',(9.61040408220088,-2.55795636240189,14.637289546299));
#88991=CARTESIAN_POINT('Ctrl Pts',(9.66740547853949,-2.32048169859289,14.6411994232527));
#88992=CARTESIAN_POINT('Ctrl Pts',(9.72439700741507,-2.08304814382013,14.645108623371));
#88993=CARTESIAN_POINT('Ctrl Pts',(9.77264329387064,-1.84348853434929,14.6490178234893));
#88994=CARTESIAN_POINT('Ctrl Pts',(9.81200678838167,-1.60246272491815,14.6529270236077));
#88995=CARTESIAN_POINT('Ctrl Pts',(9.85136599759855,-1.36146315468411,14.6568357981521));
#88996=CARTESIAN_POINT('Ctrl Pts',(9.88184430053851,-1.11899797973397,14.6607445726966));
#88997=CARTESIAN_POINT('Ctrl Pts',(9.90335553954652,-0.875735723453872,
14.6646533472411));
#88998=CARTESIAN_POINT('Ctrl Pts',(9.92486844793628,-0.632454588783239,
14.6685624251264));
#88999=CARTESIAN_POINT('Ctrl Pts',(9.93741287412366,-0.38837652814623,14.6724715030118));
#89000=CARTESIAN_POINT('Ctrl Pts',(9.94095456111795,-0.144174941609904,
14.6763805808971));
#89001=CARTESIAN_POINT('Ctrl Pts',(9.9444961992054,0.100023272768773,14.6802896048023));
#89002=CARTESIAN_POINT('Ctrl Pts',(9.93903534473031,0.344344729305567,14.6841986287075));
#89003=CARTESIAN_POINT('Ctrl Pts',(9.92458987162252,0.588115532942081,14.6881076526127));
#89004=CARTESIAN_POINT('Ctrl Pts',(9.91014122166646,0.831939946650653,14.6920175361904));
#89005=CARTESIAN_POINT('Ctrl Pts',(9.88670402048512,1.07521318548938,14.6959274197681));
#89006=CARTESIAN_POINT('Ctrl Pts',(9.85434817734733,1.3172645898267,14.6998373033458));
#89007=CARTESIAN_POINT('Ctrl Pts',(9.83126174116239,1.48997232227285,14.7026270707866));
#89008=CARTESIAN_POINT('Ctrl Pts',(9.80363585762131,1.66205807871755,14.7054168382275));
#89009=CARTESIAN_POINT('Ctrl Pts',(9.77151197839084,1.83328057213408,14.7082066056684));
#89010=CARTESIAN_POINT('Ctrl Pts',(9.7264901557007,2.07324999437786,14.7121164826221));
#89011=CARTESIAN_POINT('Ctrl Pts',(9.67261739787909,2.31159686134554,14.7160263595759));
#89012=CARTESIAN_POINT('Ctrl Pts',(9.6100354321011,2.54766226053638,14.7199362365297));
#89013=CARTESIAN_POINT('Ctrl Pts',(9.54746429983418,2.78368679464603,14.7238454366479));
#89014=CARTESIAN_POINT('Ctrl Pts',(9.4761870410031,3.01743037855659,14.7277546367662));
#89015=CARTESIAN_POINT('Ctrl Pts',(9.39639588603101,3.24824696613103,14.7316638368845));
#89016=CARTESIAN_POINT('Ctrl Pts',(9.31661341749703,3.47903842593282,14.735572611429));
#89017=CARTESIAN_POINT('Ctrl Pts',(9.22831899501513,3.70690326080634,14.7394813859735));
#89018=CARTESIAN_POINT('Ctrl Pts',(9.13175419485938,3.9312121953245,14.743390160518));
#89019=CARTESIAN_POINT('Ctrl Pts',(9.03518190078283,4.15553853735955,14.7472992384033));
#89020=CARTESIAN_POINT('Ctrl Pts',(8.93033805457291,4.37630816893196,14.7512083162886));
#89021=CARTESIAN_POINT('Ctrl Pts',(8.81751222578281,4.59291216421245,14.7551173941739));
#89022=CARTESIAN_POINT('Ctrl Pts',(8.70468795499463,4.80951316842747,14.7590264180791));
#89023=CARTESIAN_POINT('Ctrl Pts',(8.58388205340214,5.02194840372532,14.7629354419844));
#89024=CARTESIAN_POINT('Ctrl Pts',(8.45543020613305,5.22963325953291,14.7668444658896));
#89025=CARTESIAN_POINT('Ctrl Pts',(8.32695010973508,5.43736378939177,14.7707543494673));
#89026=CARTESIAN_POINT('Ctrl Pts',(8.19082085439789,5.6403416132436,14.774664233045));
#89027=CARTESIAN_POINT('Ctrl Pts',(8.04742238556117,5.83800967354191,14.7785741166227));
#89028=CARTESIAN_POINT('Ctrl Pts',(7.94510517547423,5.97904914639744,14.7813638840636));
#89029=CARTESIAN_POINT('Ctrl Pts',(7.83908808971278,6.11738596196061,14.7841536515045));
#89030=CARTESIAN_POINT('Ctrl Pts',(7.7295221690902,6.25282744344853,14.7869434189454));
#89031=CARTESIAN_POINT('Ctrl Pts',(7.57596482890402,6.44264954807725,14.7908532958992));
#89032=CARTESIAN_POINT('Ctrl Pts',(7.41538811977392,6.62684135982234,14.7947631728529));
#89033=CARTESIAN_POINT('Ctrl Pts',(7.24822961692489,6.80489025777293,14.7986730498067));
#89034=CARTESIAN_POINT('Ctrl Pts',(7.08110005074217,6.98290833383016,14.802582249925));
#89035=CARTESIAN_POINT('Ctrl Pts',(6.90739115704458,7.15478541460849,14.8064914500433));
#89036=CARTESIAN_POINT('Ctrl Pts',(6.72757885036217,7.32004418102511,14.8104006501616));
#89037=CARTESIAN_POINT('Ctrl Pts',(6.54778611888903,7.48528495659898,14.8143094247061));
#89038=CARTESIAN_POINT('Ctrl Pts',(6.36189150742211,7.64390866680942,14.8182181992506));
#89039=CARTESIAN_POINT('Ctrl Pts',(6.17040639744928,7.79547618111408,14.8221269737951));
#89040=CARTESIAN_POINT('Ctrl Pts',(5.97890642725549,7.94705545783072,14.8260360516804));
#89041=CARTESIAN_POINT('Ctrl Pts',(5.78181530953639,8.09157726805006,14.8299451295657));
#89042=CARTESIAN_POINT('Ctrl Pts',(5.57967700313877,8.22864317738012,14.8338542074511));
#89043=CARTESIAN_POINT('Ctrl Pts',(5.3775414880496,8.36570719398021,14.8377632313563));
#89044=CARTESIAN_POINT('Ctrl Pts',(5.17035915684901,8.49531535998442,14.8416722552615));
#89045=CARTESIAN_POINT('Ctrl Pts',(4.95870301034087,8.61711253583452,14.8455812791668));
#89046=CARTESIAN_POINT('Ctrl Pts',(4.74700031641688,8.73893649731729,14.8494911627445));
#89047=CARTESIAN_POINT('Ctrl Pts',(4.53082208377621,8.85294589546851,14.8534010463222));
#89048=CARTESIAN_POINT('Ctrl Pts',(4.31076718511858,8.95883085428589,14.8573109298999));
#89049=CARTESIAN_POINT('Ctrl Pts',(4.15375432801763,9.03438154645112,14.8601006973407));
#89050=CARTESIAN_POINT('Ctrl Pts',(3.9947683775805,9.10579698298566,14.8628904647815));
#89051=CARTESIAN_POINT('Ctrl Pts',(3.83403374497742,9.17297930022599,14.8656802322223));
#89052=CARTESIAN_POINT('Ctrl Pts',(3.6087631268991,9.26713574855057,14.8695901091761));
#89053=CARTESIAN_POINT('Ctrl Pts',(3.37998791368454,9.35300428089725,14.8734999861299));
#89054=CARTESIAN_POINT('Ctrl Pts',(3.14833660037946,9.43034149173354,14.8774098630837));
#89055=CARTESIAN_POINT('Ctrl Pts',(2.91672538803731,9.50766531479066,14.8813190632019));
#89056=CARTESIAN_POINT('Ctrl Pts',(2.68223933523787,9.57646067574101,14.8852282633202));
#89057=CARTESIAN_POINT('Ctrl Pts',(2.445523918826,9.63653344115247,14.8891374634385));
#89058=CARTESIAN_POINT('Ctrl Pts',(2.20883427235932,9.69659966676228,14.893046237983));
#89059=CARTESIAN_POINT('Ctrl Pts',(1.96991601846588,9.74794512391848,14.8969550125275));
#89060=CARTESIAN_POINT('Ctrl Pts',(1.72942771726594,9.7904261281495,14.900863787072));
#89061=CARTESIAN_POINT('Ctrl Pts',(1.48892075294888,9.83291042912282,14.9047728649573));
#89062=CARTESIAN_POINT('Ctrl Pts',(1.24684377337754,9.86652885077642,14.9086819428426));
#89063=CARTESIAN_POINT('Ctrl Pts',(1.00386468823217,9.89118899261967,14.912591020728));
#89064=CARTESIAN_POINT('Ctrl Pts',(0.760888958364166,9.91584879393313,14.9165000446331));
#89065=CARTESIAN_POINT('Ctrl Pts',(0.51701142694094,9.93155053658849,14.9204090685384));
#89066=CARTESIAN_POINT('Ctrl Pts',(0.272905007874495,9.93825371263367,14.9243180924436));
#89067=CARTESIAN_POINT('Ctrl Pts',(0.0287449049263693,9.94495836284129,
14.9282279760213));
#89068=CARTESIAN_POINT('Ctrl Pts',(-0.215643905956332,9.94266048342952,
14.932137859599));
#89069=CARTESIAN_POINT('Ctrl Pts',(-0.459587231326087,9.93137168656989,
14.9360477431767));
#89070=CARTESIAN_POINT('Ctrl Pts',(-0.6336448811275,9.92331694087232,14.9388375106175));
#89071=CARTESIAN_POINT('Ctrl Pts',(-0.807475704560176,9.91068595367717,
14.9416272780584));
#89072=CARTESIAN_POINT('Ctrl Pts',(-0.980835732711074,9.89349914163018,
14.9444170454993));
#89073=CARTESIAN_POINT('Ctrl Pts',(-1.22380092358777,9.86941171436048,14.948326922453));
#89074=CARTESIAN_POINT('Ctrl Pts',(-1.46591555237888,9.83636614652125,14.9522367994068));
#89075=CARTESIAN_POINT('Ctrl Pts',(-1.70651091401231,9.79444661532018,14.9561466763606));
#89076=CARTESIAN_POINT('Ctrl Pts',(-1.9470646263869,9.75253434077357,14.9600558764788));
#89077=CARTESIAN_POINT('Ctrl Pts',(-2.18609932059487,9.70175121748677,14.9639650765971));
#89078=CARTESIAN_POINT('Ctrl Pts',(-2.42295473941667,9.64223284985061,14.9678742767154));
#89079=CARTESIAN_POINT('Ctrl Pts',(-2.65978437305416,9.58272096166123,14.97178305126));
#89080=CARTESIAN_POINT('Ctrl Pts',(-2.89443493325438,9.51447579616935,14.9756918258045));
#89081=CARTESIAN_POINT('Ctrl Pts',(-3.12625860050512,9.43768356975205,14.9796006003491));
#89082=CARTESIAN_POINT('Ctrl Pts',(-3.35810025845128,9.36088538386748,14.9835096782344));
#89083=CARTESIAN_POINT('Ctrl Pts',(-3.58711431801025,9.27553889690189,14.9874187561197));
#89084=CARTESIAN_POINT('Ctrl Pts',(-3.81266907988396,9.18187989941585,14.991327834005));
#89085=CARTESIAN_POINT('Ctrl Pts',(-4.0382207270906,9.08822219525917,14.9952368579102));
#89086=CARTESIAN_POINT('Ctrl Pts',(-4.26031291404368,8.98625231956187,14.9991458818154));
#89087=CARTESIAN_POINT('Ctrl Pts',(-4.47833417492712,8.87625410957121,15.0030549057206));
#89088=CARTESIAN_POINT('Ctrl Pts',(-4.69640338304489,8.7662317087749,15.0069647892984));
#89089=CARTESIAN_POINT('Ctrl Pts',(-4.91039962535968,8.64817757115304,15.0108746728761));
#89090=CARTESIAN_POINT('Ctrl Pts',(-5.11973505570604,8.5224220125135,15.0147845564538));
#89091=CARTESIAN_POINT('Ctrl Pts',(-5.26909939256813,8.43269331445298,15.0175743238946));
#89092=CARTESIAN_POINT('Ctrl Pts',(-5.41609137512249,8.33904474758301,15.0203640913354));
#89093=CARTESIAN_POINT('Ctrl Pts',(-5.56050597917073,8.24161011305476,15.0231538587763));
#89094=CARTESIAN_POINT('Ctrl Pts',(-5.76290397259949,8.10505484810113,15.02706373573));
#89095=CARTESIAN_POINT('Ctrl Pts',(-5.96030020701914,7.96101933280805,15.0309736126838));
#89096=CARTESIAN_POINT('Ctrl Pts',(-6.15214611927763,7.80989514187337,15.0348834896376));
#89097=CARTESIAN_POINT('Ctrl Pts',(-6.3439588212522,7.65879711191979,15.0387926897559));
#89098=CARTESIAN_POINT('Ctrl Pts',(-6.53022289897422,7.5006130292946,15.0427018898742));
#89099=CARTESIAN_POINT('Ctrl Pts',(-6.71042164104554,7.33577571899439,15.0466110899924));
#89100=CARTESIAN_POINT('Ctrl Pts',(-6.89060076584068,7.1709563536532,15.0505198645369));
#89101=CARTESIAN_POINT('Ctrl Pts',(-7.06471566664228,6.9994853959583,15.0544286390814));
#89102=CARTESIAN_POINT('Ctrl Pts',(-7.23228460824575,6.82183430943112,15.058337413626));
#89103=CARTESIAN_POINT('Ctrl Pts',(-7.39986655405268,6.64416943627468,15.0622464915113));
#89104=CARTESIAN_POINT('Ctrl Pts',(-7.56090133099839,6.4603236777518,15.0661555693966));
#89105=CARTESIAN_POINT('Ctrl Pts',(-7.71494492832411,6.27080447414254,15.0700646472819));
#89106=CARTESIAN_POINT('Ctrl Pts',(-7.86898639847684,6.08128788758545,15.0739736711872));
#89107=CARTESIAN_POINT('Ctrl Pts',(-8.01603670687459,5.88609823146361,15.0778826950924));
#89108=CARTESIAN_POINT('Ctrl Pts',(-8.15569246207227,5.68577562554992,15.0817917189977));
#89109=CARTESIAN_POINT('Ctrl Pts',(-8.29537893036041,5.48540896469336,15.0857016025753));
#89110=CARTESIAN_POINT('Ctrl Pts',(-8.42766743480796,5.27990732789923,15.089611486153));
#89111=CARTESIAN_POINT('Ctrl Pts',(-8.55219743893893,5.06984052662472,15.0935213697307));
#89112=CARTESIAN_POINT('Ctrl Pts',(-8.64105168332479,4.91995434435036,15.0963111371716));
#89113=CARTESIAN_POINT('Ctrl Pts',(-8.72595692350404,4.76774462980351,15.0991009046124));
#89114=CARTESIAN_POINT('Ctrl Pts',(-8.80679624371355,4.61342648383097,15.1018906720533));
#89115=CARTESIAN_POINT('Ctrl Pts',(-8.91997001929561,4.39738350901037,15.1057963025491));
#89116=CARTESIAN_POINT('Ctrl Pts',(-9.02520827542342,4.1771395377998,15.109701933045));
#89117=CARTESIAN_POINT('Ctrl Pts',(-9.12221448249565,3.95329823506229,15.1136075635409));
#89118=CARTESIAN_POINT('Ctrl Pts',(-9.21920355188142,3.72949647744441,15.1175125040451));
#89119=CARTESIAN_POINT('Ctrl Pts',(-9.30796336338345,3.50209891511801,15.1214174445494));
#89120=CARTESIAN_POINT('Ctrl Pts',(-9.38824499467587,3.27173041675862,15.1253223850536));
#89121=CARTESIAN_POINT('Ctrl Pts',(-9.46851786192404,3.04138706686318,15.1292268992702));
#89122=CARTESIAN_POINT('Ctrl Pts',(-9.54031430430537,2.80807369426392,15.1331314134867));
#89123=CARTESIAN_POINT('Ctrl Pts',(-9.60343452253734,2.57243257857965,15.1370359277033));
#89124=CARTESIAN_POINT('Ctrl Pts',(-9.66655941457757,2.33677401458134,15.140940731034));
#89125=CARTESIAN_POINT('Ctrl Pts',(-9.72100672317706,2.09878763433068,15.1448455343648));
#89126=CARTESIAN_POINT('Ctrl Pts',(-9.76662693389493,1.85912945598688,15.1487503376955));
#89127=CARTESIAN_POINT('Ctrl Pts',(-9.81224685516775,1.61947279819445,15.1526551162516));
#89128=CARTESIAN_POINT('Ctrl Pts',(-9.84903974021967,1.37814464055025,15.1565598948077));
#89129=CARTESIAN_POINT('Ctrl Pts',(-9.87690733898645,1.13581046705674,15.1604646733637));
#89130=CARTESIAN_POINT('Ctrl Pts',(-9.90478082891521,0.893425064539732,
15.1643702773832));
#89131=CARTESIAN_POINT('Ctrl Pts',(-9.92372523004582,0.650033500982153,
15.1682758814027));
#89132=CARTESIAN_POINT('Ctrl Pts',(-9.93369410819283,0.40630698351737,15.1721814854221));
#89133=CARTESIAN_POINT('Ctrl Pts',(-9.93923159351023,0.270922440540864,
15.1743509597195));
#89134=CARTESIAN_POINT('Ctrl Pts',(-9.94200056172094,0.1354346160241,15.1765204340168));
#89135=CARTESIAN_POINT('Ctrl Pts',(-9.94199999991451,-4.12286006677384E-5,
15.1786899083142));
#89136=CARTESIAN_POINT('Origin',(0.,0.,0.));
#89137=CARTESIAN_POINT('',(-9.94157881028341,-0.000218552330966126,16.3213100916858));
#89138=CARTESIAN_POINT('',(-9.94156315955438,-0.000215792232726663,16.1786899083142));
#89139=CARTESIAN_POINT('',(-9.942,-1.2175438477123E-15,0.));
#89140=CARTESIAN_POINT('Ctrl Pts',(-9.94157881028341,-0.000218552330966126,
16.3213100916858));
#89141=CARTESIAN_POINT('Ctrl Pts',(-9.94066271461031,1.11431393761154,16.3034700970927));
#89142=CARTESIAN_POINT('Ctrl Pts',(-9.47830442710447,3.86925058390486,16.2593844980741));
#89143=CARTESIAN_POINT('Ctrl Pts',(-6.98191316447499,7.64950719205534,16.1890532946296));
#89144=CARTESIAN_POINT('Ctrl Pts',(-2.51294062811132,10.0472484347585,16.1103164813527));
#89145=CARTESIAN_POINT('Ctrl Pts',(2.55862180591419,10.0357125391651,16.0315796680756));
#89146=CARTESIAN_POINT('Ctrl Pts',(7.01664023694587,7.61766575125248,15.9528428547988));
#89147=CARTESIAN_POINT('Ctrl Pts',(9.79210537743402,3.37294292723244,15.8741060415217));
#89148=CARTESIAN_POINT('Ctrl Pts',(10.2194753373836,-1.68059380627902,15.7953692282448));
#89149=CARTESIAN_POINT('Ctrl Pts',(8.19626905631817,-6.33113301624731,15.7166324149677));
#89150=CARTESIAN_POINT('Ctrl Pts',(4.20764072067247,-9.46349994868898,15.6378956016907));
#89151=CARTESIAN_POINT('Ctrl Pts',(-0.789957649186856,-10.3265695477982,
15.5591587884139));
#89152=CARTESIAN_POINT('Ctrl Pts',(-5.59812834466891,-8.71338227955533,
15.4804219751368));
#89153=CARTESIAN_POINT('Ctrl Pts',(-9.06389741358393,-5.01077193544794,
15.4016851618598));
#89154=CARTESIAN_POINT('Ctrl Pts',(-9.93438976965992,-1.70731401312795,
15.3486478673762));
#89155=CARTESIAN_POINT('Ctrl Pts',(-9.9428212718197,-0.0341387347268834,
15.3218561773182));
#89156=CARTESIAN_POINT('Ctrl Pts',(-9.9428143739607,-3.4919416618262E-5,
15.3213100916858));
#89157=CARTESIAN_POINT('Ctrl Pts',(-9.94281021402477,-4.12319605559286E-5,
15.1786899083142));
#89158=CARTESIAN_POINT('Ctrl Pts',(-9.94281975151917,-0.040376084069569,
15.1793357673195));
#89159=CARTESIAN_POINT('Ctrl Pts',(-9.94257935794541,-0.0807108220809731,
15.1799816263249));
#89160=CARTESIAN_POINT('Ctrl Pts',(-9.92213453281451,-1.7599907672817,15.2068730897559));
#89161=CARTESIAN_POINT('Ctrl Pts',(-9.0544577245587,-5.02780939552147,15.2593642986071));
#89162=CARTESIAN_POINT('Ctrl Pts',(-5.58173134501452,-8.72389518481278,
15.3381011118842));
#89163=CARTESIAN_POINT('Ctrl Pts',(-0.770535252865366,-10.3280369590551,
15.4168379251612));
#89164=CARTESIAN_POINT('Ctrl Pts',(4.22543112554584,-9.45556998846635,15.4955747384382));
#89165=CARTESIAN_POINT('Ctrl Pts',(8.20816142456435,-6.31570724715832,15.5743115517152));
#89166=CARTESIAN_POINT('Ctrl Pts',(10.2226179418717,-1.66137124630252,15.653048364992));
#89167=CARTESIAN_POINT('Ctrl Pts',(9.78574463819948,3.39135280964152,15.7317851782691));
#89168=CARTESIAN_POINT('Ctrl Pts',(7.00230142567361,7.63084836355288,15.8105219915461));
#89169=CARTESIAN_POINT('Ctrl Pts',(2.53974329387374,10.0405067603537,15.8892588048229));
#89170=CARTESIAN_POINT('Ctrl Pts',(-2.53183187341625,10.0425046362111,15.9679956181));
#89171=CARTESIAN_POINT('Ctrl Pts',(-6.99628712208093,7.63636291102297,16.046732431377));
#89172=CARTESIAN_POINT('Ctrl Pts',(-9.48203316727476,3.8567874690065,16.1169638614483));
#89173=CARTESIAN_POINT('Ctrl Pts',(-9.9406658297407,1.10808848775586,16.1609496870941));
#89174=CARTESIAN_POINT('Ctrl Pts',(-9.94156315955438,-0.000215792232726663,
16.1786899083142));
#89175=CARTESIAN_POINT('Origin',(0.,0.,0.));
#89176=CARTESIAN_POINT('',(-9.94136243353558,0.000162173653817377,17.3213100916858));
#89177=CARTESIAN_POINT('',(-9.94137407189289,0.000167045264107003,17.1786899083142));
#89178=CARTESIAN_POINT('',(-9.942,-1.2175438477123E-15,0.));
#89179=CARTESIAN_POINT('Ctrl Pts',(-9.94136243353558,0.000162173653817377,
17.3213100916858));
#89180=CARTESIAN_POINT('Ctrl Pts',(-9.94173254800261,0.623719662799634,
17.311329621293));
#89181=CARTESIAN_POINT('Ctrl Pts',(-9.73204865908736,2.88679819383414,17.2751035464743));
#89182=CARTESIAN_POINT('Ctrl Pts',(-8.03455596699662,6.53513275653972,17.2126318672303));
#89183=CARTESIAN_POINT('Ctrl Pts',(-3.96846040138357,9.56626411515653,17.1338950539532));
#89184=CARTESIAN_POINT('Ctrl Pts',(1.0492513505079,10.3034525871473,17.0551582406764));
#89185=CARTESIAN_POINT('Ctrl Pts',(5.81535799701473,8.56992919148952,16.9764214273993));
#89186=CARTESIAN_POINT('Ctrl Pts',(9.18697258070385,4.78138115006309,16.8976846141223));
#89187=CARTESIAN_POINT('Ctrl Pts',(10.3555995890163,-0.153716407029685,
16.8189478008455));
#89188=CARTESIAN_POINT('Ctrl Pts',(9.041008502631,-5.05195381048614,16.7402109875684));
#89189=CARTESIAN_POINT('Ctrl Pts',(5.55843128949705,-8.73875923938874,16.6614741742914));
#89190=CARTESIAN_POINT('Ctrl Pts',(0.742971600270773,-10.3300563923589,
16.5827373610144));
#89191=CARTESIAN_POINT('Ctrl Pts',(-4.25064876001462,-9.4442605196381,16.5040005477376));
#89192=CARTESIAN_POINT('Ctrl Pts',(-8.22498598363295,-6.29378084331697,
16.4252637344605));
#89193=CARTESIAN_POINT('Ctrl Pts',(-9.77340015076588,-2.68986805686518,
16.3643669157766));
#89194=CARTESIAN_POINT('Ctrl Pts',(-9.94201044397911,-0.525349050959409,
16.3297157015184));
#89195=CARTESIAN_POINT('Ctrl Pts',(-9.94157881028341,-0.000218552330966126,
16.3213100916858));
#89196=CARTESIAN_POINT('Ctrl Pts',(-9.94156315955438,-0.000215792232726663,
16.1786899083142));
#89197=CARTESIAN_POINT('Ctrl Pts',(-9.94199337594416,-0.531581917419294,
16.1871952915198));
#89198=CARTESIAN_POINT('Ctrl Pts',(-9.77087211432573,-2.70234409750878,
16.2219462791508));
#89199=CARTESIAN_POINT('Ctrl Pts',(-8.2131348446615,-6.30923830794241,16.282942871208));
#89200=CARTESIAN_POINT('Ctrl Pts',(-4.23287959110267,-9.45223795575133,
16.3616796844848));
#89201=CARTESIAN_POINT('Ctrl Pts',(0.762397844591911,-10.3286408363935,
16.4404164977619));
#89202=CARTESIAN_POINT('Ctrl Pts',(5.57485630153356,-8.72829016619386,16.5191533110387));
#89203=CARTESIAN_POINT('Ctrl Pts',(9.05049364508474,-5.03494158647097,16.5978901243158));
#89204=CARTESIAN_POINT('Ctrl Pts',(10.3558703866554,-0.134240594147907,
16.6766269375928));
#89205=CARTESIAN_POINT('Ctrl Pts',(9.1779640746773,4.79865058833391,16.7553637508696));
#89206=CARTESIAN_POINT('Ctrl Pts',(5.79923042414636,8.580850681741,16.8341005641467));
#89207=CARTESIAN_POINT('Ctrl Pts',(1.02987193105673,10.3054080930073,16.9128373774237));
#89208=CARTESIAN_POINT('Ctrl Pts',(-3.98644441696093,9.5587830107304,16.9915741907007));
#89209=CARTESIAN_POINT('Ctrl Pts',(-8.04683243255047,6.52001228063464,17.0703110039775));
#89210=CARTESIAN_POINT('Ctrl Pts',(-9.73476031103565,2.87432000866741,17.1326829098488));
#89211=CARTESIAN_POINT('Ctrl Pts',(-9.94175055725434,0.617488319087645,
17.1688092112943));
#89212=CARTESIAN_POINT('Ctrl Pts',(-9.94137407189289,0.000167045264107003,
17.1786899083142));
#89213=CARTESIAN_POINT('Origin',(0.,0.,0.));
#89214=CARTESIAN_POINT('',(-4.30729783501544,8.96073829072084,18.));
#89215=CARTESIAN_POINT('Ctrl Pts',(-9.94137407189289,0.000167045264107003,
17.1786899083142));
#89216=CARTESIAN_POINT('Ctrl Pts',(-9.94075051789995,-1.02227149985294,
17.19505481572));
#89217=CARTESIAN_POINT('Ctrl Pts',(-9.53207699775168,-3.68495707954238,
17.2376653275512));
#89218=CARTESIAN_POINT('Ctrl Pts',(-7.19187963366665,-7.45244541015752,
17.3065214438087));
#89219=CARTESIAN_POINT('Ctrl Pts',(-2.79129440548034,-9.9735018662042,17.3852582570854));
#89220=CARTESIAN_POINT('Ctrl Pts',(2.27862837048033,-10.1029668943729,17.4639950703625));
#89221=CARTESIAN_POINT('Ctrl Pts',(6.8021483171817,-7.80979054448228,17.5427318836394));
#89222=CARTESIAN_POINT('Ctrl Pts',(9.69454856507843,-3.64387394710659,17.6214686969163));
#89223=CARTESIAN_POINT('Ctrl Pts',(10.2622480917845,1.39583661306226,17.7002055101934));
#89224=CARTESIAN_POINT('Ctrl Pts',(8.36911304595686,6.10080919945852,17.7789423234704));
#89225=CARTESIAN_POINT('Ctrl Pts',(4.46911207265963,9.34288597599586,17.8576791367474));
#89226=CARTESIAN_POINT('Ctrl Pts',(-0.183634414914874,10.2802458074126,
17.9313650289238));
#89227=CARTESIAN_POINT('Ctrl Pts',(-3.11352491188595,9.53306574361534,17.9788053166748));
#89228=CARTESIAN_POINT('Ctrl Pts',(-4.30729783501544,8.96073829072084,18.));
#89229=CARTESIAN_POINT('',(4.30700275658802,8.96064123010977,18.));
#89230=CARTESIAN_POINT('Origin',(0.,0.,18.));
#89231=CARTESIAN_POINT('Ctrl Pts',(4.30700275658802,8.96064123010977,18.));
#89232=CARTESIAN_POINT('Ctrl Pts',(5.78466622438187,8.25039065030617,17.9737543955743));
#89233=CARTESIAN_POINT('Ctrl Pts',(8.38051870287619,6.0857105851668,17.9212631867231));
#89234=CARTESIAN_POINT('Ctrl Pts',(10.2648846152864,1.37622265143462,17.842526373446));
#89235=CARTESIAN_POINT('Ctrl Pts',(9.68766298633001,-3.66194177412479,17.7637895601691));
#89236=CARTESIAN_POINT('Ctrl Pts',(6.78745652630585,-7.82265065129397,17.6850527468922));
#89237=CARTESIAN_POINT('Ctrl Pts',(2.25961974458035,-10.1071925353341,17.6063159336151));
#89238=CARTESIAN_POINT('Ctrl Pts',(-2.81004433424633,-9.96825624824068,
17.5275791203381));
#89239=CARTESIAN_POINT('Ctrl Pts',(-7.20588368450361,-7.43889545753228,
17.4488423070613));
#89240=CARTESIAN_POINT('Ctrl Pts',(-9.53560930616682,-3.67249284691441,
17.3800859641771));
#89241=CARTESIAN_POINT('Ctrl Pts',(-9.94075925941884,-1.01604705686179,
17.3375752257186));
#89242=CARTESIAN_POINT('Ctrl Pts',(-9.94136243353558,0.000162173653817377,
17.3213100916858));
#89243=CARTESIAN_POINT('Origin',(0.,0.,2.15141010809499));
#89244=CARTESIAN_POINT('',(5.43505795426094,-7.63293718671423,18.));
#89245=CARTESIAN_POINT('Ctrl Pts',(5.43505795426094,-7.63293718671423,18.));
#89246=CARTESIAN_POINT('Ctrl Pts',(5.17173340930988,-7.82043829245888,17.9943178253384));
#89247=CARTESIAN_POINT('Ctrl Pts',(4.8988798102261,-7.99418927223705,17.9886342308681));
#89248=CARTESIAN_POINT('Ctrl Pts',(4.54641891280022,-8.19379950750167,17.9816362724925));
#89249=CARTESIAN_POINT('Ctrl Pts',(4.47472144112314,-8.23317334688816,17.9802292444045));
#89250=CARTESIAN_POINT('Ctrl Pts',(4.33644627871265,-8.30676957699183,17.9775472605171));
#89251=CARTESIAN_POINT('Ctrl Pts',(4.26995593257482,-8.34114281713787,17.9762713286267));
#89252=CARTESIAN_POINT('Ctrl Pts',(4.1276715741662,-8.41255178530606,17.9735694011271));
#89253=CARTESIAN_POINT('Ctrl Pts',(4.0517747605446,-8.44936811214072,17.9721450558189));
#89254=CARTESIAN_POINT('Ctrl Pts',(3.84668008784851,-8.54545728989826,17.968338909957));
#89255=CARTESIAN_POINT('Ctrl Pts',(3.71661343720383,-8.60282353122374,17.9659703690349));
#89256=CARTESIAN_POINT('Ctrl Pts',(3.27981056713658,-8.78372084504184,17.9581405576608));
#89257=CARTESIAN_POINT('Ctrl Pts',(2.96784776287721,-8.89397484187954,17.9527567734968));
#89258=CARTESIAN_POINT('Ctrl Pts',(2.55580612313983,-9.01549947057141,17.9456816874559));
#89259=CARTESIAN_POINT('Ctrl Pts',(2.46046313216061,-9.041985222169,17.9440462316115));
#89260=CARTESIAN_POINT('Ctrl Pts',(2.33702254301936,-9.07417929918066,17.9419223979961));
#89261=CARTESIAN_POINT('Ctrl Pts',(2.3092933810926,-9.08127570324028,17.9414448897797));
#89262=CARTESIAN_POINT('Ctrl Pts',(2.27360711410161,-9.09023445889745,17.9408295961921));
#89263=CARTESIAN_POINT('Ctrl Pts',(2.26567947211113,-9.09221361147132,17.9406928615992));
#89264=CARTESIAN_POINT('Ctrl Pts',(2.24168151600013,-9.09817141670899,17.9402787908133));
#89265=CARTESIAN_POINT('Ctrl Pts',(2.22560324193713,-9.10211785003997,17.9400011550254));
#89266=CARTESIAN_POINT('Ctrl Pts',(2.19659036470876,-9.10915762858463,17.9394997187239));
#89267=CARTESIAN_POINT('Ctrl Pts',(2.18365947172891,-9.11226608720395,17.9392760705546));
#89268=CARTESIAN_POINT('Ctrl Pts',(2.14432794399045,-9.12163246819743,17.9385952632139));
#89269=CARTESIAN_POINT('Ctrl Pts',(2.11790672340901,-9.1278032584424,17.9381371833745));
#89270=CARTESIAN_POINT('Ctrl Pts',(2.05069967107279,-9.14319224111505,17.9369696900891));
#89271=CARTESIAN_POINT('Ctrl Pts',(2.00987843827555,-9.15225229909239,17.9362582711727));
#89272=CARTESIAN_POINT('Ctrl Pts',(1.90661786928515,-9.17444627171035,17.9344532117096));
#89273=CARTESIAN_POINT('Ctrl Pts',(1.84410260853059,-9.18721620698452,17.9333556057256));
#89274=CARTESIAN_POINT('Ctrl Pts',(1.60055448070495,-9.23437952569823,17.9290670197665));
#89275=CARTESIAN_POINT('Ctrl Pts',(1.41865333028027,-9.26406834607901,17.9258379397813));
#89276=CARTESIAN_POINT('Ctrl Pts',(1.06960173865389,-9.31051633678268,17.9196515202567));
#89277=CARTESIAN_POINT('Ctrl Pts',(0.902642524715984,-9.3281830427163,17.9166966088536));
#89278=CARTESIAN_POINT('Ctrl Pts',(0.590802233253205,-9.35272936024783,
17.9112144478403));
#89279=CARTESIAN_POINT('Ctrl Pts',(0.446060717354184,-9.3607491020278,17.9086845123872));
#89280=CARTESIAN_POINT('Ctrl Pts',(0.189989278514941,-9.36898435356703,
17.9042438448726));
#89281=CARTESIAN_POINT('Ctrl Pts',(0.078732203131157,-9.37057976180315,
17.9023261134129));
#89282=CARTESIAN_POINT('Ctrl Pts',(-0.095456492859394,-9.36997509513793,
17.8993427759256));
#89283=CARTESIAN_POINT('Ctrl Pts',(-0.158382204390103,-9.36912270812688,
17.8982689273276));
#89284=CARTESIAN_POINT('Ctrl Pts',(-0.264010037201853,-9.36662742871493,
17.8964726770231));
#89285=CARTESIAN_POINT('Ctrl Pts',(-0.30671808787091,-9.36532619335901,
17.8957481403264));
#89286=CARTESIAN_POINT('Ctrl Pts',(-0.44330767803551,-9.36022923493316,
17.8934362089332));
#89287=CARTESIAN_POINT('Ctrl Pts',(-0.537141697500538,-9.35531356388984,
17.8918560202705));
#89288=CARTESIAN_POINT('Ctrl Pts',(-1.04408865822473,-9.32110389608918,
17.8833548000159));
#89289=CARTESIAN_POINT('Ctrl Pts',(-1.45498681725177,-9.26585732928013,
17.876616120775));
#89290=CARTESIAN_POINT('Ctrl Pts',(-1.97151996293981,-9.16119194995781,
17.8679552600374));
#89291=CARTESIAN_POINT('Ctrl Pts',(-2.08174572454483,-9.13677533736938,
17.8660942221446));
#89292=CARTESIAN_POINT('Ctrl Pts',(-2.24918875884167,-9.09649686264499,
17.8632327463826));
#89293=CARTESIAN_POINT('Ctrl Pts',(-2.30674121291386,-9.08207301241379,
17.8622429414518));
#89294=CARTESIAN_POINT('Ctrl Pts',(-2.36633916169708,-9.06653346874789,
17.8612098175093));
#89295=CARTESIAN_POINT('Ctrl Pts',(-2.36852541298319,-9.06596258188607,
17.8611719076688));
#89296=CARTESIAN_POINT('Ctrl Pts',(-2.37276464952788,-9.0648539692787,17.8610983765297));
#89297=CARTESIAN_POINT('Ctrl Pts',(-2.37481765904612,-9.06431633675032,
17.861062756166));
#89298=CARTESIAN_POINT('Ctrl Pts',(-2.37880579743203,-9.06327049379004,
17.860993540846));
#89299=CARTESIAN_POINT('Ctrl Pts',(-2.38074094654839,-9.06276236094318,
17.8609599466752));
#89300=CARTESIAN_POINT('Ctrl Pts',(-2.38450706501532,-9.06177216135061,
17.8608945490873));
#89301=CARTESIAN_POINT('Ctrl Pts',(-2.3863380513045,-9.06129015936651,17.8608627463318));
#89302=CARTESIAN_POINT('Ctrl Pts',(-2.38990809638021,-9.06034919792419,
17.8608007214468));
#89303=CARTESIAN_POINT('Ctrl Pts',(-2.39164716937723,-9.05989029264033,
17.8607704998755));
#89304=CARTESIAN_POINT('Ctrl Pts',(-2.39504439832398,-9.05899278807569,
17.8607114482788));
#89305=CARTESIAN_POINT('Ctrl Pts',(-2.39670256619049,-9.05855423417919,
17.8606826187249));
#89306=CARTESIAN_POINT('Ctrl Pts',(-2.39994793551505,-9.0576949421774,17.8606261800599));
#89307=CARTESIAN_POINT('Ctrl Pts',(-2.40153514698501,-9.05727424209537,
17.8605985713466));
#89308=CARTESIAN_POINT('Ctrl Pts',(-2.40464765545685,-9.05644837705684,
17.8605444185095));
#89309=CARTESIAN_POINT('Ctrl Pts',(-2.4061729608505,-9.05604324391514,17.8605178747209));
#89310=CARTESIAN_POINT('Ctrl Pts',(-2.40916995419383,-9.05524640822137,
17.8604657086887));
#89311=CARTESIAN_POINT('Ctrl Pts',(-2.41064164915234,-9.05485473219576,
17.8604400867266));
#89312=CARTESIAN_POINT('Ctrl Pts',(-2.41353909346036,-9.05408285162861,
17.8603896319029));
#89313=CARTESIAN_POINT('Ctrl Pts',(-2.41496484861779,-9.0537026690607,17.8603647992761));
#89314=CARTESIAN_POINT('Ctrl Pts',(-2.41777757870084,-9.05295193312329,
17.8603157992498));
#89315=CARTESIAN_POINT('Ctrl Pts',(-2.4191645583989,-9.05258139775035,17.8602916320438));
#89316=CARTESIAN_POINT('Ctrl Pts',(-2.42190650722443,-9.05184820355637,
17.8602438456585));
#89317=CARTESIAN_POINT('Ctrl Pts',(-2.42326148018509,-9.05148555921146,
17.8602202266361));
#89318=CARTESIAN_POINT('Ctrl Pts',(-2.42594589511924,-9.05076645765053,
17.8601734242729));
#89319=CARTESIAN_POINT('Ctrl Pts',(-2.42727534008299,-9.05041001172889,
17.8601502410554));
#89320=CARTESIAN_POINT('Ctrl Pts',(-2.42991499213949,-9.04970165441712,
17.860104201023));
#89321=CARTESIAN_POINT('Ctrl Pts',(-2.43122520144201,-9.04934975138309,
17.8600813442998));
#89322=CARTESIAN_POINT('Ctrl Pts',(-2.43383259373152,-9.0486488368531,17.860035849225));
#89323=CARTESIAN_POINT('Ctrl Pts',(-2.43512977817829,-9.04829983093077,
17.8600132109349));
#89324=CARTESIAN_POINT('Ctrl Pts',(-2.43771736071058,-9.04760304820377,
17.8599680440296));
#89325=CARTESIAN_POINT('Ctrl Pts',(-2.4390077595318,-9.04725527425414,17.8599455154464));
#89326=CARTESIAN_POINT('Ctrl Pts',(-2.44158815874383,-9.04655924155516,
17.8599004565054));
#89327=CARTESIAN_POINT('Ctrl Pts',(-2.44287815913675,-9.04621098291973,
17.8598779261494));
#89328=CARTESIAN_POINT('Ctrl Pts',(-2.44546443228321,-9.04551217876263,
17.8598327470999));
#89329=CARTESIAN_POINT('Ctrl Pts',(-2.44676070426629,-9.04516163049414,
17.8598100983761));
#89330=CARTESIAN_POINT('Ctrl Pts',(-2.44936663183124,-9.04445631347901,
17.8597645581481));
#89331=CARTESIAN_POINT('Ctrl Pts',(-2.45067628580571,-9.04410153888975,
17.8597416665786));
#89332=CARTESIAN_POINT('Ctrl Pts',(-2.45331671935038,-9.04338565131626,
17.8596955049889));
#89333=CARTESIAN_POINT('Ctrl Pts',(-2.45464749636279,-9.04302452902106,
17.859672234864));
#89334=CARTESIAN_POINT('Ctrl Pts',(-2.45733878565391,-9.0422935775603,17.8596251650918));
#89335=CARTESIAN_POINT('Ctrl Pts',(-2.45869929426579,-9.04192373506014,
17.8596013652938));
#89336=CARTESIAN_POINT('Ctrl Pts',(-2.46145982746429,-9.04117263886177,
17.8595530643505));
#89337=CARTESIAN_POINT('Ctrl Pts',(-2.46285984706647,-9.04079136700049,
17.8595285629984));
#89338=CARTESIAN_POINT('Ctrl Pts',(-2.46571075296803,-9.04001425922299,
17.8594786593226));
#89339=CARTESIAN_POINT('Ctrl Pts',(-2.4671616326451,-9.03961839917265,17.8594532567222));
#89340=CARTESIAN_POINT('Ctrl Pts',(-2.47012771793563,-9.03880836100521,
17.859401313607));
#89341=CARTESIAN_POINT('Ctrl Pts',(-2.47164291482507,-9.03839415114688,
17.8593747727259));
#89342=CARTESIAN_POINT('Ctrl Pts',(-2.47475394849737,-9.03754284607514,
17.8593202655879));
#89343=CARTESIAN_POINT('Ctrl Pts',(-2.47634977378964,-9.03710570913601,
17.8592922988465));
#89344=CARTESIAN_POINT('Ctrl Pts',(-2.47964229611515,-9.0362028663305,17.859234583188));
#89345=CARTESIAN_POINT('Ctrl Pts',(-2.48133897791757,-9.03573710522994,
17.8592048336251));
#89346=CARTESIAN_POINT('Ctrl Pts',(-2.4848589247123,-9.0347697681043,17.8591430985237));
#89347=CARTESIAN_POINT('Ctrl Pts',(-2.4866821692442,-9.03426811797922,17.8591111121125));
#89348=CARTESIAN_POINT('Ctrl Pts',(-2.48940337214991,-9.0335185161175,17.8590633584406));
#89349=CARTESIAN_POINT('Ctrl Pts',(-2.49030144569378,-9.03327098231225,
17.8590475961459));
#89350=CARTESIAN_POINT('Ctrl Pts',(-2.49269679964682,-9.03261037242341,
17.8590055487498));
#89351=CARTESIAN_POINT('Ctrl Pts',(-2.4941940142548,-9.03219705798294,17.8589792608062));
#89352=CARTESIAN_POINT('Ctrl Pts',(-2.49840305712354,-9.03103400186164,
17.8589053412177));
#89353=CARTESIAN_POINT('Ctrl Pts',(-2.50111465039944,-9.03028341106633,
17.8588576993873));
#89354=CARTESIAN_POINT('Ctrl Pts',(-2.50571645285452,-9.02900736345855,
17.8587768119355));
#89355=CARTESIAN_POINT('Ctrl Pts',(-2.50760683593739,-9.0284825340615,17.8587435739284));
#89356=CARTESIAN_POINT('Ctrl Pts',(-2.51922633715825,-9.02525266669247,
17.8585392094608));
#89357=CARTESIAN_POINT('Ctrl Pts',(-2.52895123905259,-9.02253249735524,
17.858367898119));
#89358=CARTESIAN_POINT('Ctrl Pts',(-2.57692837139369,-9.00902906769203,
17.8575213750912));
#89359=CARTESIAN_POINT('Ctrl Pts',(-2.61511606462939,-8.99801825578328,
17.8568432510961));
#89360=CARTESIAN_POINT('Ctrl Pts',(-2.7269507693098,-8.96500042612023,17.8548457722729));
#89361=CARTESIAN_POINT('Ctrl Pts',(-2.80039834061533,-8.94232979869343,
17.8535191871347));
#89362=CARTESIAN_POINT('Ctrl Pts',(-3.21514719986506,-8.80870075620339,
17.8459594578482));
#89363=CARTESIAN_POINT('Ctrl Pts',(-3.55013107320787,-8.6791100095911,17.8396009484144));
#89364=CARTESIAN_POINT('Ctrl Pts',(-3.99617198722411,-8.47640085071411,
17.8310292850766));
#89365=CARTESIAN_POINT('Ctrl Pts',(-4.11433821616512,-8.41967832491412,
17.8287464056948));
#89366=CARTESIAN_POINT('Ctrl Pts',(-4.32944669356626,-8.31081117938263,
17.8245744894209));
#89367=CARTESIAN_POINT('Ctrl Pts',(-4.42673494212108,-8.25940124774662,
17.8226813163502));
#89368=CARTESIAN_POINT('Ctrl Pts',(-4.59289171300171,-8.16781991949712,
17.8194376033794));
#89369=CARTESIAN_POINT('Ctrl Pts',(-4.66219448547851,-8.12846105600316,
17.8180814487509));
#89370=CARTESIAN_POINT('Ctrl Pts',(-4.80825529160954,-8.04302674492959,
17.815215577553));
#89371=CARTESIAN_POINT('Ctrl Pts',(-4.88487225454889,-7.99672565947357,
17.8137076877283));
#89372=CARTESIAN_POINT('Ctrl Pts',(-5.11556459424748,-7.85276116603642,
17.8091499442718));
#89373=CARTESIAN_POINT('Ctrl Pts',(-5.26746235997193,-7.75169011417247,
17.8061254821021));
#89374=CARTESIAN_POINT('Ctrl Pts',(-5.47110055238523,-7.60744054226601,
17.8020133765405));
#89375=CARTESIAN_POINT('Ctrl Pts',(-5.52546911852387,-7.56804359707743,
17.8009095887904));
#89376=CARTESIAN_POINT('Ctrl Pts',(-5.73553736469515,-7.41235197194009,
17.7966166110124));
#89377=CARTESIAN_POINT('Ctrl Pts',(-5.88802745512071,-7.29180932295328,
17.7934401692021));
#89378=CARTESIAN_POINT('Ctrl Pts',(-6.15059826452214,-7.07063783835505,
17.7877910600257));
#89379=CARTESIAN_POINT('Ctrl Pts',(-6.26223254759748,-6.97195967658334,
17.7853276886563));
#89380=CARTESIAN_POINT('Ctrl Pts',(-6.41088827117743,-6.83410471048899,
17.7819303760864));
#89381=CARTESIAN_POINT('Ctrl Pts',(-6.44999480582586,-6.79720844219528,
17.7810251689012));
#89382=CARTESIAN_POINT('Ctrl Pts',(-6.51948245708224,-6.73050849004815,
17.7793938098659));
#89383=CARTESIAN_POINT('Ctrl Pts',(-6.54998208221477,-6.70083060120725,
17.7786695235695));
#89384=CARTESIAN_POINT('Ctrl Pts',(-6.61901516356093,-6.63273577637062,
17.7770117166984));
#89385=CARTESIAN_POINT('Ctrl Pts',(-6.65741825669758,-6.59418893821198,
17.7760762915812));
#89386=CARTESIAN_POINT('Ctrl Pts',(-6.90114577647515,-6.34524974414563,
17.7700606523033));
#89387=CARTESIAN_POINT('Ctrl Pts',(-7.09680853719885,-6.12562776781217,
17.7648739067136));
#89388=CARTESIAN_POINT('Ctrl Pts',(-7.39447503280842,-5.75806949730283,
17.7565634306888));
#89389=CARTESIAN_POINT('Ctrl Pts',(-7.50311871094122,-5.61576666118042,
17.7534266386592));
#89390=CARTESIAN_POINT('Ctrl Pts',(-7.68587913412623,-5.36160575399376,
17.7479844753182));
#89391=CARTESIAN_POINT('Ctrl Pts',(-7.76179416352488,-5.25110520178583,
17.7456685424781));
#89392=CARTESIAN_POINT('Ctrl Pts',(-7.88080730734507,-5.06964914838692,
17.7419479200684));
#89393=CARTESIAN_POINT('Ctrl Pts',(-7.92537907135638,-4.99968328172741,
17.7405324801543));
#89394=CARTESIAN_POINT('Ctrl Pts',(-8.01271269076847,-4.85848953299843,
17.7377135355649));
#89395=CARTESIAN_POINT('Ctrl Pts',(-8.05546810646493,-4.7872663213259,17.7363101750378));
#89396=CARTESIAN_POINT('Ctrl Pts',(-8.16511258240989,-4.59898850408819,
17.7326468294348));
#89397=CARTESIAN_POINT('Ctrl Pts',(-8.23043242904693,-4.48104239159288,
17.7303983629533));
#89398=CARTESIAN_POINT('Ctrl Pts',(-8.44519726647871,-4.07269859987177,
17.7227502607937));
#89399=CARTESIAN_POINT('Ctrl Pts',(-8.58199585935785,-3.77592076526816,
17.7174303767798));
#89400=CARTESIAN_POINT('Ctrl Pts',(-8.76170886081674,-3.32552559871771,
17.7094574446755));
#89401=CARTESIAN_POINT('Ctrl Pts',(-8.81665846743111,-3.1769790456373,17.706841786847));
#89402=CARTESIAN_POINT('Ctrl Pts',(-8.88542812814894,-2.9755207694532,17.7032759598392));
#89403=CARTESIAN_POINT('Ctrl Pts',(-8.90258869274198,-2.92377691001589,
17.7023584285052));
#89404=CARTESIAN_POINT('Ctrl Pts',(-8.93228939684027,-2.83153461312139,
17.7007175813594));
#89405=CARTESIAN_POINT('Ctrl Pts',(-8.94500803018642,-2.7910953864332,17.6999963039132));
#89406=CARTESIAN_POINT('Ctrl Pts',(-8.97312511096158,-2.69952989921963,
17.6983591543055));
#89407=CARTESIAN_POINT('Ctrl Pts',(-8.98836184050942,-2.64835559195336,
17.6974415425835));
#89408=CARTESIAN_POINT('Ctrl Pts',(-9.08923736807116,-2.29865220910489,
17.6911593580062));
#89409=CARTESIAN_POINT('Ctrl Pts',(-9.16042570936088,-1.99615590881768,
17.6856746100559));
#89410=CARTESIAN_POINT('Ctrl Pts',(-9.24738045489873,-1.5221379244134,17.6772099419781));
#89411=CARTESIAN_POINT('Ctrl Pts',(-9.27366979599149,-1.35277413855341,
17.6742093367514));
#89412=CARTESIAN_POINT('Ctrl Pts',(-9.30307904527794,-1.12165193445107,
17.6701613101347));
#89413=CARTESIAN_POINT('Ctrl Pts',(-9.31025464449662,-1.06044389441446,
17.669093620974));
#89414=CARTESIAN_POINT('Ctrl Pts',(-9.327702919294,-0.897746231131952,17.6662677079331));
#89415=CARTESIAN_POINT('Ctrl Pts',(-9.33692305467132,-0.796151987863134,
17.6645156600135));
#89416=CARTESIAN_POINT('Ctrl Pts',(-9.35033546607144,-0.615669393400805,
17.661425569898));
#89417=CARTESIAN_POINT('Ctrl Pts',(-9.35519237750183,-0.536840519826683,
17.6600834659791));
#89418=CARTESIAN_POINT('Ctrl Pts',(-9.36364869020217,-0.364023800022639,
17.6571567877683));
#89419=CARTESIAN_POINT('Ctrl Pts',(-9.3668306914568,-0.270024021379157,
17.6555750100059));
#89420=CARTESIAN_POINT('Ctrl Pts',(-9.37244921469699,0.0290670400761349,
17.6505696804282));
#89421=CARTESIAN_POINT('Ctrl Pts',(-9.36956780917658,0.234197798430648,
17.6471792276701));
#89422=CARTESIAN_POINT('Ctrl Pts',(-9.34814447079211,0.690895122437159,
17.6396630215888));
#89423=CARTESIAN_POINT('Ctrl Pts',(-9.32617337359789,0.942141712008976,
17.6355508486332));
#89424=CARTESIAN_POINT('Ctrl Pts',(-9.28274444142092,1.28070425840881,17.6299221748402));
#89425=CARTESIAN_POINT('Ctrl Pts',(-9.27012730391731,1.369046194616,17.6284450033721));
#89426=CARTESIAN_POINT('Ctrl Pts',(-9.2455797347387,1.52497492148424,17.6258139309914));
#89427=CARTESIAN_POINT('Ctrl Pts',(-9.23416498448879,1.59263622613457,17.6246642674182));
#89428=CARTESIAN_POINT('Ctrl Pts',(-9.21441227425665,1.70235999137002,17.6227829179499));
#89429=CARTESIAN_POINT('Ctrl Pts',(-9.2065269247092,1.74450138629159,17.622056197817));
#89430=CARTESIAN_POINT('Ctrl Pts',(-9.18842549147059,1.83769771091373,17.6204388904723));
#89431=CARTESIAN_POINT('Ctrl Pts',(-9.17807255192514,1.88872446491027,17.6195468587525));
#89432=CARTESIAN_POINT('Ctrl Pts',(-9.14364260010235,2.05144842909699,17.6166841016798));
#89433=CARTESIAN_POINT('Ctrl Pts',(-9.11794764537212,2.16279247266174,17.6146980598199));
#89434=CARTESIAN_POINT('Ctrl Pts',(-9.03172707097941,2.50751054212063,17.60848999762));
#89435=CARTESIAN_POINT('Ctrl Pts',(-8.96422744525356,2.73903803209347,17.6042371945682));
#89436=CARTESIAN_POINT('Ctrl Pts',(-8.8155583916291,3.18428183696196,17.5960009448771));
#89437=CARTESIAN_POINT('Ctrl Pts',(-8.73534978439387,3.39814440108498,17.5920177556867));
#89438=CARTESIAN_POINT('Ctrl Pts',(-8.61129849737214,3.69539094008042,17.5864689864665));
#89439=CARTESIAN_POINT('Ctrl Pts',(-8.5738909715581,3.78137140125063,17.5848621231655));
#89440=CARTESIAN_POINT('Ctrl Pts',(-8.50258983866926,3.93875558063206,17.581917248113));
#89441=CARTESIAN_POINT('Ctrl Pts',(-8.4690710749203,4.01031976907668,17.5805767848049));
#89442=CARTESIAN_POINT('Ctrl Pts',(-8.39078039496613,4.17211381894889,17.5775419233537));
#89443=CARTESIAN_POINT('Ctrl Pts',(-8.34545074462236,4.26206303199321,17.5758516325593));
#89444=CARTESIAN_POINT('Ctrl Pts',(-8.15480909024632,4.6256525542636,17.5689986414954));
#89445=CARTESIAN_POINT('Ctrl Pts',(-7.99741806875747,4.89273723055219,17.5639232311556));
#89446=CARTESIAN_POINT('Ctrl Pts',(-7.69792564336745,5.34777710476087,17.5549937080992));
#89447=CARTESIAN_POINT('Ctrl Pts',(-7.56143022874022,5.53909300302034,17.5511420183421));
#89448=CARTESIAN_POINT('Ctrl Pts',(-7.38197849851632,5.77160577303791,17.5462304507517));
#89449=CARTESIAN_POINT('Ctrl Pts',(-7.34562996101493,5.81779685152484,17.5452427180747));
#89450=CARTESIAN_POINT('Ctrl Pts',(-7.28506001311455,5.89329541735242,17.543605792899));
#89451=CARTESIAN_POINT('Ctrl Pts',(-7.26109060063673,5.92280284624779,17.5429601787401));
#89452=CARTESIAN_POINT('Ctrl Pts',(-7.20217142363888,5.9944397671214,17.5413781864001));
#89453=CARTESIAN_POINT('Ctrl Pts',(-7.16703090961068,6.03641029581767,17.5404390969865));
#89454=CARTESIAN_POINT('Ctrl Pts',(-7.02390939662403,6.20433770297883,17.53663612949));
#89455=CARTESIAN_POINT('Ctrl Pts',(-6.91295983407911,6.32772436311716,17.5337376670905));
#89456=CARTESIAN_POINT('Ctrl Pts',(-6.61571769808706,6.64113264382029,17.5261598168459));
#89457=CARTESIAN_POINT('Ctrl Pts',(-6.42450354344367,6.82628142864941,17.5214674537071));
#89458=CARTESIAN_POINT('Ctrl Pts',(-6.13725192150899,7.08164673447656,17.5147571853769));
#89459=CARTESIAN_POINT('Ctrl Pts',(-6.04735193846027,7.15856942725955,17.5127010557886));
#89460=CARTESIAN_POINT('Ctrl Pts',(-5.87669772026817,7.29907982997101,17.5088826400314));
#89461=CARTESIAN_POINT('Ctrl Pts',(-5.79630704782713,7.36308136169744,17.5071174985878));
#89462=CARTESIAN_POINT('Ctrl Pts',(-5.65225519607771,7.47394413925783,17.5040134495763));
#89463=CARTESIAN_POINT('Ctrl Pts',(-5.58902317741581,7.52134627273996,17.5026703381065));
#89464=CARTESIAN_POINT('Ctrl Pts',(-5.44965948607934,7.62309282923207,17.4997512290324));
#89465=CARTESIAN_POINT('Ctrl Pts',(-5.37329833790121,7.6771086889815,17.4981779204531));
#89466=CARTESIAN_POINT('Ctrl Pts',(-4.96105298026001,7.95955596448136,17.489814956217));
#89467=CARTESIAN_POINT('Ctrl Pts',(-4.61139195497046,8.16710731926021,17.4831994402264));
#89468=CARTESIAN_POINT('Ctrl Pts',(-4.09779590051228,8.42843855321351,17.4737323081364));
#89469=CARTESIAN_POINT('Ctrl Pts',(-3.94415149332015,8.50142201912503,17.4709267787813));
#89470=CARTESIAN_POINT('Ctrl Pts',(-3.73798435551296,8.59256198411049,17.4671522037786));
#89471=CARTESIAN_POINT('Ctrl Pts',(-3.68716471958991,8.61449155809334,17.4662209372371));
#89472=CARTESIAN_POINT('Ctrl Pts',(-3.59716792531311,8.65238448829839,17.4645679384425));
#89473=CARTESIAN_POINT('Ctrl Pts',(-3.55807147983913,8.66853515562089,17.4638484218738));
#89474=CARTESIAN_POINT('Ctrl Pts',(-3.46049619639913,8.70807198395108,17.4620494472781));
#89475=CARTESIAN_POINT('Ctrl Pts',(-3.40188852154157,8.731134294211,17.4609662711997));
#89476=CARTESIAN_POINT('Ctrl Pts',(-3.05004679173551,8.86550472347874,17.4544569331904));
#89477=CARTESIAN_POINT('Ctrl Pts',(-2.7516073127372,8.9626232997902,17.4489151936215));
#89478=CARTESIAN_POINT('Ctrl Pts',(-2.289278927606,9.08780064158446,17.4405056123968));
#89479=CARTESIAN_POINT('Ctrl Pts',(-2.12858066178144,9.12677725577002,17.437612546485));
#89480=CARTESIAN_POINT('Ctrl Pts',(-1.84205614088508,9.18829297884701,17.4325233808913));
#89481=CARTESIAN_POINT('Ctrl Pts',(-1.71664166978723,9.21254797552443,17.4303188085686));
#89482=CARTESIAN_POINT('Ctrl Pts',(-1.50993939243815,9.24815633737036,17.4267248355999));
#89483=CARTESIAN_POINT('Ctrl Pts',(-1.42892894402909,9.26101909726844,17.4253261191149));
#89484=CARTESIAN_POINT('Ctrl Pts',(-1.27442953798112,9.28347485399893,17.4226766578634));
#89485=CARTESIAN_POINT('Ctrl Pts',(-1.20097517839325,9.29326286405183,17.4214247553364));
#89486=CARTESIAN_POINT('Ctrl Pts',(-0.998794625944924,9.31776689324801,
17.417998685079));
#89487=CARTESIAN_POINT('Ctrl Pts',(-0.869867223823576,9.33068602629054,
17.4158360257985));
#89488=CARTESIAN_POINT('Ctrl Pts',(-0.389845385362464,9.36875061026307,
17.4078466738288));
#89489=CARTESIAN_POINT('Ctrl Pts',(-0.0376895342458689,9.3767823092476,
17.4021202534462));
#89490=CARTESIAN_POINT('Ctrl Pts',(0.459198076892439,9.36011777438784,17.3939371295269));
#89491=CARTESIAN_POINT('Ctrl Pts',(0.604181764716027,9.35187851683964,17.3915352355229));
#89492=CARTESIAN_POINT('Ctrl Pts',(0.802143936256767,9.33600566197487,17.3882068704053));
#89493=CARTESIAN_POINT('Ctrl Pts',(0.8553355003856,9.331282751013,17.3873076833968));
#89494=CARTESIAN_POINT('Ctrl Pts',(0.950864154843593,9.32197702039714,17.3856819018984));
#89495=CARTESIAN_POINT('Ctrl Pts',(0.993215774129613,9.31755979942169,17.384957101502));
#89496=CARTESIAN_POINT('Ctrl Pts',(1.08994031614121,9.30680458690925,17.3832930709139));
#89497=CARTESIAN_POINT('Ctrl Pts',(1.14429071831867,9.30027850368848,17.3823518758648));
#89498=CARTESIAN_POINT('Ctrl Pts',(1.54549695993146,9.24853377581089,17.3753658993395));
#89499=CARTESIAN_POINT('Ctrl Pts',(1.88963550895892,9.18440066605291,17.3691734691346));
#89500=CARTESIAN_POINT('Ctrl Pts',(2.43983833349401,9.04962562656187,17.359240707693));
#89501=CARTESIAN_POINT('Ctrl Pts',(2.64844483369874,8.99078837493938,17.3554642978226));
#89502=CARTESIAN_POINT('Ctrl Pts',(2.9432811953222,8.8964771745061,17.3501331714831));
#89503=CARTESIAN_POINT('Ctrl Pts',(3.03131267439286,8.86686832175376,17.3485419562679));
#89504=CARTESIAN_POINT('Ctrl Pts',(3.19347262899132,8.80962957948602,17.3456116555802));
#89505=CARTESIAN_POINT('Ctrl Pts',(3.26771946954745,8.78236017605666,17.344270295258));
#89506=CARTESIAN_POINT('Ctrl Pts',(3.43684076487632,8.71780364758471,17.3412144874972));
#89507=CARTESIAN_POINT('Ctrl Pts',(3.5314699299078,8.67990178988407,17.3395043855483));
#89508=CARTESIAN_POINT('Ctrl Pts',(3.85125396758341,8.54572323888136,17.3337174454855));
#89509=CARTESIAN_POINT('Ctrl Pts',(4.0732459106679,8.44216861802731,17.329689109298));
#89510=CARTESIAN_POINT('Ctrl Pts',(4.29092662815677,8.33003803918537,17.3256735943175));
#89511=CARTESIAN_POINT('',(-5.44031476324441,-7.62919132931695,18.));
#89512=CARTESIAN_POINT('Origin',(0.,0.,18.));
#89513=CARTESIAN_POINT('',(-9.37025622235751,0.0001620501840075,17.8485898927132));
#89514=CARTESIAN_POINT('Ctrl Pts',(-9.37024999859875,0.000162049617987492,
17.848589892721));
#89515=CARTESIAN_POINT('Ctrl Pts',(-9.37025401433264,-0.232041092363098,
17.8525347710883));
#89516=CARTESIAN_POINT('Ctrl Pts',(-9.36162238595604,-0.464285151285067,
17.8564796494555));
#89517=CARTESIAN_POINT('Ctrl Pts',(-9.34437206291106,-0.695913652968009,
17.8604245278228));
#89518=CARTESIAN_POINT('Ctrl Pts',(-9.32712467813233,-0.927502701116926,
17.8643687342546));
#89519=CARTESIAN_POINT('Ctrl Pts',(-9.30126155031182,-1.15847611112298,
17.8683129406865));
#89520=CARTESIAN_POINT('Ctrl Pts',(-9.26685163678969,-1.38818075344252,
17.8722571471183));
#89521=CARTESIAN_POINT('Ctrl Pts',(-9.23122356614152,-1.62601724842557,
17.8763409837521));
#89522=CARTESIAN_POINT('Ctrl Pts',(-9.18643257651936,-1.86249318006461,
17.8804248203858));
#89523=CARTESIAN_POINT('Ctrl Pts',(-9.13261349805945,-2.09689192796442,
17.8845086570195));
#89524=CARTESIAN_POINT('Ctrl Pts',(-9.0806330980643,-2.32328266193568,17.8884529731953));
#89525=CARTESIAN_POINT('Ctrl Pts',(-9.02023131849495,-2.54773548938585,
17.8923972893711));
#89526=CARTESIAN_POINT('Ctrl Pts',(-8.95158132950295,-2.76961671785001,
17.8963416055469));
#89527=CARTESIAN_POINT('Ctrl Pts',(-8.8829280686371,-2.99150852122316,17.9002861097097));
#89528=CARTESIAN_POINT('Ctrl Pts',(-8.80602590278989,-3.21082820383465,
17.9042306138725));
#89529=CARTESIAN_POINT('Ctrl Pts',(-8.72109763885253,-3.42695798575075,
17.9081751180353));
#89530=CARTESIAN_POINT('Ctrl Pts',(-8.63614852834321,-3.64314081908745,
17.9121205904198));
#89531=CARTESIAN_POINT('Ctrl Pts',(-8.5431694923091,-3.85613191730517,17.9160660628043));
#89532=CARTESIAN_POINT('Ctrl Pts',(-8.44243160884847,-4.06533314654732,
17.9200115351888));
#89533=CARTESIAN_POINT('Ctrl Pts',(-8.43177899963791,-4.08745530024887,
17.9204287523668));
#89534=CARTESIAN_POINT('Ctrl Pts',(-8.42103967296831,-4.10953509567068,
17.9208459695449));
#89535=CARTESIAN_POINT('Ctrl Pts',(-8.41021397995651,-4.13157184057642,
17.921263186723));
#89536=CARTESIAN_POINT('Ctrl Pts',(-8.30662153564395,-4.34244427774887,
17.9252555913884));
#89537=CARTESIAN_POINT('Ctrl Pts',(-8.19508047047344,-4.54944676716263,
17.9292479960538));
#89538=CARTESIAN_POINT('Ctrl Pts',(-8.0759039439886,-4.75198490632803,17.9332404007192));
#89539=CARTESIAN_POINT('Ctrl Pts',(-7.95674906674446,-4.95448625303896,
17.9372320801367));
#89540=CARTESIAN_POINT('Ctrl Pts',(-7.82996163792674,-5.15252462967349,
17.9412237595541));
#89541=CARTESIAN_POINT('Ctrl Pts',(-7.69589996486297,-5.34553166610415,
17.9452154389716));
#89542=CARTESIAN_POINT('Ctrl Pts',(-7.56185645952786,-5.53851254666648,
17.9492065774459));
#89543=CARTESIAN_POINT('Ctrl Pts',(-7.42054083642917,-5.72646322075847,
17.9531977159202));
#89544=CARTESIAN_POINT('Ctrl Pts',(-7.27235438521001,-5.90884479051674,
17.9571888543944));
#89545=CARTESIAN_POINT('Ctrl Pts',(-7.12416940821138,-6.09122454586719,
17.9611799531632));
#89546=CARTESIAN_POINT('Ctrl Pts',(-6.96911391244025,-6.26803509066209,
17.965171051932));
#89547=CARTESIAN_POINT('Ctrl Pts',(-6.80762984841542,-6.43877013951139,
17.9691621507008));
#89548=CARTESIAN_POINT('Ctrl Pts',(-6.64615731476965,-6.60949299743743,
17.9731529644948));
#89549=CARTESIAN_POINT('Ctrl Pts',(-6.47825732118779,-6.77414102530206,
17.9771437782888));
#89550=CARTESIAN_POINT('Ctrl Pts',(-6.30440966688583,-6.93224377922304,
17.9811345920828));
#89551=CARTESIAN_POINT('Ctrl Pts',(-6.13054820256237,-7.09035909243013,
17.9851257228971));
#89552=CARTESIAN_POINT('Ctrl Pts',(-5.95073833798997,-7.24192790543682,
17.9891168537113));
#89553=CARTESIAN_POINT('Ctrl Pts',(-5.76549496927381,-7.38651831526724,
17.9931079845256));
#89554=CARTESIAN_POINT('Ctrl Pts',(-5.65886686284328,-7.46974613451433,
17.9954053230171));
#89555=CARTESIAN_POINT('Ctrl Pts',(-5.5504391147669,-7.55066254303808,17.9977026615085));
#89556=CARTESIAN_POINT('Ctrl Pts',(-5.44031476324441,-7.62919132931695,
18.));
#89557=CARTESIAN_POINT('Ctrl Pts',(4.29125029737042,8.33066558789285,17.5228836507406));
#89558=CARTESIAN_POINT('Ctrl Pts',(4.20937266281399,8.37289598640675,17.5244488072731));
#89559=CARTESIAN_POINT('Ctrl Pts',(2.7433241481266,9.10149525341159,17.5522595682313));
#89560=CARTESIAN_POINT('Ctrl Pts',(-0.473662841069232,9.74960156866327,
17.6063159336151));
#89561=CARTESIAN_POINT('Ctrl Pts',(-5.04583236791708,8.35587341299396,17.6850527468921));
#89562=CARTESIAN_POINT('Ctrl Pts',(-8.40806015501699,4.95813329461504,17.7637895601691));
#89563=CARTESIAN_POINT('Ctrl Pts',(-9.33992788001211,1.78304083363767,17.81830194184));
#89564=CARTESIAN_POINT('Ctrl Pts',(-9.37097584595092,0.119140517507502,
17.8465687190854));
#89565=CARTESIAN_POINT('Ctrl Pts',(-9.37090218672064,0.000162108931356462,
17.848589891905));
#89566=CARTESIAN_POINT('Ctrl Pts',(-4.05890219815148,8.44447251167999,3.66935213444816));
#89567=CARTESIAN_POINT('Ctrl Pts',(-5.45144634927424,7.77513520159967,3.69559773887382));
#89568=CARTESIAN_POINT('Ctrl Pts',(-7.89776706951283,5.73514866702576,3.74808894772514));
#89569=CARTESIAN_POINT('Ctrl Pts',(-9.67358643625363,1.29694711723465,3.82682576100211));
#89570=CARTESIAN_POINT('Ctrl Pts',(-9.12961484805542,-3.45099953375481,
3.90556257427908));
#89571=CARTESIAN_POINT('Ctrl Pts',(-6.39647197105479,-7.37203461182231,
3.98429938755606));
#89572=CARTESIAN_POINT('Ctrl Pts',(-2.12945660839726,-9.52497797369592,
4.06303620083303));
#89573=CARTESIAN_POINT('Ctrl Pts',(2.64817455363187,-9.39404484874638,4.14177301411));
#89574=CARTESIAN_POINT('Ctrl Pts',(6.79079602168952,-7.01038540771718,4.22050982738697));
#89575=CARTESIAN_POINT('Ctrl Pts',(9.30501602531431,-2.94571581100747,4.29924664066395));
#89576=CARTESIAN_POINT('Ctrl Pts',(9.58794458405767,1.82534318116471,4.37798345394092));
#89577=CARTESIAN_POINT('Ctrl Pts',(7.57173346773308,6.15868302513809,4.4567202672179));
#89578=CARTESIAN_POINT('Ctrl Pts',(3.73986123984316,9.01520910973077,4.53545708049487));
#89579=CARTESIAN_POINT('Ctrl Pts',(-0.988810284069998,9.70993258668408,
4.61419389377184));
#89580=CARTESIAN_POINT('Ctrl Pts',(-5.48037016060699,8.07626705693223,4.69293070704882));
#89581=CARTESIAN_POINT('Ctrl Pts',(-8.65776628439157,4.50595450829045,4.77166752032579));
#89582=CARTESIAN_POINT('Ctrl Pts',(-9.75907571166627,-0.144861728555519,
4.85040433360277));
#89583=CARTESIAN_POINT('Ctrl Pts',(-8.52021031990554,-4.76094110276756,
4.92914114687973));
#89584=CARTESIAN_POINT('Ctrl Pts',(-5.23824345717932,-8.23537182090993,
5.00787796015672));
#89585=CARTESIAN_POINT('Ctrl Pts',(-0.70017347004904,-9.73500390508311,
5.08661477343368));
#89586=CARTESIAN_POINT('Ctrl Pts',(4.00579442225045,-8.90023341090876,5.16535158671067));
#89587=CARTESIAN_POINT('Ctrl Pts',(7.75119395567349,-5.93123394107183,5.24408839998763));
#89588=CARTESIAN_POINT('Ctrl Pts',(9.63789809505959,-1.53995587317032,5.3228252132646));
#89589=CARTESIAN_POINT('Ctrl Pts',(9.21348514579648,3.22059548021945,5.40156202654158));
#89590=CARTESIAN_POINT('Ctrl Pts',(6.57972709342064,7.20886503988206,5.48029883981855));
#89591=CARTESIAN_POINT('Ctrl Pts',(2.36818521591906,9.46848681488684,5.55903565309553));
#89592=CARTESIAN_POINT('Ctrl Pts',(-2.41123497551512,9.45761543293126,5.63777246637249));
#89593=CARTESIAN_POINT('Ctrl Pts',(-6.61245374788223,7.17885779318626,5.71650927964948));
#89594=CARTESIAN_POINT('Ctrl Pts',(-9.22804101623034,3.17864794936077,5.79524609292644));
#89595=CARTESIAN_POINT('Ctrl Pts',(-9.63079276036606,-1.5837848938706,5.87398290620342));
#89596=CARTESIAN_POINT('Ctrl Pts',(-7.72413123801395,-5.96643447973725,
5.95271971948039));
#89597=CARTESIAN_POINT('Ctrl Pts',(-3.96526381766737,-8.9183645720204,6.03145653275737));
#89598=CARTESIAN_POINT('Ctrl Pts',(0.744452934971506,-9.73171791672532,
6.11019334603434));
#89599=CARTESIAN_POINT('Ctrl Pts',(5.27565380349995,-8.21145667520394,6.18893015931131));
#89600=CARTESIAN_POINT('Ctrl Pts',(8.54178073820683,-4.72213146825887,6.26766697258829));
#89601=CARTESIAN_POINT('Ctrl Pts',(9.75963374084516,-0.100464061641155,
6.34640378586526));
#89602=CARTESIAN_POINT('Ctrl Pts',(8.63717808998542,4.54529409664561,6.42514059914223));
#89603=CARTESIAN_POINT('Ctrl Pts',(5.44357272566864,8.10111472351062,6.50387741241921));
#89604=CARTESIAN_POINT('Ctrl Pts',(0.944627356376894,9.71433080251592,6.58261422569617));
#89605=CARTESIAN_POINT('Ctrl Pts',(-3.7808346666298,8.99810163349664,6.66135103897316));
#89606=CARTESIAN_POINT('Ctrl Pts',(-7.59967249422965,6.12417519047048,6.74008785225012));
#89607=CARTESIAN_POINT('Ctrl Pts',(-9.59614897362004,1.78170386406272,6.81882466552711));
#89608=CARTESIAN_POINT('Ctrl Pts',(-9.29151958371627,-2.98801064398065,
6.89756147880407));
#89609=CARTESIAN_POINT('Ctrl Pts',(-6.75883284418958,-7.04121597221882,
6.97629829208105));
#89610=CARTESIAN_POINT('Ctrl Pts',(-2.60541366604633,-9.40597487833683,
7.05503510535802));
#89611=CARTESIAN_POINT('Ctrl Pts',(2.17276995618375,-9.5152306593498,7.133771918635));
#89612=CARTESIAN_POINT('Ctrl Pts',(6.42993481218324,-7.34278435569223,7.21250873191196));
#89613=CARTESIAN_POINT('Ctrl Pts',(9.14523524150828,-3.40957712342747,7.29124554518895));
#89614=CARTESIAN_POINT('Ctrl Pts',(9.66755653428997,1.34122870511777,7.36998235846591));
#89615=CARTESIAN_POINT('Ctrl Pts',(7.87164880166345,5.77041497003424,7.44871917174289));
#89616=CARTESIAN_POINT('Ctrl Pts',(4.18816123796882,8.81588618505821,7.52745598501985));
#89617=CARTESIAN_POINT('Ctrl Pts',(-0.499625282810953,9.74735442876174,
7.60619279829684));
#89618=CARTESIAN_POINT('Ctrl Pts',(-5.0676042981128,8.34145853318671,7.6849296115738));
#89619=CARTESIAN_POINT('Ctrl Pts',(-8.42039855276698,4.93532491287903,7.76366642485078));
#89620=CARTESIAN_POINT('Ctrl Pts',(-9.75402568268881,0.34572643024801,7.84240323812776));
#89621=CARTESIAN_POINT('Ctrl Pts',(-8.74868894185552,-4.32677542539241,
7.92114005140473));
#89622=CARTESIAN_POINT('Ctrl Pts',(-5.64546277391199,-7.96173937349739,
7.9998768646817));
#89623=CARTESIAN_POINT('Ctrl Pts',(-1.18848443312888,-9.68752024696387,
8.07861367795868));
#89624=CARTESIAN_POINT('Ctrl Pts',(3.5534862011415,-9.0902849021041,8.15735049123564));
#89625=CARTESIAN_POINT('Ctrl Pts',(7.44334960193927,-6.31324722202728,8.23608730451263));
#89626=CARTESIAN_POINT('Ctrl Pts',(9.54833705892713,-2.02232618344405,8.31482411778959));
#89627=CARTESIAN_POINT('Ctrl Pts',(9.36368369138254,2.75353799880477,8.39356093106657));
#89628=CARTESIAN_POINT('Ctrl Pts',(6.93366840212465,6.86911830386571,8.47229774434354));
#89629=CARTESIAN_POINT('Ctrl Pts',(2.84099603035075,9.33752029923663,8.55103455762052));
#89630=CARTESIAN_POINT('Ctrl Pts',(-1.93293219291658,9.56683421622385,8.62977137089749));
#89631=CARTESIAN_POINT('Ctrl Pts',(-6.24335347956852,7.50207178799861,8.70850818417446));
#89632=CARTESIAN_POINT('Ctrl Pts',(-9.05665155821197,3.63835214571946,8.78724499745144));
#89633=CARTESIAN_POINT('Ctrl Pts',(-9.69821239996552,-1.09782513556562,
8.86598181072841));
#89634=CARTESIAN_POINT('Ctrl Pts',(-8.01419310154301,-5.57074974436163,
8.94471862400538));
#89635=CARTESIAN_POINT('Ctrl Pts',(-4.40841260138079,-8.70783797042137,
9.02345543728235));
#89636=CARTESIAN_POINT('Ctrl Pts',(0.254481970185954,-9.7568326166833,9.10219225055933));
#89637=CARTESIAN_POINT('Ctrl Pts',(4.85635310861981,-8.46619030423503,9.1809290638363));
#89638=CARTESIAN_POINT('Ctrl Pts',(8.2936964065283,-5.14540024677036,9.25966587711328));
#89639=CARTESIAN_POINT('Ctrl Pts',(9.74225508555788,-0.590770370826471,
9.33840269039025));
#89640=CARTESIAN_POINT('Ctrl Pts',(8.85467242089165,4.10552312157971,9.41713950366722));
#89641=CARTESIAN_POINT('Ctrl Pts',(5.84378605029053,7.81733384099428,9.4958763169442));
#89642=CARTESIAN_POINT('Ctrl Pts',(1.43159063205072,9.65458917020032,9.57461313022116));
#89643=CARTESIAN_POINT('Ctrl Pts',(-3.32389266290867,9.17672497945682,9.65334994349815));
#89644=CARTESIAN_POINT('Ctrl Pts',(-7.28232404292288,6.49833057923279,9.73208675677511));
#89645=CARTESIAN_POINT('Ctrl Pts',(-9.49449255818395,2.26167080843221,9.81082357005209));
#89646=CARTESIAN_POINT('Ctrl Pts',(-9.42993187596523,-2.51732568369289,
9.88956038332907));
#89647=CARTESIAN_POINT('Ctrl Pts',(-7.10412330707039,-6.69268076491505,
9.96829719660603));
#89648=CARTESIAN_POINT('Ctrl Pts',(-3.07478346922299,-9.26316632693798,
10.047034009883));
#89649=CARTESIAN_POINT('Ctrl Pts',(1.69187321388056,-9.61239350064688,10.12577082316));
#89650=CARTESIAN_POINT('Ctrl Pts',(6.05282763107886,-7.65661945322955,10.2045076364369));
#89651=CARTESIAN_POINT('Ctrl Pts',(8.96234593301987,-3.86482847743687,10.2832444497139));
#89652=CARTESIAN_POINT('Ctrl Pts',(9.72274098918695,0.853727966221407,10.3619812629909));
#89653=CARTESIAN_POINT('Ctrl Pts',(8.15167407896019,5.36756495009922,10.4407180762679));
#89654=CARTESIAN_POINT('Ctrl Pts',(4.6258787543211,8.59428819236621,10.5194548895448));
#89655=CARTESIAN_POINT('Ctrl Pts',(-0.00917787727279524,9.76014649222507,
10.5981917028218));
#89656=CARTESIAN_POINT('Ctrl Pts',(-4.64203370234336,8.5855731835116,10.6769285160988));
#89657=CARTESIAN_POINT('Ctrl Pts',(-8.16175434919945,5.35222474550992,10.7556653293757));
#89658=CARTESIAN_POINT('Ctrl Pts',(-9.72432938604995,0.83544106598262,10.8344021426527));
#89659=CARTESIAN_POINT('Ctrl Pts',(-8.9550615673234,-3.88167697117781,10.9131389559297));
#89660=CARTESIAN_POINT('Ctrl Pts',(-6.03841725526543,-7.6679893606106,10.9918757692066));
#89661=CARTESIAN_POINT('Ctrl Pts',(-1.67379236000308,-9.61555837789571,
11.0706125824837));
#89662=CARTESIAN_POINT('Ctrl Pts',(3.09219910784695,-9.25736725319652,11.1493493957606));
#89663=CARTESIAN_POINT('Ctrl Pts',(7.11669755222962,-6.67930832745529,11.2280862090376));
#89664=CARTESIAN_POINT('Ctrl Pts',(9.43464949004539,-2.49958652242944,11.3068230223146));
#89665=CARTESIAN_POINT('Ctrl Pts',(9.49022228223122,2.27952293626696,11.3855598355915));
#89666=CARTESIAN_POINT('Ctrl Pts',(7.27008986656942,6.51201482761895,11.4642966488685));
#89667=CARTESIAN_POINT('Ctrl Pts',(3.30662827706433,9.18295993786554,11.5430334621455));
#89668=CARTESIAN_POINT('Ctrl Pts',(-1.44974531879287,9.65187972851728,11.6217702754224));
#89669=CARTESIAN_POINT('Ctrl Pts',(-5.85847763988178,7.80632970903293,11.7005070886994));
#89670=CARTESIAN_POINT('Ctrl Pts',(-8.86237794769954,4.08886303209752,11.7792439019764));
#89671=CARTESIAN_POINT('Ctrl Pts',(-9.74112680492853,-0.609091416314159,
11.8579807152534));
#89672=CARTESIAN_POINT('Ctrl Pts',(-8.28400487420087,-5.16098895826575,
11.9367175285304));
#89673=CARTESIAN_POINT('Ctrl Pts',(-4.84042230288836,-8.47530859100871,
12.0154543418073));
#89674=CARTESIAN_POINT('Ctrl Pts',(-0.236132014171883,-9.75729396169901,
12.0941911550843));
#89675=CARTESIAN_POINT('Ctrl Pts',(4.42478148508795,-8.6995317455796,12.1729279683613));
#89676=CARTESIAN_POINT('Ctrl Pts',(8.02465574103572,-5.555667738534,12.2516647816382));
#89677=CARTESIAN_POINT('Ctrl Pts',(9.7002599095219,-1.07958393413709,12.3304015949152));
#89678=CARTESIAN_POINT('Ctrl Pts',(9.04979295584846,3.65537839893496,12.4091384081922));
#89679=CARTESIAN_POINT('Ctrl Pts',(6.22923342192782,7.51380028735541,12.4878752214692));
#89680=CARTESIAN_POINT('Ctrl Pts',(1.91493659528631,9.57045252948668,12.5666120347461));
#89681=CARTESIAN_POINT('Ctrl Pts',(-2.85855191865109,9.33216077398482,12.6453488480231));
#89682=CARTESIAN_POINT('Ctrl Pts',(-6.94657477175178,6.85606612596367,12.7240856613001));
#89683=CARTESIAN_POINT('Ctrl Pts',(-9.36884566302788,2.73592301161571,12.802822474577));
#89684=CARTESIAN_POINT('Ctrl Pts',(-9.54451681903836,-2.04027999897532,
12.881559287854));
#89685=CARTESIAN_POINT('Ctrl Pts',(-7.43146322387599,-6.32723463570806,
12.960296101131));
#89686=CARTESIAN_POINT('Ctrl Pts',(-3.53638397561942,-9.09695180596813,
13.039032914408));
#89687=CARTESIAN_POINT('Ctrl Pts',(1.20670148270599,-9.68526795265676,13.1177697276849));
#89688=CARTESIAN_POINT('Ctrl Pts',(5.66042629521671,-7.95110796930491,13.1965065409619));
#89689=CARTESIAN_POINT('Ctrl Pts',(8.75681076146596,-4.3103142659206,13.2752433542389));
#89690=CARTESIAN_POINT('Ctrl Pts',(9.7533582311345,0.364070045850259,13.3539801675159));
#89691=CARTESIAN_POINT('Ctrl Pts',(8.41110188140746,4.9511522824196,13.4327169807928));
#89692=CARTESIAN_POINT('Ctrl Pts',(5.05190769966626,8.35097433699671,13.5114537940698));
#89693=CARTESIAN_POINT('Ctrl Pts',(0.481292718728248,9.74827682731795,13.5901906073468));
#89694=CARTESIAN_POINT('Ctrl Pts',(-4.20473371559156,8.80799399205588,13.6689274206238));
#89695=CARTESIAN_POINT('Ctrl Pts',(-7.88248720017234,5.75560069169532,13.7476642339007));
#89696=CARTESIAN_POINT('Ctrl Pts',(-9.67006186293461,1.32304472718883,13.8264010471777));
#89697=CARTESIAN_POINT('Ctrl Pts',(-9.13880673570443,-3.42677037902575,
13.9051378604547));
#89698=CARTESIAN_POINT('Ctrl Pts',(-6.4161139936889,-7.35486403702436,13.9838746737316));
#89699=CARTESIAN_POINT('Ctrl Pts',(-2.15487098431875,-9.51930012259652,
14.0626114870086));
#89700=CARTESIAN_POINT('Ctrl Pts',(2.62309871231088,-9.4010582876928,14.1413483002856));
#89701=CARTESIAN_POINT('Ctrl Pts',(6.77206318411236,-7.02849230016758,14.2200851135626));
#89702=CARTESIAN_POINT('Ctrl Pts',(9.29712265162198,-2.97053095991647,14.2988219268396));
#89703=CARTESIAN_POINT('Ctrl Pts',(9.59278118340142,1.79974802417014,14.3775587401165));
#89704=CARTESIAN_POINT('Ctrl Pts',(7.58814142420382,6.13845693227594,14.4562955533935));
#89705=CARTESIAN_POINT('Ctrl Pts',(3.76390540652066,9.00519627070335,14.5350323666704));
#89706=CARTESIAN_POINT('Ctrl Pts',(-0.962895259358665,9.71253707857168,
14.6137691799475));
#89707=CARTESIAN_POINT('Ctrl Pts',(-5.4587987248176,8.09086276394888,14.6925059932244));
#89708=CARTESIAN_POINT('Ctrl Pts',(-8.64571107107811,4.52904226725275,14.7712428065014));
#89709=CARTESIAN_POINT('Ctrl Pts',(-9.7594275400581,-0.118818657963835,
14.8499796197784));
#89710=CARTESIAN_POINT('Ctrl Pts',(-8.53288480140027,-4.73818749620118,
14.9287164330553));
#89711=CARTESIAN_POINT('Ctrl Pts',(-5.26020132936178,-8.22136398401781,
15.0074532463323));
#89712=CARTESIAN_POINT('Ctrl Pts',(-0.726149345231843,-9.73310078605705,
15.0861900596093));
#89713=CARTESIAN_POINT('Ctrl Pts',(3.98202941880643,-8.91089139709851,15.1649268728862));
#89714=CARTESIAN_POINT('Ctrl Pts',(7.73533854789984,-5.95189728847034,15.2436636861632));
#89715=CARTESIAN_POINT('Ctrl Pts',(9.63375432524542,-1.56566962796746,15.3224004994402));
#89716=CARTESIAN_POINT('Ctrl Pts',(9.22204666848199,3.19599734472079,15.4011373127172));
#89717=CARTESIAN_POINT('Ctrl Pts',(6.59894090044666,7.19128102465388,15.4798741259942));
#89718=CARTESIAN_POINT('Ctrl Pts',(2.39344393789276,9.46213347502903,15.5586109392711));
#89719=CARTESIAN_POINT('Ctrl Pts',(-2.3859882468475,9.46401626525843,15.6373477525481));
#89720=CARTESIAN_POINT('Ctrl Pts',(-6.59327304475852,7.19647791216796,15.7160845658251));
#89721=CARTESIAN_POINT('Ctrl Pts',(-9.21952577002525,3.20326214334899,15.7948213791021));
#89722=CARTESIAN_POINT('Ctrl Pts',(-9.63498488216568,-1.55807897862842,
15.873558192379));
#89723=CARTESIAN_POINT('Ctrl Pts',(-7.74002547913806,-5.94580098598721,
15.952295005656));
#89724=CARTESIAN_POINT('Ctrl Pts',(-3.98904882300254,-8.90775130277384,
16.031031818933));
#89725=CARTESIAN_POINT('Ctrl Pts',(0.718480684171045,-9.73366987764925,
16.1097686322099));
#89726=CARTESIAN_POINT('Ctrl Pts',(5.25372231584012,-8.22550579692042,16.1885054454869));
#89727=CARTESIAN_POINT('Ctrl Pts',(8.52914906873457,-4.74490884446967,16.2672422587639));
#89728=CARTESIAN_POINT('Ctrl Pts',(9.75933089707706,-0.126507799846194,
16.3459790720408));
#89729=CARTESIAN_POINT('Ctrl Pts',(8.64927669253978,4.52222915143409,16.4247158853178));
#89730=CARTESIAN_POINT('Ctrl Pts',(5.46517159297118,8.08655941555927,16.5034526985948));
#89731=CARTESIAN_POINT('Ctrl Pts',(0.970547195120261,9.71177543306001,16.5821895118718));
#89732=CARTESIAN_POINT('Ctrl Pts',(-3.75680929901023,9.0081589371075,16.6609263251487));
#89733=CARTESIAN_POINT('Ctrl Pts',(-7.58330275007955,6.14443353614328,16.7396631384257));
#89734=CARTESIAN_POINT('Ctrl Pts',(-9.5913602389158,1.80730529622961,16.8183999517027));
#89735=CARTESIAN_POINT('Ctrl Pts',(-9.29946015674463,-2.96320499781051,
16.8971367649797));
#89736=CARTESIAN_POINT('Ctrl Pts',(-6.77759864659425,-7.02315479381199,
16.9758735782566));
#89737=CARTESIAN_POINT('Ctrl Pts',(-2.63050470092249,-9.39898833036069,
17.0546103915336));
#89738=CARTESIAN_POINT('Ctrl Pts',(2.14737027682777,-9.52099565589916,17.1333472048106));
#89739=CARTESIAN_POINT('Ctrl Pts',(6.41031741029837,-7.35991542137126,17.2120840180876));
#89740=CARTESIAN_POINT('Ctrl Pts',(9.13610385335678,-3.43397225624563,17.2908208313645));
#89741=CARTESIAN_POINT('Ctrl Pts',(9.67110162026351,1.31543084999252,17.3695576446415));
#89742=CARTESIAN_POINT('Ctrl Pts',(7.88701871315299,5.74937822649567,17.4482944579185));
#89743=CARTESIAN_POINT('Ctrl Pts',(4.21167337024702,8.80469843374058,17.5270312711955));
#89744=CARTESIAN_POINT('Ctrl Pts',(-0.473614874379152,9.74861425009761,
17.6057680844724));
#89745=CARTESIAN_POINT('Ctrl Pts',(-5.04532138867952,8.35502723390706,17.6845048977494));
#89746=CARTESIAN_POINT('Ctrl Pts',(-8.40720869110497,4.95763119645048,17.7632417110264));
#89747=CARTESIAN_POINT('Ctrl Pts',(-9.75304724334012,0.372042784836709,
17.8419785243033));
#89748=CARTESIAN_POINT('Ctrl Pts',(-8.76018319001389,-4.30436209043516,
17.9207211504403));
#89749=CARTESIAN_POINT('Ctrl Pts',(-6.69727900373269,-6.7319066656312,17.9732181721515));
#89750=CARTESIAN_POINT('Ctrl Pts',(-5.43892795783426,-7.62901472696143,
17.9994695894372));
#89751=CARTESIAN_POINT('Ctrl Pts',(-4.14169175030982,8.61671467552761,3.77968718924866));
#89752=CARTESIAN_POINT('Ctrl Pts',(-5.5626396670332,7.9337248718815,3.80593279367432));
#89753=CARTESIAN_POINT('Ctrl Pts',(-8.05885806575159,5.85212866962865,3.85842400252563));
#89754=CARTESIAN_POINT('Ctrl Pts',(-9.8708988743772,1.32340098721405,3.93716081580261));
#89755=CARTESIAN_POINT('Ctrl Pts',(-9.31583188107312,-3.52138967669254,
4.01589762907957));
#89756=CARTESIAN_POINT('Ctrl Pts',(-6.52694100529715,-7.52240222705742,
4.09463444235655));
#89757=CARTESIAN_POINT('Ctrl Pts',(-2.17289119990582,-9.71925924046788,
4.17337125563352));
#89758=CARTESIAN_POINT('Ctrl Pts',(2.70218945091914,-9.585655468568,4.2521080689105));
#89759=CARTESIAN_POINT('Ctrl Pts',(6.92930809564152,-7.15337645308571,4.33084488218747));
#89760=CARTESIAN_POINT('Ctrl Pts',(9.49481072150404,-3.00579966641305,4.40958169546445));
#89761=CARTESIAN_POINT('Ctrl Pts',(9.78351018270518,1.86257476180559,4.48831850874142));
#89762=CARTESIAN_POINT('Ctrl Pts',(7.72617434663415,6.28430187098475,4.56705532201839));
#89763=CARTESIAN_POINT('Ctrl Pts',(3.81614330382639,9.19909260540809,4.64579213529537));
#89764=CARTESIAN_POINT('Ctrl Pts',(-1.00897907764797,9.90798637834857,4.72452894857234));
#89765=CARTESIAN_POINT('Ctrl Pts',(-5.59215343822949,8.24099892286858,4.80326576184931));
#89766=CARTESIAN_POINT('Ctrl Pts',(-8.8343590078385,4.59786260007872,4.88200257512628));
#89767=CARTESIAN_POINT('Ctrl Pts',(-9.95813187715264,-0.147816477659208,
4.96073938840327));
#89768=CARTESIAN_POINT('Ctrl Pts',(-8.69399731014175,-4.85805016391465,
5.03947620168022));
#89769=CARTESIAN_POINT('Ctrl Pts',(-5.34508806903368,-8.40334895157867,
5.11821301495721));
#89770=CARTESIAN_POINT('Ctrl Pts',(-0.714454929711948,-9.93356907719506,
5.19694982823418));
#89771=CARTESIAN_POINT('Ctrl Pts',(4.08750073348098,-9.08177174374406,5.27568664151115));
#89772=CARTESIAN_POINT('Ctrl Pts',(7.90929529563061,-6.05221350100097,5.35442345478813));
#89773=CARTESIAN_POINT('Ctrl Pts',(9.83448259699735,-1.57136640016983,5.43316026806509));
#89774=CARTESIAN_POINT('Ctrl Pts',(9.4014128838399,3.28628606463705,5.51189708134208));
#89775=CARTESIAN_POINT('Ctrl Pts',(6.71393398799339,7.35590448037256,5.59063389461904));
#89776=CARTESIAN_POINT('Ctrl Pts',(2.41648916212977,9.66161582976643,5.66937070789602));
#89777=CARTESIAN_POINT('Ctrl Pts',(-2.46041700898769,9.65052270390096,5.74810752117299));
#89778=CARTESIAN_POINT('Ctrl Pts',(-6.74732816902602,7.325285174949,5.82684433444997));
#89779=CARTESIAN_POINT('Ctrl Pts',(-9.41626565080774,3.24348292870976,5.90558114772694));
#89780=CARTESIAN_POINT('Ctrl Pts',(-9.82723233457501,-1.61608940274454,
5.98431796100391));
#89781=CARTESIAN_POINT('Ctrl Pts',(-7.88168057889206,-6.08813202612909,
6.06305477428089));
#89782=CARTESIAN_POINT('Ctrl Pts',(-4.04614342491783,-9.10027272670288,
6.14179158755786));
#89783=CARTESIAN_POINT('Ctrl Pts',(0.759637564233405,-9.93021606443235,
6.22052840083484));
#89784=CARTESIAN_POINT('Ctrl Pts',(5.38326147533128,-8.37894600791499,6.29926521411181));
#89785=CARTESIAN_POINT('Ctrl Pts',(8.71600770092424,-4.81844892810506,6.37800202738878));
#89786=CARTESIAN_POINT('Ctrl Pts',(9.95870128846972,-0.102513230176209,
6.45673884066575));
#89787=CARTESIAN_POINT('Ctrl Pts',(8.813350875402,4.63800459921958,6.53547565394273));
#89788=CARTESIAN_POINT('Ctrl Pts',(5.55460544488635,8.2663534080614,6.6142124672197));
#89789=CARTESIAN_POINT('Ctrl Pts',(0.963894949428697,9.91247430472313,6.69294928049667));
#89790=CARTESIAN_POINT('Ctrl Pts',(-3.85795246685114,9.18163618745848,6.77168609377365));
#89791=CARTESIAN_POINT('Ctrl Pts',(-7.75468324630784,6.24909017895906,6.85042290705061));
#89792=CARTESIAN_POINT('Ctrl Pts',(-9.79188191745213,1.81804533221925,6.92915972032761));
#89793=CARTESIAN_POINT('Ctrl Pts',(-9.48103899257435,-3.0489571883867,7.00789653360456));
#89794=CARTESIAN_POINT('Ctrl Pts',(-6.89669296423347,-7.18483586955351,
7.08663334688156));
#89795=CARTESIAN_POINT('Ctrl Pts',(-2.65855636820297,-9.59782883533654,
7.1653701601585));
#89796=CARTESIAN_POINT('Ctrl Pts',(2.21708801137054,-9.70931310985319,7.2441069734355));
#89797=CARTESIAN_POINT('Ctrl Pts',(6.56108638901859,-7.49255535255931,7.32284378671246));
#89798=CARTESIAN_POINT('Ctrl Pts',(9.33177088416849,-3.47912237219609,7.40158059998944));
#89799=CARTESIAN_POINT('Ctrl Pts',(9.86474598031898,1.36858578799824,7.48031741326641));
#89800=CARTESIAN_POINT('Ctrl Pts',(8.03220706279482,5.88811430049716,7.55905422654339));
#89801=CARTESIAN_POINT('Ctrl Pts',(4.27358729071193,8.99570408495051,7.63779103982036));
#89802=CARTESIAN_POINT('Ctrl Pts',(-0.509816154970842,9.94617151488255,
7.71652785309733));
#89803=CARTESIAN_POINT('Ctrl Pts',(-5.17096837782566,8.51159951776734,7.7952646663743));
#89804=CARTESIAN_POINT('Ctrl Pts',(-8.59214967933906,5.03599088592941,7.87400147965128));
#89805=CARTESIAN_POINT('Ctrl Pts',(-9.9529788425798,0.352778222809711,7.95273829292826));
#89806=CARTESIAN_POINT('Ctrl Pts',(-8.92713621752499,-4.41502879595184,
8.03147510620521));
#89807=CARTESIAN_POINT('Ctrl Pts',(-5.76061345061262,-8.12413521477522,
8.11021191948221));
#89808=CARTESIAN_POINT('Ctrl Pts',(-1.21272598642642,-9.88511689345029,
8.18894873275916));
#89809=CARTESIAN_POINT('Ctrl Pts',(3.62596676776546,-9.27569972101245,8.26768554603615));
#89810=CARTESIAN_POINT('Ctrl Pts',(7.59517183120687,-6.44201871852076,8.34642235931312));
#89811=CARTESIAN_POINT('Ctrl Pts',(9.7430947816743,-2.06357563240139,8.42515917259009));
#89812=CARTESIAN_POINT('Ctrl Pts',(9.5546750337497,2.80970199750268,8.50389598586707));
#89813=CARTESIAN_POINT('Ctrl Pts',(7.07509464838597,7.00922791980045,8.58263279914403));
#89814=CARTESIAN_POINT('Ctrl Pts',(2.89894391319049,9.52797798609473,8.66136961242102));
#89815=CARTESIAN_POINT('Ctrl Pts',(-1.97235826991761,9.76196922605361,8.74010642569798));
#89816=CARTESIAN_POINT('Ctrl Pts',(-6.37069935126138,7.65509177548957,8.81884323897496));
#89817=CARTESIAN_POINT('Ctrl Pts',(-9.24138035677726,3.71256372560816,8.89758005225193));
#89818=CARTESIAN_POINT('Ctrl Pts',(-9.89602713462341,-1.12021750840057,
8.97631686552891));
#89819=CARTESIAN_POINT('Ctrl Pts',(-8.17765884311456,-5.68437649711558,
9.05505367880587));
#89820=CARTESIAN_POINT('Ctrl Pts',(-4.49833112791335,-8.88545200757823,
9.13379049208287));
#89821=CARTESIAN_POINT('Ctrl Pts',(0.259672646707696,-9.95584302969276,
9.21252730535982));
#89822=CARTESIAN_POINT('Ctrl Pts',(4.95540829136565,-8.638875446561,9.2912641186368));
#89823=CARTESIAN_POINT('Ctrl Pts',(8.46286318555204,-5.25035113282513,9.37000093191377));
#89824=CARTESIAN_POINT('Ctrl Pts',(9.94096816021956,-0.602820332131643,
9.44873774519074));
#89825=CARTESIAN_POINT('Ctrl Pts',(9.03528144482141,4.18926360213774,9.52747455846772));
#89826=CARTESIAN_POINT('Ctrl Pts',(5.96298193291937,7.97678423821325,9.60621137174469));
#89827=CARTESIAN_POINT('Ctrl Pts',(1.46079082991595,9.85151412050775,9.68494818502168));
#89828=CARTESIAN_POINT('Ctrl Pts',(-3.39169020311791,9.36390291926418,9.76368499829864));
#89829=CARTESIAN_POINT('Ctrl Pts',(-7.43086182894297,6.63087722661854,9.84242181157562));
#89830=CARTESIAN_POINT('Ctrl Pts',(-9.6881520130042,2.30780217701878,9.92115862485258));
#89831=CARTESIAN_POINT('Ctrl Pts',(-9.62227448457758,-2.56867165258183,
9.99989543812957));
#89832=CARTESIAN_POINT('Ctrl Pts',(-7.24902632723626,-6.82919157897666,
10.0786322514066));
#89833=CARTESIAN_POINT('Ctrl Pts',(-3.13749992159695,-9.45210741355117,
10.1573690646836));
#89834=CARTESIAN_POINT('Ctrl Pts',(1.72638240352046,-9.80845778459312,10.2361058779605));
#89835=CARTESIAN_POINT('Ctrl Pts',(6.17628734121842,-7.81279175417053,10.3148426912375));
#89836=CARTESIAN_POINT('Ctrl Pts',(9.14515117686653,-3.94365950198376,10.3935795045144));
#89837=CARTESIAN_POINT('Ctrl Pts',(9.92105603422868,0.871141481634682,10.4723163177914));
#89838=CARTESIAN_POINT('Ctrl Pts',(8.31794402422896,5.47704733639615,10.5510531310684));
#89839=CARTESIAN_POINT('Ctrl Pts',(4.72023294462003,8.76958615123051,10.6297899443454));
#89840=CARTESIAN_POINT('Ctrl Pts',(-0.00936507871595034,9.95922449845521,
10.7085267576224));
#89841=CARTESIAN_POINT('Ctrl Pts',(-4.73671740561069,8.76069338207398,10.7872635708993));
#89842=CARTESIAN_POINT('Ctrl Pts',(-8.32822990204828,5.46139423718515,10.8660003841763));
#89843=CARTESIAN_POINT('Ctrl Pts',(-9.92267682967102,0.852481582932977,
10.9447371974533));
#89844=CARTESIAN_POINT('Ctrl Pts',(-9.13771823174039,-3.9608516549663,11.0234740107302));
#89845=CARTESIAN_POINT('Ctrl Pts',(-6.16158303652923,-7.82439357389984,
11.1022108240072));
#89846=CARTESIAN_POINT('Ctrl Pts',(-1.707932753914,-9.81168721593988,11.1809476372842));
#89847=CARTESIAN_POINT('Ctrl Pts',(3.15527078753404,-9.44619005592542,11.2596844505612));
#89848=CARTESIAN_POINT('Ctrl Pts',(7.2618570496582,-6.81554638350144,11.3384212638381));
#89849=CARTESIAN_POINT('Ctrl Pts',(9.62708832397628,-2.5505706651041,11.4171580771151));
#89850=CARTESIAN_POINT('Ctrl Pts',(9.6837946361024,2.32601843525042,11.4958948903921));
#89851=CARTESIAN_POINT('Ctrl Pts',(7.41837811172063,6.64484059303715,11.5746317036691));
#89852=CARTESIAN_POINT('Ctrl Pts',(3.37407367506801,9.37026505231005,11.653368516946));
#89853=CARTESIAN_POINT('Ctrl Pts',(-1.47931581835828,9.84874941425992,11.732105330223));
#89854=CARTESIAN_POINT('Ctrl Pts',(-5.97797318731239,7.96555565463604,11.8108421435));
#89855=CARTESIAN_POINT('Ctrl Pts',(-9.04314414149503,4.17226369630137,11.8895789567769));
#89856=CARTESIAN_POINT('Ctrl Pts',(-9.93981686601572,-0.621515072543928,
11.9683157700539));
#89857=CARTESIAN_POINT('Ctrl Pts',(-8.45297397474363,-5.26625780774518,
12.0470525833309));
#89858=CARTESIAN_POINT('Ctrl Pts',(-4.93915254450293,-8.64817971930859,
12.1257893966079));
#89859=CARTESIAN_POINT('Ctrl Pts',(-0.240948406080153,-9.95631378477686,
12.2045262098849));
#89860=CARTESIAN_POINT('Ctrl Pts',(4.51503388824163,-8.87697636041459,12.2832630231618));
#89861=CARTESIAN_POINT('Ctrl Pts',(8.18833488938468,-5.66898686315428,12.3619998364388));
#89862=CARTESIAN_POINT('Ctrl Pts',(9.89811640729478,-1.10160424062915,12.4407366497158));
#89863=CARTESIAN_POINT('Ctrl Pts',(9.23438185929177,3.72993726383072,12.5194734629927));
#89864=CARTESIAN_POINT('Ctrl Pts',(6.35629128637356,7.66705950140611,12.5982102762697));
#89865=CARTESIAN_POINT('Ctrl Pts',(1.95399561553263,9.76566134216263,12.6769470895467));
#89866=CARTESIAN_POINT('Ctrl Pts',(-2.91685788948089,9.52250914244261,12.7556839028237));
#89867=CARTESIAN_POINT('Ctrl Pts',(-7.08826426962872,6.99590951622696,12.8344207161006));
#89868=CARTESIAN_POINT('Ctrl Pts',(-9.55994229428842,2.79172771688173,12.9131575293776));
#89869=CARTESIAN_POINT('Ctrl Pts',(-9.73919662023581,-2.08189565245661,
12.9918943426546));
#89870=CARTESIAN_POINT('Ctrl Pts',(-7.58304300632705,-6.45629143390576,
13.0706311559316));
#89871=CARTESIAN_POINT('Ctrl Pts',(-3.60851570762686,-9.28250260991829,
13.1493679692085));
#89872=CARTESIAN_POINT('Ctrl Pts',(1.23131460972035,-9.88281865902736,13.2281047824855));
#89873=CARTESIAN_POINT('Ctrl Pts',(5.77588218331859,-8.1132869615066,13.3068415957625));
#89874=CARTESIAN_POINT('Ctrl Pts',(8.93542369813816,-4.39823187770733,13.3855784090395));
#89875=CARTESIAN_POINT('Ctrl Pts',(9.95229777699576,0.371495993699875,13.4643152223164));
#89876=CARTESIAN_POINT('Ctrl Pts',(8.58266338348975,5.05214108681008,13.5430520355934));
#89877=CARTESIAN_POINT('Ctrl Pts',(5.15495161538101,8.5213094157184,13.6217888488704));
#89878=CARTESIAN_POINT('Ctrl Pts',(0.491109661018408,9.94711272763029,13.7005256621473));
#89879=CARTESIAN_POINT('Ctrl Pts',(-4.2904977976671,8.98765091464637,13.7792624754243));
#89880=CARTESIAN_POINT('Ctrl Pts',(-8.04326653244926,5.87299785487033,13.8579992887013));
#89881=CARTESIAN_POINT('Ctrl Pts',(-9.86730241022852,1.35003091091588,13.9367361019783));
#89882=CARTESIAN_POINT('Ctrl Pts',(-9.32521125593535,-3.49666631915414,
14.0154729152552));
#89883=CARTESIAN_POINT('Ctrl Pts',(-6.54698366686712,-7.50488142352065,
14.0942097285322));
#89884=CARTESIAN_POINT('Ctrl Pts',(-2.19882395362953,-9.71346557806612,
14.1729465418092));
#89885=CARTESIAN_POINT('Ctrl Pts',(2.67660213689652,-9.59281196084291,14.2516833550862));
#89886=CARTESIAN_POINT('Ctrl Pts',(6.9101931638039,-7.17185267237469,14.3304201683631));
#89887=CARTESIAN_POINT('Ctrl Pts',(9.48675634642733,-3.0311209706726,14.4091569816401));
#89888=CARTESIAN_POINT('Ctrl Pts',(9.78844543431353,1.83645753961172,14.4878937949171));
#89889=CARTESIAN_POINT('Ctrl Pts',(7.74291697669439,6.26366322588849,14.566630608194));
#89890=CARTESIAN_POINT('Ctrl Pts',(3.84067790010628,9.18887553419707,14.645367421471));
#89891=CARTESIAN_POINT('Ctrl Pts',(-0.98253546338574,9.91064399413679,14.724104234748));
#89892=CARTESIAN_POINT('Ctrl Pts',(-5.57014200920517,8.25589233896724,14.802841048025));
#89893=CARTESIAN_POINT('Ctrl Pts',(-8.82205790397076,4.62142128076604,14.8815778613019));
#89894=CARTESIAN_POINT('Ctrl Pts',(-9.95849088179891,-0.121242205760894,
14.9603146745789));
#89895=CARTESIAN_POINT('Ctrl Pts',(-8.70693031342283,-4.83483245133989,
15.0390514878559));
#89896=CARTESIAN_POINT('Ctrl Pts',(-5.36749381660599,-8.38905539640943,
15.1177883011329));
#89897=CARTESIAN_POINT('Ctrl Pts',(-0.740960635614568,-9.93162714019209,
15.1965251144098));
#89898=CARTESIAN_POINT('Ctrl Pts',(4.06325099453557,-9.09264712120377,15.2752619276868));
#89899=CARTESIAN_POINT('Ctrl Pts',(7.89311648462012,-6.07329831932775,15.3539987409638));
#89900=CARTESIAN_POINT('Ctrl Pts',(9.83025430658368,-1.59760463920927,15.4327355542408));
#89901=CARTESIAN_POINT('Ctrl Pts',(9.41014903616523,3.26118620021702,15.5114723675177));
#89902=CARTESIAN_POINT('Ctrl Pts',(6.73353969962842,7.33796180344845,15.5902091807947));
#89903=CARTESIAN_POINT('Ctrl Pts',(2.44226308702735,9.65513290064143,15.6689459940717));
#89904=CARTESIAN_POINT('Ctrl Pts',(-2.43465532202399,9.65705409420066,15.7476828073487));
#89905=CARTESIAN_POINT('Ctrl Pts',(-6.72775623651459,7.34326469203596,15.8264196206256));
#89906=CARTESIAN_POINT('Ctrl Pts',(-9.40757671886562,3.26859917916485,15.9051564339026));
#89907=CARTESIAN_POINT('Ctrl Pts',(-9.83150996321104,-1.5898591631637,15.9838932471796));
#89908=CARTESIAN_POINT('Ctrl Pts',(-7.89789901533805,-6.06707767037656,
16.0626300604565));
#89909=CARTESIAN_POINT('Ctrl Pts',(-4.07041357373357,-9.0894429782792,16.1413668737335));
#89910=CARTESIAN_POINT('Ctrl Pts',(0.733135556639757,-9.93220783956288,
16.2201036870105));
#89911=CARTESIAN_POINT('Ctrl Pts',(5.36088265044753,-8.39328168999638,16.2988405002875));
#89912=CARTESIAN_POINT('Ctrl Pts',(8.70311838290376,-4.84169089515441,16.3775773135644));
#89913=CARTESIAN_POINT('Ctrl Pts',(9.95839226758806,-0.129088183305203,
16.4563141268414));
#89914=CARTESIAN_POINT('Ctrl Pts',(8.82569625352232,4.61446919761579,16.5350509401184));
#89915=CARTESIAN_POINT('Ctrl Pts',(5.57664486494524,8.25150121504901,16.6137877533954));
#89916=CARTESIAN_POINT('Ctrl Pts',(0.990343475914901,9.90986681331834,16.6925245666723));
#89917=CARTESIAN_POINT('Ctrl Pts',(-3.83343705307411,9.1918986301984,16.7712613799493));
#89918=CARTESIAN_POINT('Ctrl Pts',(-7.73797960798613,6.26976173472755,16.8499981932263));
#89919=CARTESIAN_POINT('Ctrl Pts',(-9.7869955067798,1.84416895758031,16.9287350065032));
#89920=CARTESIAN_POINT('Ctrl Pts',(-9.4891415297134,-3.02364558069367,17.0074718197802));
#89921=CARTESIAN_POINT('Ctrl Pts',(-6.9158415332832,-7.16640629673887,17.0862086330572));
#89922=CARTESIAN_POINT('Ctrl Pts',(-2.68415918568418,-9.59069978252784,
17.1649454463342));
#89923=CARTESIAN_POINT('Ctrl Pts',(2.19117025397864,-9.71519569521335,17.2436822596111));
#89924=CARTESIAN_POINT('Ctrl Pts',(6.54106885038804,-7.51003584110843,17.3224190728881));
#89925=CARTESIAN_POINT('Ctrl Pts',(9.32245324281387,-3.50401509328376,17.4011558861651));
#89926=CARTESIAN_POINT('Ctrl Pts',(9.86836337551943,1.34226173323373,17.479892699442));
#89927=CARTESIAN_POINT('Ctrl Pts',(8.04789047483866,5.86664846985783,17.5586295127191));
#89928=CARTESIAN_POINT('Ctrl Pts',(4.29757900067065,8.98428813672743,17.637366325996));
#89929=CARTESIAN_POINT('Ctrl Pts',(-0.483275211443491,9.94745703283269,
17.716103139273));
#89930=CARTESIAN_POINT('Ctrl Pts',(-5.14823096320779,8.52544497969089,17.7948399525499));
#89931=CARTESIAN_POINT('Ctrl Pts',(-8.57869078366569,5.05875215144844,17.873576765827));
#89932=CARTESIAN_POINT('Ctrl Pts',(-9.95198044597383,0.379631352887077,
17.9523135791039));
#89933=CARTESIAN_POINT('Ctrl Pts',(-8.93886491421426,-4.39215829551661,
18.0310562052408));
#89934=CARTESIAN_POINT('Ctrl Pts',(-6.83388360821196,-6.86921757158827,
18.0835532269521));
#89935=CARTESIAN_POINT('Ctrl Pts',(-5.54986593758053,-7.78462397345723,
18.1098046442377));
#89936=CARTESIAN_POINT('Ctrl Pts',(-4.22448130246814,8.78895683937523,3.89002224404915));
#89937=CARTESIAN_POINT('Ctrl Pts',(-5.67383298479217,8.09231454216333,3.91626784847481));
#89938=CARTESIAN_POINT('Ctrl Pts',(-8.21994906199031,5.96910867223154,3.96875905732613));
#89939=CARTESIAN_POINT('Ctrl Pts',(-10.0682113125008,1.34985485719344,4.0474958706031));
#89940=CARTESIAN_POINT('Ctrl Pts',(-9.50204891409078,-3.59177981963027,
4.12623268388007));
#89941=CARTESIAN_POINT('Ctrl Pts',(-6.65741003953953,-7.67276984229252,
4.20496949715705));
#89942=CARTESIAN_POINT('Ctrl Pts',(-2.21632579141437,-9.91354050723984,
4.28370631043402));
#89943=CARTESIAN_POINT('Ctrl Pts',(2.75620434820641,-9.77726608838962,4.362443123711));
#89944=CARTESIAN_POINT('Ctrl Pts',(7.06782016959352,-7.29636749845425,4.44117993698797));
#89945=CARTESIAN_POINT('Ctrl Pts',(9.68460541769376,-3.06588352181864,4.51991675026494));
#89946=CARTESIAN_POINT('Ctrl Pts',(9.97907578135268,1.89980634244646,4.59865356354192));
#89947=CARTESIAN_POINT('Ctrl Pts',(7.88061522553522,6.40992071683142,4.67739037681889));
#89948=CARTESIAN_POINT('Ctrl Pts',(3.89242536780961,9.3829761010854,4.75612719009586));
#89949=CARTESIAN_POINT('Ctrl Pts',(-1.02914787122592,10.1060401700131,4.83486400337284));
#89950=CARTESIAN_POINT('Ctrl Pts',(-5.703936715852,8.40573078880492,4.9136008166498));
#89951=CARTESIAN_POINT('Ctrl Pts',(-9.01095173128544,4.68977069186698,4.99233762992679));
#89952=CARTESIAN_POINT('Ctrl Pts',(-10.157188042639,-0.150771226762893,
5.07107444320375));
#89953=CARTESIAN_POINT('Ctrl Pts',(-8.86778430037797,-4.95515922506173,
5.14981125648073));
#89954=CARTESIAN_POINT('Ctrl Pts',(-5.45193268088805,-8.57132608224742,
5.2285480697577));
#89955=CARTESIAN_POINT('Ctrl Pts',(-0.728736389374847,-10.1321342493071,
5.30728488303467));
#89956=CARTESIAN_POINT('Ctrl Pts',(4.16920704471151,-9.26331007657935,5.38602169631165));
#89957=CARTESIAN_POINT('Ctrl Pts',(8.06739663558773,-6.1731930609301,5.46475850958863));
#89958=CARTESIAN_POINT('Ctrl Pts',(10.0310670989351,-1.60277692716936,5.54349532286559));
#89959=CARTESIAN_POINT('Ctrl Pts',(9.58934062188332,3.35197664905467,5.62223213614258));
#89960=CARTESIAN_POINT('Ctrl Pts',(6.84814088256617,7.50294392086303,5.70096894941953));
#89961=CARTESIAN_POINT('Ctrl Pts',(2.46479310834046,9.85474484464604,5.77970576269653));
#89962=CARTESIAN_POINT('Ctrl Pts',(-2.50959904246025,9.84342997487063,5.85844257597348));
#89963=CARTESIAN_POINT('Ctrl Pts',(-6.8822025901698,7.47171255671175,5.93717938925047));
#89964=CARTESIAN_POINT('Ctrl Pts',(-9.60449028538516,3.30831790805872,6.01591620252743));
#89965=CARTESIAN_POINT('Ctrl Pts',(-10.0236719087839,-1.64839391161847,
6.09465301580442));
#89966=CARTESIAN_POINT('Ctrl Pts',(-8.03922991977018,-6.20982957252095,
6.17338982908138));
#89967=CARTESIAN_POINT('Ctrl Pts',(-4.12702303216825,-9.28218088138534,
6.25212664235836));
#89968=CARTESIAN_POINT('Ctrl Pts',(0.774822193495284,-10.1287142121394,
6.33086345563533));
#89969=CARTESIAN_POINT('Ctrl Pts',(5.49086914716262,-8.54643534062606,6.40960026891231));
#89970=CARTESIAN_POINT('Ctrl Pts',(8.89023466364162,-4.91476638795123,6.48833708218927));
#89971=CARTESIAN_POINT('Ctrl Pts',(10.1577688360944,-0.104562398711278,
6.56707389546626));
#89972=CARTESIAN_POINT('Ctrl Pts',(8.98952366081856,4.73071510179355,6.64581070874322));
#89973=CARTESIAN_POINT('Ctrl Pts',(5.66563816410407,8.43159209261217,6.7245475220202));
#89974=CARTESIAN_POINT('Ctrl Pts',(0.983162542480492,10.1106178069303,6.80328433529717));
#89975=CARTESIAN_POINT('Ctrl Pts',(-3.93507026707246,9.36517074142033,6.88202114857415));
#89976=CARTESIAN_POINT('Ctrl Pts',(-7.90969399838605,6.37400516744763,6.96075796185111));
#89977=CARTESIAN_POINT('Ctrl Pts',(-9.98761486128421,1.85438680037579,7.0394947751281));
#89978=CARTESIAN_POINT('Ctrl Pts',(-9.67055840143241,-3.10990373279276,
7.11823158840506));
#89979=CARTESIAN_POINT('Ctrl Pts',(-7.03455308427736,-7.32845576688822,
7.19696840168204));
#89980=CARTESIAN_POINT('Ctrl Pts',(-2.71169907035961,-9.78968279233623,
7.275705214959));
#89981=CARTESIAN_POINT('Ctrl Pts',(2.26140606655735,-9.90339556035661,7.35444202823599));
#89982=CARTESIAN_POINT('Ctrl Pts',(6.6922379658539,-7.64232634942638,7.43317884151296));
#89983=CARTESIAN_POINT('Ctrl Pts',(9.51830652682872,-3.54866762096472,7.51191565478993));
#89984=CARTESIAN_POINT('Ctrl Pts',(10.061935426348,1.39594287087871,7.59065246806691));
#89985=CARTESIAN_POINT('Ctrl Pts',(8.1927653239262,6.00581363096009,7.66938928134388));
#89986=CARTESIAN_POINT('Ctrl Pts',(4.35901334345506,9.17552198484281,7.74812609462085));
#89987=CARTESIAN_POINT('Ctrl Pts',(-0.520007027130731,10.1449886010034,
7.82686290789783));
#89988=CARTESIAN_POINT('Ctrl Pts',(-5.2743324575385,8.68174050234795,7.9055997211748));
#89989=CARTESIAN_POINT('Ctrl Pts',(-8.7639008059111,5.13665685897979,7.98433653445178));
#89990=CARTESIAN_POINT('Ctrl Pts',(-10.1519320024708,0.359830015371412,
8.06307334772874));
#89991=CARTESIAN_POINT('Ctrl Pts',(-9.10558349319444,-4.50328216651126,
8.14181016100572));
#89992=CARTESIAN_POINT('Ctrl Pts',(-5.87576412731326,-8.28653105605306,
8.2205469742827));
#89993=CARTESIAN_POINT('Ctrl Pts',(-1.23696753972395,-10.0827135399367,
8.29928378755967));
#89994=CARTESIAN_POINT('Ctrl Pts',(3.69844733438944,-9.46111453992081,8.37802060083665));
#89995=CARTESIAN_POINT('Ctrl Pts',(7.74699406047446,-6.57079021501422,8.45675741411361));
#89996=CARTESIAN_POINT('Ctrl Pts',(9.93785250442149,-2.10482508135873,8.53549422739059));
#89997=CARTESIAN_POINT('Ctrl Pts',(9.74566637611686,2.86586599620061,8.61423104066756));
#89998=CARTESIAN_POINT('Ctrl Pts',(7.21652089464729,7.1493375357352,8.69296785394453));
#89999=CARTESIAN_POINT('Ctrl Pts',(2.95689179603023,9.71843567295284,8.77170466722151));
#90000=CARTESIAN_POINT('Ctrl Pts',(-2.01178434691864,9.95710423588336,8.85044148049848));
#90001=CARTESIAN_POINT('Ctrl Pts',(-6.49804522295423,7.80811176298054,8.92917829377545));
#90002=CARTESIAN_POINT('Ctrl Pts',(-9.42610915534255,3.78677530549685,9.00791510705244));
#90003=CARTESIAN_POINT('Ctrl Pts',(-10.0938418692813,-1.14260988123551,
9.08665192032941));
#90004=CARTESIAN_POINT('Ctrl Pts',(-8.34112458468613,-5.79800324986954,
9.16538873360637));
#90005=CARTESIAN_POINT('Ctrl Pts',(-4.58824965444592,-9.06306604473511,
9.24412554688336));
#90006=CARTESIAN_POINT('Ctrl Pts',(0.264863323229445,-10.1548534427022,
9.32286236016032));
#90007=CARTESIAN_POINT('Ctrl Pts',(5.05446347411148,-8.81156058888697,9.4015991734373));
#90008=CARTESIAN_POINT('Ctrl Pts',(8.6320299645758,-5.35530201887989,9.48033598671427));
#90009=CARTESIAN_POINT('Ctrl Pts',(10.1396812348812,-0.614870293436814,
9.55907279999125));
#90010=CARTESIAN_POINT('Ctrl Pts',(9.21589046875117,4.27300408269577,9.63780961326821));
#90011=CARTESIAN_POINT('Ctrl Pts',(6.0821778155482,8.13623463543219,9.71654642654519));
#90012=CARTESIAN_POINT('Ctrl Pts',(1.48999102778118,10.0484390708152,9.79528323982216));
#90013=CARTESIAN_POINT('Ctrl Pts',(-3.45948774332716,9.55108085907153,9.87402005309914));
#90014=CARTESIAN_POINT('Ctrl Pts',(-7.57939961496306,6.76342387400428,9.95275686637611));
#90015=CARTESIAN_POINT('Ctrl Pts',(-9.88181146782447,2.35393354560535,10.0314936796531));
#90016=CARTESIAN_POINT('Ctrl Pts',(-9.81461709318993,-2.62001762147078,
10.11023049293));
#90017=CARTESIAN_POINT('Ctrl Pts',(-7.39392934740214,-6.96570239303823,
10.188967306207));
#90018=CARTESIAN_POINT('Ctrl Pts',(-3.2002163739709,-9.64104850016438,10.267704119484));
#90019=CARTESIAN_POINT('Ctrl Pts',(1.76089159316035,-10.0045220685393,10.346440932761));
#90020=CARTESIAN_POINT('Ctrl Pts',(6.299747051358,-7.96896405511154,10.4251777460379));
#90021=CARTESIAN_POINT('Ctrl Pts',(9.32795642071318,-4.02249052653063,10.5039145593149));
#90022=CARTESIAN_POINT('Ctrl Pts',(10.1193710792704,0.888554997047943,10.5826513725919));
#90023=CARTESIAN_POINT('Ctrl Pts',(8.48421396949771,5.58652972269309,10.6613881858689));
#90024=CARTESIAN_POINT('Ctrl Pts',(4.81458713491896,8.94488411009478,10.7401249991458));
#90025=CARTESIAN_POINT('Ctrl Pts',(-0.00955228015910545,10.1583025046853,
10.8188618124228));
#90026=CARTESIAN_POINT('Ctrl Pts',(-4.83140110887802,8.93581358063637,10.8975986256998));
#90027=CARTESIAN_POINT('Ctrl Pts',(-8.49470545489712,5.57056372886038,10.9763354389768));
#90028=CARTESIAN_POINT('Ctrl Pts',(-10.1210242732921,0.869522099883329,
11.0550722522537));
#90029=CARTESIAN_POINT('Ctrl Pts',(-9.32037489615738,-4.04002633875481,
11.1338090655307));
#90030=CARTESIAN_POINT('Ctrl Pts',(-6.28474881779303,-7.98079778718909,
11.2125458788077));
#90031=CARTESIAN_POINT('Ctrl Pts',(-1.74207314782492,-10.007816053984,11.2912826920847));
#90032=CARTESIAN_POINT('Ctrl Pts',(3.21834246722113,-9.63501285865432,11.3700195053616));
#90033=CARTESIAN_POINT('Ctrl Pts',(7.40701654708679,-6.95178443954758,11.4487563186386));
#90034=CARTESIAN_POINT('Ctrl Pts',(9.81952715790716,-2.60155480777876,11.5274931319156));
#90035=CARTESIAN_POINT('Ctrl Pts',(9.87736698997358,2.37251393423389,11.6062299451925));
#90036=CARTESIAN_POINT('Ctrl Pts',(7.56666635687184,6.77766635845533,11.6849667584695));
#90037=CARTESIAN_POINT('Ctrl Pts',(3.44151907307169,9.55757016675457,11.7637035717465));
#90038=CARTESIAN_POINT('Ctrl Pts',(-1.50888631792369,10.0456191000026,11.8424403850235));
#90039=CARTESIAN_POINT('Ctrl Pts',(-6.09746873474301,8.12478160023917,11.9211771983004));
#90040=CARTESIAN_POINT('Ctrl Pts',(-9.22391033529052,4.25566436050519,11.9999140115774));
#90041=CARTESIAN_POINT('Ctrl Pts',(-10.138506927103,-0.633938728773694,
12.0786508248544));
#90042=CARTESIAN_POINT('Ctrl Pts',(-8.62194307528639,-5.37152665722461,
12.1573876381314));
#90043=CARTESIAN_POINT('Ctrl Pts',(-5.03788278611751,-8.82105084760849,
12.2361244514083));
#90044=CARTESIAN_POINT('Ctrl Pts',(-0.245764797988416,-10.1553336078547,
12.3148612646853));
#90045=CARTESIAN_POINT('Ctrl Pts',(4.60528629139531,-9.05442097524958,12.3935980779623));
#90046=CARTESIAN_POINT('Ctrl Pts',(8.35201403773365,-5.78230598777455,12.4723348912392));
#90047=CARTESIAN_POINT('Ctrl Pts',(10.0959729050677,-1.12362454712121,12.5510717045162));
#90048=CARTESIAN_POINT('Ctrl Pts',(9.41897076273508,3.80449612872647,12.6298085177932));
#90049=CARTESIAN_POINT('Ctrl Pts',(6.48334915081932,7.82031871545681,12.7085453310702));
#90050=CARTESIAN_POINT('Ctrl Pts',(1.99305463577895,9.96087015483855,12.7872821443471));
#90051=CARTESIAN_POINT('Ctrl Pts',(-2.97516386031069,9.7128575109004,12.8660189576241));
#90052=CARTESIAN_POINT('Ctrl Pts',(-7.22995376750567,7.13575290649022,12.9447557709011));
#90053=CARTESIAN_POINT('Ctrl Pts',(-9.75103892554896,2.84753242214774,13.0234925841781));
#90054=CARTESIAN_POINT('Ctrl Pts',(-9.93387642143324,-2.12351130593791,
13.102229397455));
#90055=CARTESIAN_POINT('Ctrl Pts',(-7.73462278877812,-6.58534823210344,
13.180966210732));
#90056=CARTESIAN_POINT('Ctrl Pts',(-3.68064743963431,-9.46805341386847,
13.259703024009));
#90057=CARTESIAN_POINT('Ctrl Pts',(1.25592773673471,-10.0803693653979,13.338439837286));
#90058=CARTESIAN_POINT('Ctrl Pts',(5.89133807142048,-8.2754659537083,13.4171766505629));
#90059=CARTESIAN_POINT('Ctrl Pts',(9.11403663481036,-4.48614948949405,13.4959134638399));
#90060=CARTESIAN_POINT('Ctrl Pts',(10.1512373228571,0.378921941549486,13.5746502771169));
#90061=CARTESIAN_POINT('Ctrl Pts',(8.75422488557203,5.15312989120056,13.6533870903938));
#90062=CARTESIAN_POINT('Ctrl Pts',(5.25799553109575,8.69164449444008,13.7321239036708));
#90063=CARTESIAN_POINT('Ctrl Pts',(0.500926603308566,10.1459486279426,13.8108607169478));
#90064=CARTESIAN_POINT('Ctrl Pts',(-4.37626187974265,9.16730783723688,13.8895975302248));
#90065=CARTESIAN_POINT('Ctrl Pts',(-8.20404586472617,5.99039501804534,13.9683343435018));
#90066=CARTESIAN_POINT('Ctrl Pts',(-10.0645429575225,1.37701709464294,14.0470711567787));
#90067=CARTESIAN_POINT('Ctrl Pts',(-9.51161577616627,-3.56656225928252,
14.1258079700557));
#90068=CARTESIAN_POINT('Ctrl Pts',(-6.67785334004534,-7.65489881001693,
14.2045447833327));
#90069=CARTESIAN_POINT('Ctrl Pts',(-2.24277692294032,-9.90763103353571,
14.2832815966096));
#90070=CARTESIAN_POINT('Ctrl Pts',(2.73010556148216,-9.78456563399303,14.3620184098866));
#90071=CARTESIAN_POINT('Ctrl Pts',(7.04832314349544,-7.3152130445818,14.4407552231636));
#90072=CARTESIAN_POINT('Ctrl Pts',(9.67639004123265,-3.09171098142872,14.5194920364405));
#90073=CARTESIAN_POINT('Ctrl Pts',(9.98410968522563,1.87316705505327,14.5982288497175));
#90074=CARTESIAN_POINT('Ctrl Pts',(7.89769252918495,6.38886951950104,14.6769656629945));
#90075=CARTESIAN_POINT('Ctrl Pts',(3.91745039369191,9.37255479769078,14.7557024762715));
#90076=CARTESIAN_POINT('Ctrl Pts',(-1.00217566741281,10.1087509097019,14.8344392895485));
#90077=CARTESIAN_POINT('Ctrl Pts',(-5.68148529359275,8.4209219139856,14.9131761028254));
#90078=CARTESIAN_POINT('Ctrl Pts',(-8.99840473686339,4.71380029427931,14.9919129161024));
#90079=CARTESIAN_POINT('Ctrl Pts',(-10.1575542235398,-0.123665753557948,
15.0706497293794));
#90080=CARTESIAN_POINT('Ctrl Pts',(-8.88097582544536,-4.93147740647859,
15.1493865426563));
#90081=CARTESIAN_POINT('Ctrl Pts',(-5.47478630385019,-8.55674680880107,
15.2281233559333));
#90082=CARTESIAN_POINT('Ctrl Pts',(-0.755771925997289,-10.1301534943271,
15.3068601692103));
#90083=CARTESIAN_POINT('Ctrl Pts',(4.1444725702647,-9.27440284530902,15.3855969824873));
#90084=CARTESIAN_POINT('Ctrl Pts',(8.05089442134039,-6.19469935018516,15.4643337957642));
#90085=CARTESIAN_POINT('Ctrl Pts',(10.0267542879219,-1.62953965045109,15.5430706090412));
#90086=CARTESIAN_POINT('Ctrl Pts',(9.59825140384847,3.32637505571324,15.6218074223182));
#90087=CARTESIAN_POINT('Ctrl Pts',(6.86813849881018,7.48464258224303,15.7005442355952));
#90088=CARTESIAN_POINT('Ctrl Pts',(2.49108223616196,9.84813232625381,15.7792810488721));
#90089=CARTESIAN_POINT('Ctrl Pts',(-2.4833223972005,9.8500919231429,15.8580178621491));
#90090=CARTESIAN_POINT('Ctrl Pts',(-6.86223942827068,7.49005147190398,15.9367546754261));
#90091=CARTESIAN_POINT('Ctrl Pts',(-9.59562766770601,3.33393621498071,16.0154914887031));
#90092=CARTESIAN_POINT('Ctrl Pts',(-10.0280350442564,-1.62163934769899,
16.09422830198));
#90093=CARTESIAN_POINT('Ctrl Pts',(-8.05577255153804,-6.18835435476593,
16.172965115257));
#90094=CARTESIAN_POINT('Ctrl Pts',(-4.15177832446459,-9.27113465378456,
16.251701928534));
#90095=CARTESIAN_POINT('Ctrl Pts',(0.747790429108468,-10.1307458014765,
16.3304387418109));
#90096=CARTESIAN_POINT('Ctrl Pts',(5.46804298505493,-8.56105758307237,16.4091755550879));
#90097=CARTESIAN_POINT('Ctrl Pts',(8.87708769707297,-4.93847294583914,16.4879123683649));
#90098=CARTESIAN_POINT('Ctrl Pts',(10.1574536380991,-0.131668566764218,
16.5666491816419));
#90099=CARTESIAN_POINT('Ctrl Pts',(9.00211581450489,4.70670924379752,16.6453859949188));
#90100=CARTESIAN_POINT('Ctrl Pts',(5.68811813691929,8.41644301453876,16.7241228081958));
#90101=CARTESIAN_POINT('Ctrl Pts',(1.01013975670955,10.1079581935767,16.8028596214728));
#90102=CARTESIAN_POINT('Ctrl Pts',(-3.91006480713798,9.37563832328931,16.8815964347498));
#90103=CARTESIAN_POINT('Ctrl Pts',(-7.8926564658927,6.39508993331182,16.9603332480267));
#90104=CARTESIAN_POINT('Ctrl Pts',(-9.98263077464382,1.88103261893102,17.0390700613037));
#90105=CARTESIAN_POINT('Ctrl Pts',(-9.67882290268214,-3.08408616357684,
17.1178068745807));
#90106=CARTESIAN_POINT('Ctrl Pts',(-7.05408441997216,-7.30965779966574,
17.1965436878577));
#90107=CARTESIAN_POINT('Ctrl Pts',(-2.73781367044585,-9.78241123469498,
17.2752805011346));
#90108=CARTESIAN_POINT('Ctrl Pts',(2.2349702311295,-9.90939573452754,17.3540173144116));
#90109=CARTESIAN_POINT('Ctrl Pts',(6.6718202904777,-7.66015626084561,17.4327541276886));
#90110=CARTESIAN_POINT('Ctrl Pts',(9.50880263227094,-3.57405793032188,17.5114909409656));
#90111=CARTESIAN_POINT('Ctrl Pts',(10.0656251307754,1.36909261647494,17.5902277542425));
#90112=CARTESIAN_POINT('Ctrl Pts',(8.20876223652433,5.98391871322,17.6689645675195));
#90113=CARTESIAN_POINT('Ctrl Pts',(4.38348463109427,9.16387783971426,17.7477013807964));
#90114=CARTESIAN_POINT('Ctrl Pts',(-0.492935548507827,10.1462998155679,
17.8264381940735));
#90115=CARTESIAN_POINT('Ctrl Pts',(-5.25114053773606,8.6958627254747,17.9051750073504));
#90116=CARTESIAN_POINT('Ctrl Pts',(-8.7501728762264,5.15987310644641,17.9839118206274));
#90117=CARTESIAN_POINT('Ctrl Pts',(-10.1509136486076,0.387219920937437,
18.0626486339044));
#90118=CARTESIAN_POINT('Ctrl Pts',(-9.11754663841461,-4.47995450059806,
18.1413912600413));
#90119=CARTESIAN_POINT('Ctrl Pts',(-6.97048821269124,-7.00652847754534,
18.1938882817526));
#90120=CARTESIAN_POINT('Ctrl Pts',(-5.66080391732681,-7.94023321995303,
18.2201396990381));
#90121=CARTESIAN_POINT('Ctrl Pts',(-4.30727085462648,8.96119900322285,4.00035729884965));
#90122=CARTESIAN_POINT('Ctrl Pts',(-5.78502630255113,8.25090421244517,4.02660290327531));
#90123=CARTESIAN_POINT('Ctrl Pts',(-8.38104005822907,6.08608867483443,4.07909411212662));
#90124=CARTESIAN_POINT('Ctrl Pts',(-10.2655237506244,1.37630872717284,4.1578309254036));
#90125=CARTESIAN_POINT('Ctrl Pts',(-9.68826594710846,-3.662169962568,4.23656773868056));
#90126=CARTESIAN_POINT('Ctrl Pts',(-6.7878790737819,-7.82313745752762,4.31530455195755));
#90127=CARTESIAN_POINT('Ctrl Pts',(-2.25976038292293,-10.1078217740118,
4.39404136523451));
#90128=CARTESIAN_POINT('Ctrl Pts',(2.8102192454937,-9.96887670821123,4.47277817851149));
#90129=CARTESIAN_POINT('Ctrl Pts',(7.20633224354552,-7.43935854382279,4.55151499178846));
#90130=CARTESIAN_POINT('Ctrl Pts',(9.87440011388349,-3.12596737722422,4.63025180506544));
#90131=CARTESIAN_POINT('Ctrl Pts',(10.1746413800002,1.93703792308732,4.70898861834241));
#90132=CARTESIAN_POINT('Ctrl Pts',(8.03505610443629,6.5355395626781,4.78772543161938));
#90133=CARTESIAN_POINT('Ctrl Pts',(3.96870743179283,9.56685959676272,4.86646224489636));
#90134=CARTESIAN_POINT('Ctrl Pts',(-1.04931666480389,10.3040939616776,4.94519905817333));
#90135=CARTESIAN_POINT('Ctrl Pts',(-5.8157199934745,8.57046265474128,5.0239358714503));
#90136=CARTESIAN_POINT('Ctrl Pts',(-9.18754445473239,4.78167878365525,5.10267268472728));
#90137=CARTESIAN_POINT('Ctrl Pts',(-10.3562442081254,-0.15372597586658,
5.18140949800426));
#90138=CARTESIAN_POINT('Ctrl Pts',(-9.04157129061419,-5.0522682862088,5.26014631128122));
#90139=CARTESIAN_POINT('Ctrl Pts',(-5.5587772927424,-8.73930321291617,5.3388831245582));
#90140=CARTESIAN_POINT('Ctrl Pts',(-0.74301784903776,-10.330699421419,5.41761993783518));
#90141=CARTESIAN_POINT('Ctrl Pts',(4.25091335594205,-9.44484840941464,5.49635675111214));
#90142=CARTESIAN_POINT('Ctrl Pts',(8.22549797554484,-6.29417262085923,5.57509356438912));
#90143=CARTESIAN_POINT('Ctrl Pts',(10.2276516008729,-1.63418745416888,5.65383037766609));
#90144=CARTESIAN_POINT('Ctrl Pts',(9.77726835992674,3.41766723347228,5.73256719094306));
#90145=CARTESIAN_POINT('Ctrl Pts',(6.98234777713893,7.64998336135349,5.81130400422005));
#90146=CARTESIAN_POINT('Ctrl Pts',(2.51309705455117,10.0478738595257,5.89004081749701));
#90147=CARTESIAN_POINT('Ctrl Pts',(-2.55878107593283,10.0363372458403,5.96877763077398));
#90148=CARTESIAN_POINT('Ctrl Pts',(-7.01707701131357,7.6181399384745,6.04751444405097));
#90149=CARTESIAN_POINT('Ctrl Pts',(-9.79271491996257,3.3731528874077,6.12625125732793));
#90150=CARTESIAN_POINT('Ctrl Pts',(-10.2201114829928,-1.68069842049241,
6.20498807060491));
#90151=CARTESIAN_POINT('Ctrl Pts',(-8.19677926064828,-6.33152711891279,
6.28372488388187));
#90152=CARTESIAN_POINT('Ctrl Pts',(-4.2079026394187,-9.46408903606783,6.36246169715886));
#90153=CARTESIAN_POINT('Ctrl Pts',(0.790006822757178,-10.3272123598464,
6.44119851043582));
#90154=CARTESIAN_POINT('Ctrl Pts',(5.59847681899395,-8.7139246733371,6.51993532371281));
#90155=CARTESIAN_POINT('Ctrl Pts',(9.06446162635903,-5.01108384779742,6.59867213698977));
#90156=CARTESIAN_POINT('Ctrl Pts',(10.3568363837189,-0.106611567246333,
6.67740895026675));
#90157=CARTESIAN_POINT('Ctrl Pts',(9.16569644623514,4.82342560436751,6.75614576354371));
#90158=CARTESIAN_POINT('Ctrl Pts',(5.77667088332179,8.59683077716295,6.8348825768207));
#90159=CARTESIAN_POINT('Ctrl Pts',(1.00243013553229,10.3087613091375,6.91361939009766));
#90160=CARTESIAN_POINT('Ctrl Pts',(-4.0121880672938,9.54870529538218,6.99235620337465));
#90161=CARTESIAN_POINT('Ctrl Pts',(-8.06470475046425,6.4989201559362,7.0710930166516));
#90162=CARTESIAN_POINT('Ctrl Pts',(-10.1833478051164,1.89072826853232,7.14982982992859));
#90163=CARTESIAN_POINT('Ctrl Pts',(-9.86007781029048,-3.1708502771988,7.22856664320556));
#90164=CARTESIAN_POINT('Ctrl Pts',(-7.17241320432127,-7.47207566422293,
7.30730345648254));
#90165=CARTESIAN_POINT('Ctrl Pts',(-2.76484177251623,-9.98153674933592,
7.38604026975951));
#90166=CARTESIAN_POINT('Ctrl Pts',(2.30572412174414,-10.09747801086,7.46477708303648));
#90167=CARTESIAN_POINT('Ctrl Pts',(6.82338954268924,-7.79209734629346,7.54351389631346));
#90168=CARTESIAN_POINT('Ctrl Pts',(9.70484216948892,-3.61821286973333,7.62225070959043));
#90169=CARTESIAN_POINT('Ctrl Pts',(10.2591248723769,1.42329995375918,7.7009875228674));
#90170=CARTESIAN_POINT('Ctrl Pts',(8.35332358505756,6.12351296142299,7.77972433614438));
#90171=CARTESIAN_POINT('Ctrl Pts',(4.44443939619817,9.35533988473514,7.85846114942134));
#90172=CARTESIAN_POINT('Ctrl Pts',(-0.530197899290624,10.3438056871242,
7.93719796269834));
#90173=CARTESIAN_POINT('Ctrl Pts',(-5.37769653725135,8.85188148692859,8.0159347759753));
#90174=CARTESIAN_POINT('Ctrl Pts',(-8.93565193248317,5.23732283203015,8.09467158925227));
#90175=CARTESIAN_POINT('Ctrl Pts',(-10.3508851623618,0.366881807933114,
8.17340840252925));
#90176=CARTESIAN_POINT('Ctrl Pts',(-9.28403076886391,-4.59153553707068,
8.25214521580621));
#90177=CARTESIAN_POINT('Ctrl Pts',(-5.99091480401388,-8.44892689733091,
8.33088202908319));
#90178=CARTESIAN_POINT('Ctrl Pts',(-1.26120909302149,-10.2803101864231,
8.40961884236016));
#90179=CARTESIAN_POINT('Ctrl Pts',(3.77092790101342,-9.64652935882917,8.48835565563714));
#90180=CARTESIAN_POINT('Ctrl Pts',(7.89881628974206,-6.69956171150768,8.56709246891411));
#90181=CARTESIAN_POINT('Ctrl Pts',(10.1326102271687,-2.14607453031608,8.64582928219108));
#90182=CARTESIAN_POINT('Ctrl Pts',(9.93665771848401,2.92202999489853,8.72456609546806));
#90183=CARTESIAN_POINT('Ctrl Pts',(7.35794714090862,7.28944715166994,8.80330290874504));
#90184=CARTESIAN_POINT('Ctrl Pts',(3.01483967886997,9.90889335981096,8.88203972202201));
#90185=CARTESIAN_POINT('Ctrl Pts',(-2.05121042391966,10.1522392457131,8.96077653529897));
#90186=CARTESIAN_POINT('Ctrl Pts',(-6.62539109464709,7.96113175047151,9.03951334857597));
#90187=CARTESIAN_POINT('Ctrl Pts',(-9.61083795390783,3.86098688538555,9.11825016185292));
#90188=CARTESIAN_POINT('Ctrl Pts',(-10.2916566039392,-1.16500225407046,
9.1969869751299));
#90189=CARTESIAN_POINT('Ctrl Pts',(-8.50459032625769,-5.91163000262351,
9.27572378840688));
#90190=CARTESIAN_POINT('Ctrl Pts',(-4.67816818097848,-9.24068008189199,
9.35446060168385));
#90191=CARTESIAN_POINT('Ctrl Pts',(0.270053999751182,-10.3538638557117,
9.43319741496082));
#90192=CARTESIAN_POINT('Ctrl Pts',(5.15351865685732,-8.98424573121294,9.51193422823778));
#90193=CARTESIAN_POINT('Ctrl Pts',(8.80119674359953,-5.46025290493465,9.59067104151478));
#90194=CARTESIAN_POINT('Ctrl Pts',(10.3383943095429,-0.626920254741986,
9.66940785479173));
#90195=CARTESIAN_POINT('Ctrl Pts',(9.39649949268091,4.3567445632538,9.74814466806871));
#90196=CARTESIAN_POINT('Ctrl Pts',(6.20137369817706,8.29568503265116,9.8268814813457));
#90197=CARTESIAN_POINT('Ctrl Pts',(1.51919122564639,10.2453640211226,9.90561829462266));
#90198=CARTESIAN_POINT('Ctrl Pts',(-3.52728528353637,9.7382587988789,9.98435510789964));
#90199=CARTESIAN_POINT('Ctrl Pts',(-7.72793740098316,6.89597052139002,10.0630919211766));
#90200=CARTESIAN_POINT('Ctrl Pts',(-10.0754709226447,2.40006491419192,10.1418287344536));
#90201=CARTESIAN_POINT('Ctrl Pts',(-10.0069597018023,-2.67136359035973,
10.2205655477306));
#90202=CARTESIAN_POINT('Ctrl Pts',(-7.538832367568,-7.10221320709983,10.2993023610076));
#90203=CARTESIAN_POINT('Ctrl Pts',(-3.26293282634487,-9.82998958677756,
10.3780391742845));
#90204=CARTESIAN_POINT('Ctrl Pts',(1.79540078280026,-10.2005863524856,10.4567759875615));
#90205=CARTESIAN_POINT('Ctrl Pts',(6.42320676149755,-8.12513635605253,10.5355128008385));
#90206=CARTESIAN_POINT('Ctrl Pts',(9.51076166455986,-4.10132155107751,10.6142496141155));
#90207=CARTESIAN_POINT('Ctrl Pts',(10.3176861243121,0.905968512461215,10.6929864273924));
#90208=CARTESIAN_POINT('Ctrl Pts',(8.65048391476648,5.69601210899002,10.7717232406694));
#90209=CARTESIAN_POINT('Ctrl Pts',(4.90894132521788,9.12018206895907,10.8504600539464));
#90210=CARTESIAN_POINT('Ctrl Pts',(-0.00973948160225924,10.3573805109155,
10.9291968672234));
#90211=CARTESIAN_POINT('Ctrl Pts',(-4.92608481214535,9.11093377919877,11.0079336805003));
#90212=CARTESIAN_POINT('Ctrl Pts',(-8.66118100774594,5.67973322053559,11.0866704937773));
#90213=CARTESIAN_POINT('Ctrl Pts',(-10.3193717169132,0.886562616833696,
11.1654073070543));
#90214=CARTESIAN_POINT('Ctrl Pts',(-9.50303156057435,-4.11920102254332,
11.2441441203313));
#90215=CARTESIAN_POINT('Ctrl Pts',(-6.40791459905685,-8.13720200047834,
11.3228809336082));
#90216=CARTESIAN_POINT('Ctrl Pts',(-1.77621354173583,-10.2039448920282,
11.4016177468852));
#90217=CARTESIAN_POINT('Ctrl Pts',(3.28141414690822,-9.82383566138324,11.4803545601622));
#90218=CARTESIAN_POINT('Ctrl Pts',(7.55217604451536,-7.08802249559372,11.5590913734392));
#90219=CARTESIAN_POINT('Ctrl Pts',(10.011965991838,-2.65253895045342,11.6378281867161));
#90220=CARTESIAN_POINT('Ctrl Pts',(10.0709393438447,2.41900943321736,11.7165649999931));
#90221=CARTESIAN_POINT('Ctrl Pts',(7.71495460202305,6.91049212387352,11.7953018132701));
#90222=CARTESIAN_POINT('Ctrl Pts',(3.50896447107535,9.74487528119909,11.874038626547));
#90223=CARTESIAN_POINT('Ctrl Pts',(-1.53845681748908,10.2424887857452,11.952775439824));
#90224=CARTESIAN_POINT('Ctrl Pts',(-6.21696428217363,8.28400754584229,12.031512253101));
#90225=CARTESIAN_POINT('Ctrl Pts',(-9.404676529086,4.33906502470902,12.110249066378));
#90226=CARTESIAN_POINT('Ctrl Pts',(-10.3371969881901,-0.646362385003455,
12.188985879655));
#90227=CARTESIAN_POINT('Ctrl Pts',(-8.79091217582913,-5.47679550670405,
12.2677226929319));
#90228=CARTESIAN_POINT('Ctrl Pts',(-5.13661302773209,-8.99392197590836,
12.3464595062089));
#90229=CARTESIAN_POINT('Ctrl Pts',(-0.250581189896677,-10.3543534309325,
12.4251963194859));
#90230=CARTESIAN_POINT('Ctrl Pts',(4.69553869454898,-9.23186559008456,12.5039331327628));
#90231=CARTESIAN_POINT('Ctrl Pts',(8.51569318608262,-5.89562511239483,12.5826699460398));
#90232=CARTESIAN_POINT('Ctrl Pts',(10.2938294028405,-1.14564485361329,12.6614067593168));
#90233=CARTESIAN_POINT('Ctrl Pts',(9.6035596661784,3.87905499362223,12.7401435725938));
#90234=CARTESIAN_POINT('Ctrl Pts',(6.61040701526504,7.97357792950751,12.8188803858707));
#90235=CARTESIAN_POINT('Ctrl Pts',(2.03211365602528,10.1560789675144,12.8976171991477));
#90236=CARTESIAN_POINT('Ctrl Pts',(-3.0334698311405,9.9032058793582,12.9763540124247));
#90237=CARTESIAN_POINT('Ctrl Pts',(-7.37164326538263,7.2755962967535,13.0550908257017));
#90238=CARTESIAN_POINT('Ctrl Pts',(-9.94213555680948,2.90333712741376,13.1338276389786));
#90239=CARTESIAN_POINT('Ctrl Pts',(-10.1285562226306,-2.1651269594192,13.2125644522556));
#90240=CARTESIAN_POINT('Ctrl Pts',(-7.88620257122917,-6.71440503030112,
13.2913012655326));
#90241=CARTESIAN_POINT('Ctrl Pts',(-3.75277917164178,-9.65360421781864,
13.3700380788095));
#90242=CARTESIAN_POINT('Ctrl Pts',(1.28054086374907,-10.2779200717686,13.4487748920865));
#90243=CARTESIAN_POINT('Ctrl Pts',(6.00679395952235,-8.43764494590998,13.5275117053635));
#90244=CARTESIAN_POINT('Ctrl Pts',(9.29264957148258,-4.57406710128077,13.6062485186405));
#90245=CARTESIAN_POINT('Ctrl Pts',(10.3501768687183,0.386347889399096,13.6849853319174));
#90246=CARTESIAN_POINT('Ctrl Pts',(8.92578638765432,5.25411869559104,13.7637221451944));
#90247=CARTESIAN_POINT('Ctrl Pts',(5.3610394468105,8.86197957316176,13.8424589584714));
#90248=CARTESIAN_POINT('Ctrl Pts',(0.51074354559872,10.344784528255,13.9211957717484));
#90249=CARTESIAN_POINT('Ctrl Pts',(-4.46202596181818,9.34696475982737,13.9999325850253));
#90250=CARTESIAN_POINT('Ctrl Pts',(-8.36482519700309,6.10779218122034,14.0786693983023));
#90251=CARTESIAN_POINT('Ctrl Pts',(-10.2617835048164,1.40400327837,14.1574062115793));
#90252=CARTESIAN_POINT('Ctrl Pts',(-9.69802029639719,-3.6364581994109,14.2361430248563));
#90253=CARTESIAN_POINT('Ctrl Pts',(-6.80872301322356,-7.80491619651322,
14.3148798381332));
#90254=CARTESIAN_POINT('Ctrl Pts',(-2.28672989225111,-10.1017964890053,
14.3936166514102));
#90255=CARTESIAN_POINT('Ctrl Pts',(2.78360898606781,-9.97631930714313,14.4723534646872));
#90256=CARTESIAN_POINT('Ctrl Pts',(7.18645312318698,-7.45857341678894,14.5510902779641));
#90257=CARTESIAN_POINT('Ctrl Pts',(9.86602373603799,-3.15230099218483,14.6298270912411));
#90258=CARTESIAN_POINT('Ctrl Pts',(10.1797739361378,1.90987657049483,14.7085639045181));
#90259=CARTESIAN_POINT('Ctrl Pts',(8.05246808167551,6.51407581311359,14.787300717795));
#90260=CARTESIAN_POINT('Ctrl Pts',(3.99422288727754,9.55623406118449,14.8660375310721));
#90261=CARTESIAN_POINT('Ctrl Pts',(-1.02181587143989,10.306857825267,14.944774344349));
#90262=CARTESIAN_POINT('Ctrl Pts',(-5.79282857798032,8.58595148900395,15.023511157626));
#90263=CARTESIAN_POINT('Ctrl Pts',(-9.17475156975602,4.80617930779259,15.102247970903));
#90264=CARTESIAN_POINT('Ctrl Pts',(-10.3566175652806,-0.126089301355015,
15.1809847841799));
#90265=CARTESIAN_POINT('Ctrl Pts',(-9.0550213374679,-5.02812236161728,15.2597215974569));
#90266=CARTESIAN_POINT('Ctrl Pts',(-5.58207879109441,-8.72443822119271,
15.3384584107339));
#90267=CARTESIAN_POINT('Ctrl Pts',(-0.770583216380001,-10.3286798484622,
15.4171952240108));
#90268=CARTESIAN_POINT('Ctrl Pts',(4.22569414599381,-9.45615856941429,15.4959320372878));
#90269=CARTESIAN_POINT('Ctrl Pts',(8.2086723580607,-6.31610038104256,15.5746688505648));
#90270=CARTESIAN_POINT('Ctrl Pts',(10.2232542692602,-1.66147466169291,15.6534056638418));
#90271=CARTESIAN_POINT('Ctrl Pts',(9.78635377153171,3.39156391120948,15.7321424771188));
#90272=CARTESIAN_POINT('Ctrl Pts',(7.00273729799194,7.63132336103759,15.8108792903957));
#90273=CARTESIAN_POINT('Ctrl Pts',(2.53990138529655,10.0411317518662,15.8896161036727));
#90274=CARTESIAN_POINT('Ctrl Pts',(-2.531989472377,10.0431297520852,15.9683529169496));
#90275=CARTESIAN_POINT('Ctrl Pts',(-6.99672262002677,7.63683825177198,16.0470897302267));
#90276=CARTESIAN_POINT('Ctrl Pts',(-9.78367861654637,3.39927325079658,16.1258265435036));
#90277=CARTESIAN_POINT('Ctrl Pts',(-10.2245601253017,-1.65341953223427,
16.2045633567806));
#90278=CARTESIAN_POINT('Ctrl Pts',(-8.21364608773801,-6.30963103915528,
16.2833001700575));
#90279=CARTESIAN_POINT('Ctrl Pts',(-4.23314307519562,-9.45282632928991,
16.3620369833346));
#90280=CARTESIAN_POINT('Ctrl Pts',(0.762445301577178,-10.3292837633901,
16.4407737966115));
#90281=CARTESIAN_POINT('Ctrl Pts',(5.57520331966233,-8.72883347614835,16.5195106098885));
#90282=CARTESIAN_POINT('Ctrl Pts',(9.05105701124216,-5.03525499652388,16.5982474231654));
#90283=CARTESIAN_POINT('Ctrl Pts',(10.3565150086101,-0.134248950223226,
16.6769842364424));
#90284=CARTESIAN_POINT('Ctrl Pts',(9.17853537548744,4.79894928997922,16.7557210497194));
#90285=CARTESIAN_POINT('Ctrl Pts',(5.79959140889334,8.58138481402851,16.8344578629964));
#90286=CARTESIAN_POINT('Ctrl Pts',(1.02993603750419,10.306049573835,16.9131946762733));
#90287=CARTESIAN_POINT('Ctrl Pts',(-3.98669256120186,9.55937801638022,16.9919314895503));
#90288=CARTESIAN_POINT('Ctrl Pts',(-8.0473333237993,6.52041813189609,17.0706683028273));
#90289=CARTESIAN_POINT('Ctrl Pts',(-10.1782660425078,1.91789628028175,17.1494051161043));
#90290=CARTESIAN_POINT('Ctrl Pts',(-9.86850427565091,-3.14452674646001,
17.2281419293812));
#90291=CARTESIAN_POINT('Ctrl Pts',(-7.1923273066611,-7.4529093025926,17.3068787426582));
#90292=CARTESIAN_POINT('Ctrl Pts',(-2.79146815520754,-9.97412268686214,
17.3856155559352));
#90293=CARTESIAN_POINT('Ctrl Pts',(2.27877020828039,-10.1035957738417,17.4643523692122));
#90294=CARTESIAN_POINT('Ctrl Pts',(6.80257173056734,-7.8102766805828,17.5430891824891));
#90295=CARTESIAN_POINT('Ctrl Pts',(9.69515202172803,-3.64410076735999,17.6218259957661));
#90296=CARTESIAN_POINT('Ctrl Pts',(10.2628868860313,1.39592349971614,17.7005628090431));
#90297=CARTESIAN_POINT('Ctrl Pts',(8.36963399820998,6.10118895658217,17.77929962232));
#90298=CARTESIAN_POINT('Ctrl Pts',(4.4693902615179,9.3434675427011,17.858036435597));
#90299=CARTESIAN_POINT('Ctrl Pts',(-0.502595885572172,10.3451425983029,
17.936773248874));
#90300=CARTESIAN_POINT('Ctrl Pts',(-5.35405011226431,8.86628047125853,18.015510062151));
#90301=CARTESIAN_POINT('Ctrl Pts',(-8.92165496878712,5.26099406144437,18.094246875428));
#90302=CARTESIAN_POINT('Ctrl Pts',(-10.3498468512413,0.394808488987801,
18.1729836887049));
#90303=CARTESIAN_POINT('Ctrl Pts',(-9.29622836261498,-4.56775070567949,
18.2517263148418));
#90304=CARTESIAN_POINT('Ctrl Pts',(-7.10709281717051,-7.14383938350242,
18.304223336553));
#90305=CARTESIAN_POINT('Ctrl Pts',(-5.77174189707308,-8.09584246644884,
18.3304747538387));
#90306=CARTESIAN_POINT('Ctrl Pts',(-4.3073013591307,8.9607364793544,18.));
#90307=CARTESIAN_POINT('Ctrl Pts',(-4.52760625432587,8.84750150850078,18.));
#90308=CARTESIAN_POINT('Ctrl Pts',(-4.74323706131295,8.72624255457085,18.));
#90309=CARTESIAN_POINT('Ctrl Pts',(-4.95372227598611,8.59714960774005,18.));
#90310=CARTESIAN_POINT('Ctrl Pts',(-5.01160312760282,8.56165063118779,18.));
#90311=CARTESIAN_POINT('Ctrl Pts',(-5.06909476851584,8.52555897874492,18.));
#90312=CARTESIAN_POINT('Ctrl Pts',(-5.1261871168107,8.48887796796154,18.));
#90313=CARTESIAN_POINT('Ctrl Pts',(-5.33322421369055,8.35585961769175,18.));
#90314=CARTESIAN_POINT('Ctrl Pts',(-5.53501269654285,8.21509436198934,18.));
#90315=CARTESIAN_POINT('Ctrl Pts',(-5.7312285379337,8.06700108805411,18.));
#90316=CARTESIAN_POINT('Ctrl Pts',(-5.92834760164166,7.9182261099859,18.));
#90317=CARTESIAN_POINT('Ctrl Pts',(-6.11984306788491,7.76205502130544,18.));
#90318=CARTESIAN_POINT('Ctrl Pts',(-6.30535299141809,7.59887183662814,18.));
#90319=CARTESIAN_POINT('Ctrl Pts',(-6.49030070142005,7.43618320120592,18.));
#90320=CARTESIAN_POINT('Ctrl Pts',(-6.66929951885765,7.26652439975838,18.));
#90321=CARTESIAN_POINT('Ctrl Pts',(-6.84195102169195,7.09024304306413,18.));
#90322=CARTESIAN_POINT('Ctrl Pts',(-6.99683870006296,6.93209898042791,18.));
#90323=CARTESIAN_POINT('Ctrl Pts',(-7.14661770651649,6.76862435341091,18.));
#90324=CARTESIAN_POINT('Ctrl Pts',(-7.29096872875563,6.60005246861241,18.));
#90325=CARTESIAN_POINT('Ctrl Pts',(-7.31275740699813,6.57460783717417,18.));
#90326=CARTESIAN_POINT('Ctrl Pts',(-7.33441899362598,6.54905088798603,18.));
#90327=CARTESIAN_POINT('Ctrl Pts',(-7.3559421054481,6.523395076923,18.));
#90328=CARTESIAN_POINT('Ctrl Pts',(-7.51382905139519,6.33519191708182,18.));
#90329=CARTESIAN_POINT('Ctrl Pts',(-7.66443332067489,6.14147855738646,18.));
#90330=CARTESIAN_POINT('Ctrl Pts',(-7.80743627194425,5.94265874500182,18.));
#90331=CARTESIAN_POINT('Ctrl Pts',(-7.95018354749679,5.74419440358892,18.));
#90332=CARTESIAN_POINT('Ctrl Pts',(-8.08535707059586,5.54064133904095,18.));
#90333=CARTESIAN_POINT('Ctrl Pts',(-8.2126006506496,5.33236758982748,18.));
#90334=CARTESIAN_POINT('Ctrl Pts',(-8.28587672164632,5.21242847755421,18.));
#90335=CARTESIAN_POINT('Ctrl Pts',(-8.35652223535198,5.09092327046725,18.));
#90336=CARTESIAN_POINT('Ctrl Pts',(-8.42446243614109,4.96791819110294,18.));
#90337=CARTESIAN_POINT('Ctrl Pts',(-8.54281535446282,4.75364137204628,18.));
#90338=CARTESIAN_POINT('Ctrl Pts',(-8.65296146393977,4.53481380518235,18.));
#90339=CARTESIAN_POINT('Ctrl Pts',(-8.75476116990247,4.31194123524967,18.));
#90340=CARTESIAN_POINT('Ctrl Pts',(-8.8562212171741,4.08981228834281,18.));
#90341=CARTESIAN_POINT('Ctrl Pts',(-8.94939060020028,3.86366463572551,18.));
#90342=CARTESIAN_POINT('Ctrl Pts',(-9.03408085695094,3.6339875819897,18.));
#90343=CARTESIAN_POINT('Ctrl Pts',(-9.05818284480564,3.56862382266211,18.));
#90344=CARTESIAN_POINT('Ctrl Pts',(-9.08159777671273,3.50297417480271,18.));
#90345=CARTESIAN_POINT('Ctrl Pts',(-9.10432053672134,3.43704986001775,18.));
#90346=CARTESIAN_POINT('Ctrl Pts',(-9.11838840419275,3.39623551690155,18.));
#90347=CARTESIAN_POINT('Ctrl Pts',(-9.13219095806272,3.35531589487388,18.));
#90348=CARTESIAN_POINT('Ctrl Pts',(-9.14572691705035,3.31429365769524,18.));
#90349=CARTESIAN_POINT('Ctrl Pts',(-9.15617345111333,3.28263426818186,18.));
#90350=CARTESIAN_POINT('Ctrl Pts',(-9.16646082010693,3.25091466828912,18.));
#90351=CARTESIAN_POINT('Ctrl Pts',(-9.17658220167961,3.21915638737006,18.));
#90352=CARTESIAN_POINT('Ctrl Pts',(-9.25054140040622,2.98709152618069,18.));
#90353=CARTESIAN_POINT('Ctrl Pts',(-9.31573488780019,2.75268296772533,18.));
#90354=CARTESIAN_POINT('Ctrl Pts',(-9.37209036933886,2.51644592272189,18.));
#90355=CARTESIAN_POINT('Ctrl Pts',(-9.42853307221032,2.27984325383666,18.));
#90356=CARTESIAN_POINT('Ctrl Pts',(-9.47611053782495,2.04140578250418,18.));
#90357=CARTESIAN_POINT('Ctrl Pts',(-9.51470041111593,1.80163458795178,18.));
#90358=CARTESIAN_POINT('Ctrl Pts',(-9.5529252224677,1.56413163969781,18.));
#90359=CARTESIAN_POINT('Ctrl Pts',(-9.58233174292863,1.32531944671551,18.));
#90360=CARTESIAN_POINT('Ctrl Pts',(-9.60275090844265,1.0856784282915,18.));
#90361=CARTESIAN_POINT('Ctrl Pts',(-9.62309540351779,0.846913748325436,
18.));
#90362=CARTESIAN_POINT('Ctrl Pts',(-9.63451826958938,0.607325689922282,
18.));
#90363=CARTESIAN_POINT('Ctrl Pts',(-9.63680089853934,0.367392081352794,
18.));
#90364=CARTESIAN_POINT('Ctrl Pts',(-9.63858576602893,0.179779592864777,
18.));
#90365=CARTESIAN_POINT('Ctrl Pts',(-9.63478088238045,-0.00804422448828743,
18.));
#90366=CARTESIAN_POINT('Ctrl Pts',(-9.62541795260051,-0.195838307668789,
18.));
#90367=CARTESIAN_POINT('Ctrl Pts',(-9.62262270781222,-0.251903069940943,
18.));
#90368=CARTESIAN_POINT('Ctrl Pts',(-9.61933196404203,-0.307965141664495,
18.));
#90369=CARTESIAN_POINT('Ctrl Pts',(-9.61554626324484,-0.364017993970899,
18.));
#90370=CARTESIAN_POINT('Ctrl Pts',(-9.61250490227994,-0.409049803431933,
18.));
#90371=CARTESIAN_POINT('Ctrl Pts',(-9.60914339172037,-0.454082657053631,
18.));
#90372=CARTESIAN_POINT('Ctrl Pts',(-9.60546607932598,-0.499066988202734,
18.));
#90373=CARTESIAN_POINT('Ctrl Pts',(-9.58595145068401,-0.737788212546353,
18.));
#90374=CARTESIAN_POINT('Ctrl Pts',(-9.55753446716396,-0.975378206055743,
18.));
#90375=CARTESIAN_POINT('Ctrl Pts',(-9.52041083245154,-1.21135394166142,
18.));
#90376=CARTESIAN_POINT('Ctrl Pts',(-9.48257537067788,-1.45185439354827,
18.));
#90377=CARTESIAN_POINT('Ctrl Pts',(-9.43569613673507,-1.69067876605208,
18.));
#90378=CARTESIAN_POINT('Ctrl Pts',(-9.37992571664595,-1.92731195007808,
18.));
#90379=CARTESIAN_POINT('Ctrl Pts',(-9.32477727545944,-2.1613060855209,18.));
#90380=CARTESIAN_POINT('Ctrl Pts',(-9.26093458221553,-2.39315826150895,
18.));
#90381=CARTESIAN_POINT('Ctrl Pts',(-9.18849501396502,-2.62235702764131,
18.));
#90382=CARTESIAN_POINT('Ctrl Pts',(-9.11482995641156,-2.85543324145767,
18.));
#90383=CARTESIAN_POINT('Ctrl Pts',(-9.03227465025842,-3.08576625698368,
18.));
#90384=CARTESIAN_POINT('Ctrl Pts',(-8.94088139600402,-3.31279382281833,
18.));
#90385=CARTESIAN_POINT('Ctrl Pts',(-8.84948814174963,-3.53982138865298,
18.));
#90386=CARTESIAN_POINT('Ctrl Pts',(-8.74925676736514,-3.76354421054282,
18.));
#90387=CARTESIAN_POINT('Ctrl Pts',(-8.64019169798513,-3.98336495971754,
18.));
#90388=CARTESIAN_POINT('Ctrl Pts',(-8.62858600317367,-4.00675624844683,
18.));
#90389=CARTESIAN_POINT('Ctrl Pts',(-8.61688134356907,-4.03010103399861,
18.));
#90390=CARTESIAN_POINT('Ctrl Pts',(-8.60508170405194,-4.0533909536201,18.));
#90391=CARTESIAN_POINT('Ctrl Pts',(-8.58155518124463,-4.0998271879101,18.));
#90392=CARTESIAN_POINT('Ctrl Pts',(-8.5576466944477,-4.14605418913442,18.));
#90393=CARTESIAN_POINT('Ctrl Pts',(-8.53335745420521,-4.19206686624084,
18.));
#90394=CARTESIAN_POINT('Ctrl Pts',(-8.42201512723478,-4.40298982999017,
18.));
#90395=CARTESIAN_POINT('Ctrl Pts',(-8.30267566618238,-4.60941115010306,
18.));
#90396=CARTESIAN_POINT('Ctrl Pts',(-8.17572619796266,-4.81098138527243,
18.));
#90397=CARTESIAN_POINT('Ctrl Pts',(-8.04812742875072,-5.01358257988993,
18.));
#90398=CARTESIAN_POINT('Ctrl Pts',(-7.91284017586144,-5.21128344591977,
18.));
#90399=CARTESIAN_POINT('Ctrl Pts',(-7.77021399871967,-5.40369944292422,
18.));
#90400=CARTESIAN_POINT('Ctrl Pts',(-7.68992477437975,-5.51201708460596,
18.));
#90401=CARTESIAN_POINT('Ctrl Pts',(-7.60730913056893,-5.61865939762238,
18.));
#90402=CARTESIAN_POINT('Ctrl Pts',(-7.52242418953522,-5.72355274841017,
18.));
#90403=CARTESIAN_POINT('Ctrl Pts',(-7.47738280262866,-5.7792109362963,18.));
#90404=CARTESIAN_POINT('Ctrl Pts',(-7.43170242560918,-5.83437663101952,
18.));
#90405=CARTESIAN_POINT('Ctrl Pts',(-7.38539120988832,-5.88903836524094,
18.));
#90406=CARTESIAN_POINT('Ctrl Pts',(-7.35170722773477,-5.92879601036723,
18.));
#90407=CARTESIAN_POINT('Ctrl Pts',(-7.31768946871676,-5.96828709416038,
18.));
#90408=CARTESIAN_POINT('Ctrl Pts',(-7.28334090389888,-6.00750717725608,
18.));
#90409=CARTESIAN_POINT('Ctrl Pts',(-7.25650547538877,-6.03814856625314,
18.));
#90410=CARTESIAN_POINT('Ctrl Pts',(-7.22947175915789,-6.06862028964852,
18.));
#90411=CARTESIAN_POINT('Ctrl Pts',(-7.20225223828727,-6.0989084687769,18.));
#90412=CARTESIAN_POINT('Ctrl Pts',(-7.04281668321099,-6.27631837523831,
18.));
#90413=CARTESIAN_POINT('Ctrl Pts',(-6.8769088257654,-6.44754939973975,18.));
#90414=CARTESIAN_POINT('Ctrl Pts',(-6.70488545274962,-6.61223355200001,
18.));
#90415=CARTESIAN_POINT('Ctrl Pts',(-6.53342044592134,-6.77638316025832,
18.));
#90416=CARTESIAN_POINT('Ctrl Pts',(-6.35587907752285,-6.93402877733524,
18.));
#90417=CARTESIAN_POINT('Ctrl Pts',(-6.17257983213519,-7.08476792573877,
18.));
#90418=CARTESIAN_POINT('Ctrl Pts',(-5.99170876215547,-7.23351022416951,
18.));
#90419=CARTESIAN_POINT('Ctrl Pts',(-5.80523086450408,-7.37552817919547,
18.));
#90420=CARTESIAN_POINT('Ctrl Pts',(-5.6134254389644,-7.51039211345532,18.));
#90421=CARTESIAN_POINT('Ctrl Pts',(-5.5561940083516,-7.55063318522919,18.));
#90422=CARTESIAN_POINT('Ctrl Pts',(-5.49848810023155,-7.5902370047748,18.));
#90423=CARTESIAN_POINT('Ctrl Pts',(-5.44031476324441,-7.62919132931695,
18.));
#90424=CARTESIAN_POINT('Ctrl Pts',(-5.4406043999737,-7.62923403168952,4.));
#90425=CARTESIAN_POINT('Ctrl Pts',(-5.63890667642695,-7.49673345057434,
4.));
#90426=CARTESIAN_POINT('Ctrl Pts',(-5.83187819659435,-7.35682734686391,
4.));
#90427=CARTESIAN_POINT('Ctrl Pts',(-6.01906043119416,-7.20976889497537,
4.));
#90428=CARTESIAN_POINT('Ctrl Pts',(-6.06595632464851,-7.17292545464531,
4.));
#90429=CARTESIAN_POINT('Ctrl Pts',(-6.11248873150584,-7.13563283968316,
4.));
#90430=CARTESIAN_POINT('Ctrl Pts',(-6.15865021542981,-7.09789457099519,
4.));
#90431=CARTESIAN_POINT('Ctrl Pts',(-6.34204542282573,-6.94796400064803,
4.));
#90432=CARTESIAN_POINT('Ctrl Pts',(-6.51958844489126,-6.79100259370661,
4.));
#90433=CARTESIAN_POINT('Ctrl Pts',(-6.69101403836337,-6.62745756012925,
4.));
#90434=CARTESIAN_POINT('Ctrl Pts',(-6.81071898340218,-6.51325553895363,
4.));
#90435=CARTESIAN_POINT('Ctrl Pts',(-6.92744041708859,-6.39584230707921,
4.));
#90436=CARTESIAN_POINT('Ctrl Pts',(-7.04107814220401,-6.27535881881818,
4.));
#90437=CARTESIAN_POINT('Ctrl Pts',(-7.09297519101191,-6.22033538831146,
4.));
#90438=CARTESIAN_POINT('Ctrl Pts',(-7.14422896803321,-6.16467149349175,
4.));
#90439=CARTESIAN_POINT('Ctrl Pts',(-7.19482929716662,-6.10837999905884,
4.));
#90440=CARTESIAN_POINT('Ctrl Pts',(-7.22002600107554,-6.08034934901944,
4.));
#90441=CARTESIAN_POINT('Ctrl Pts',(-7.24506190537271,-6.05216166512634,
4.));
#90442=CARTESIAN_POINT('Ctrl Pts',(-7.26993182670183,-6.02382294123104,
4.));
#90443=CARTESIAN_POINT('Ctrl Pts',(-7.32949916007229,-5.9559472856861,4.));
#90444=CARTESIAN_POINT('Ctrl Pts',(-7.38807638127959,-5.8872485811258,4.));
#90445=CARTESIAN_POINT('Ctrl Pts',(-7.44564690314271,-5.81775662713007,
4.));
#90446=CARTESIAN_POINT('Ctrl Pts',(-7.59853619808971,-5.63320773809693,
4.));
#90447=CARTESIAN_POINT('Ctrl Pts',(-7.74433637265751,-5.44305767811413,
4.));
#90448=CARTESIAN_POINT('Ctrl Pts',(-7.88277765536633,-5.24776290323712,
4.));
#90449=CARTESIAN_POINT('Ctrl Pts',(-8.02123619232692,-5.05244378832838,
4.));
#90450=CARTESIAN_POINT('Ctrl Pts',(-8.15233441656134,-4.85197814519116,
4.));
#90451=CARTESIAN_POINT('Ctrl Pts',(-8.27576400153287,-4.64678738411282,
4.));
#90452=CARTESIAN_POINT('Ctrl Pts',(-8.34639728459589,-4.52936580230562,
4.));
#90453=CARTESIAN_POINT('Ctrl Pts',(-8.41451852921977,-4.41039625175062,
4.));
#90454=CARTESIAN_POINT('Ctrl Pts',(-8.48006348530507,-4.28995353694912,
4.));
#90455=CARTESIAN_POINT('Ctrl Pts',(-8.52315852127724,-4.21076387176417,
4.));
#90456=CARTESIAN_POINT('Ctrl Pts',(-8.56513975274644,-4.13093731242842,
4.));
#90457=CARTESIAN_POINT('Ctrl Pts',(-8.60598770490748,-4.05049453408062,
4.));
#90458=CARTESIAN_POINT('Ctrl Pts',(-8.62649497932659,-4.01010910364066,
4.));
#90459=CARTESIAN_POINT('Ctrl Pts',(-8.64671849536238,-3.96956421778801,
4.));
#90460=CARTESIAN_POINT('Ctrl Pts',(-8.6666390866119,-3.9288971669964,4.));
#90461=CARTESIAN_POINT('Ctrl Pts',(-8.75648890768642,-3.74547252906847,
4.));
#90462=CARTESIAN_POINT('Ctrl Pts',(-8.84025123269583,-3.55942237588939,
4.));
#90463=CARTESIAN_POINT('Ctrl Pts',(-8.91776910989646,-3.37102286161559,
4.));
#90464=CARTESIAN_POINT('Ctrl Pts',(-9.00791436630044,-3.1519337542521,4.));
#90465=CARTESIAN_POINT('Ctrl Pts',(-9.08961652951227,-2.92966789467907,
4.));
#90466=CARTESIAN_POINT('Ctrl Pts',(-9.16289515281366,-2.70474471828656,
4.));
#90467=CARTESIAN_POINT('Ctrl Pts',(-9.23731564864513,-2.47631665076847,
4.));
#90468=CARTESIAN_POINT('Ctrl Pts',(-9.30304826291371,-2.24514723374452,
4.));
#90469=CARTESIAN_POINT('Ctrl Pts',(-9.36006571799165,-2.01175648923436,
4.));
#90470=CARTESIAN_POINT('Ctrl Pts',(-9.41722423408095,-1.77778833672838,
4.));
#90471=CARTESIAN_POINT('Ctrl Pts',(-9.46562455384306,-1.54158720587045,
4.));
#90472=CARTESIAN_POINT('Ctrl Pts',(-9.50518897333799,-1.30366226406109,
4.));
#90473=CARTESIAN_POINT('Ctrl Pts',(-9.54451505536745,-1.06717059053488,
4.));
#90474=CARTESIAN_POINT('Ctrl Pts',(-9.57511144928619,-0.828975161295982,
4.));
#90475=CARTESIAN_POINT('Ctrl Pts',(-9.59685078292151,-0.589571184533304,
4.));
#90476=CARTESIAN_POINT('Ctrl Pts',(-9.60170018041594,-0.536167291638293,
4.));
#90477=CARTESIAN_POINT('Ctrl Pts',(-9.60610864276964,-0.482703263990903,
4.));
#90478=CARTESIAN_POINT('Ctrl Pts',(-9.61007440021997,-0.429184616207386,
4.));
#90479=CARTESIAN_POINT('Ctrl Pts',(-9.62255729760149,-0.260725552170613,
4.));
#90480=CARTESIAN_POINT('Ctrl Pts',(-9.63062282883421,-0.0921565796354109,
4.));
#90481=CARTESIAN_POINT('Ctrl Pts',(-9.63427539043941,0.0763415761908876,
4.));
#90482=CARTESIAN_POINT('Ctrl Pts',(-9.6395510673353,0.31971647955428,4.));
#90483=CARTESIAN_POINT('Ctrl Pts',(-9.63562264690952,0.562944862804888,
4.));
#90484=CARTESIAN_POINT('Ctrl Pts',(-9.62246124849151,0.805502024763583,
4.));
#90485=CARTESIAN_POINT('Ctrl Pts',(-9.61376654195987,0.965740570349518,
4.));
#90486=CARTESIAN_POINT('Ctrl Pts',(-9.60104133774746,1.12568650575829,4.));
#90487=CARTESIAN_POINT('Ctrl Pts',(-9.58426497005538,1.28519040638768,4.));
#90488=CARTESIAN_POINT('Ctrl Pts',(-9.55895733896447,1.52580660822461,4.00000000000001));
#90489=CARTESIAN_POINT('Ctrl Pts',(-9.52443315490438,1.76541730862835,4.));
#90490=CARTESIAN_POINT('Ctrl Pts',(-9.48091210802519,2.00354972609759,4.));
#90491=CARTESIAN_POINT('Ctrl Pts',(-9.43726373818328,2.24237881166393,4.));
#90492=CARTESIAN_POINT('Ctrl Pts',(-9.38456561231773,2.47972158484106,4.00000000000001));
#90493=CARTESIAN_POINT('Ctrl Pts',(-9.3229878038817,2.71509158677534,4.));
#90494=CARTESIAN_POINT('Ctrl Pts',(-9.28748541748832,2.8507930182864,4.));
#90495=CARTESIAN_POINT('Ctrl Pts',(-9.24903044791309,2.98583846655917,4.));
#90496=CARTESIAN_POINT('Ctrl Pts',(-9.20764807916007,3.12013200861045,4.));
#90497=CARTESIAN_POINT('Ctrl Pts',(-9.19463326690819,3.16236751346685,4.));
#90498=CARTESIAN_POINT('Ctrl Pts',(-9.18132886310879,3.20452862831681,4.));
#90499=CARTESIAN_POINT('Ctrl Pts',(-9.16773554415993,3.24661231613881,4.));
#90500=CARTESIAN_POINT('Ctrl Pts',(-9.15670129834845,3.28077334464322,4.));
#90501=CARTESIAN_POINT('Ctrl Pts',(-9.14547611387815,3.31488477940298,4.00000000000001));
#90502=CARTESIAN_POINT('Ctrl Pts',(-9.13406922931753,3.34891920626068,4.00000000000001));
#90503=CARTESIAN_POINT('Ctrl Pts',(-9.05631917672066,3.58090003014193,4.00000000000001));
#90504=CARTESIAN_POINT('Ctrl Pts',(-8.9700425839685,3.80958444813462,4.));
#90505=CARTESIAN_POINT('Ctrl Pts',(-8.87551055116939,4.03450558990744,4.));
#90506=CARTESIAN_POINT('Ctrl Pts',(-8.78048518937392,4.26060051497725,4.));
#90507=CARTESIAN_POINT('Ctrl Pts',(-8.67711781422885,4.48289341815704,4.));
#90508=CARTESIAN_POINT('Ctrl Pts',(-8.5656314199461,4.7009025036125,4.));
#90509=CARTESIAN_POINT('Ctrl Pts',(-8.45449720704987,4.91822290644901,4.));
#90510=CARTESIAN_POINT('Ctrl Pts',(-8.33529494633942,5.13128713343155,4.));
#90511=CARTESIAN_POINT('Ctrl Pts',(-8.20819692963572,5.33960104088448,4.));
#90512=CARTESIAN_POINT('Ctrl Pts',(-8.12092504012807,5.4826398449952,4.));
#90513=CARTESIAN_POINT('Ctrl Pts',(-8.02992938519569,5.6234385784565,4.));
#90514=CARTESIAN_POINT('Ctrl Pts',(-7.9352532849449,5.76183032119093,4.));
#90515=CARTESIAN_POINT('Ctrl Pts',(-7.82259240106539,5.92651112254192,4.));
#90516=CARTESIAN_POINT('Ctrl Pts',(-7.70472028337977,6.08778406995721,4.));
#90517=CARTESIAN_POINT('Ctrl Pts',(-7.58184069322956,6.24546702512108,4.));
#90518=CARTESIAN_POINT('Ctrl Pts',(-7.52808087253885,6.31445331800527,4.));
#90519=CARTESIAN_POINT('Ctrl Pts',(-7.47336236631123,6.38275226745228,4.));
#90520=CARTESIAN_POINT('Ctrl Pts',(-7.4177012476084,6.45034764911358,4.));
#90521=CARTESIAN_POINT('Ctrl Pts',(-7.38744554517405,6.48709045632159,4.));
#90522=CARTESIAN_POINT('Ctrl Pts',(-7.35691132086333,6.52362537091555,4.));
#90523=CARTESIAN_POINT('Ctrl Pts',(-7.32610108765794,6.55994970757211,4.));
#90524=CARTESIAN_POINT('Ctrl Pts',(-7.30425531243344,6.58570521836257,4.));
#90525=CARTESIAN_POINT('Ctrl Pts',(-7.28227098144389,6.61135450032982,4.));
#90526=CARTESIAN_POINT('Ctrl Pts',(-7.26016370234522,6.63687994473654,4.));
#90527=CARTESIAN_POINT('Ctrl Pts',(-7.10051291614676,6.82121548641077,4.));
#90528=CARTESIAN_POINT('Ctrl Pts',(-6.93426438810104,6.99931954457605,4.));
#90529=CARTESIAN_POINT('Ctrl Pts',(-6.76187972113722,7.17093268814279,4.));
#90530=CARTESIAN_POINT('Ctrl Pts',(-6.58682736884097,7.34520157757143,4.));
#90531=CARTESIAN_POINT('Ctrl Pts',(-6.40544712427759,7.51277759797145,4.));
#90532=CARTESIAN_POINT('Ctrl Pts',(-6.21817619061028,7.67336148139723,4.));
#90533=CARTESIAN_POINT('Ctrl Pts',(-6.03066159759768,7.8341543014857,4.));
#90534=CARTESIAN_POINT('Ctrl Pts',(-5.83724049632752,7.98793722962644,4.));
#90535=CARTESIAN_POINT('Ctrl Pts',(-5.63831244115613,8.13437529745182,4.));
#90536=CARTESIAN_POINT('Ctrl Pts',(-5.44040076795292,8.28006517009946,4.));
#90537=CARTESIAN_POINT('Ctrl Pts',(-5.2370377676165,8.4184854581206,4.));
#90538=CARTESIAN_POINT('Ctrl Pts',(-5.02858537665499,8.54926573852366,4.));
#90539=CARTESIAN_POINT('Ctrl Pts',(-4.82013298569347,8.68004601892672,4.));
#90540=CARTESIAN_POINT('Ctrl Pts',(-4.60659073270969,8.80318675135613,4.));
#90541=CARTESIAN_POINT('Ctrl Pts',(-4.38829619315135,8.91827026601966,4.));
#90542=CARTESIAN_POINT('Ctrl Pts',(-4.36127103682207,8.93251775925059,4.));
#90543=CARTESIAN_POINT('Ctrl Pts',(-4.33417301792296,8.94664169673992,4.));
#90544=CARTESIAN_POINT('Ctrl Pts',(-4.30700275658822,8.96064123010968,4.));
#90545=CARTESIAN_POINT('Ctrl Pts',(5.77174310293177,-8.09584396947078,3.66952413717531));
#90546=CARTESIAN_POINT('Ctrl Pts',(7.10709424093549,-7.14384070838492,3.69577555387736));
#90547=CARTESIAN_POINT('Ctrl Pts',(9.2962305957292,-4.5677522174272,3.74827257500505));
#90548=CARTESIAN_POINT('Ctrl Pts',(10.3498486095772,0.394808939182714,3.82701520055842));
#90549=CARTESIAN_POINT('Ctrl Pts',(8.92165680290257,5.2609948509435,3.90575201383539));
#90550=CARTESIAN_POINT('Ctrl Pts',(5.35405107811436,8.86628230701266,3.98448882711236));
#90551=CARTESIAN_POINT('Ctrl Pts',(0.502596015216245,10.3451445080436,4.06322564038934));
#90552=CARTESIAN_POINT('Ctrl Pts',(-4.46939113767733,9.34346938332682,4.14196245366631));
#90553=CARTESIAN_POINT('Ctrl Pts',(-8.36963559720786,6.10119010282693,4.2206992669433));
#90554=CARTESIAN_POINT('Ctrl Pts',(-10.2628888627734,1.39592378273276,4.29943608022025));
#90555=CARTESIAN_POINT('Ctrl Pts',(-9.69515388203774,-3.64410147588179,
4.37817289349724));
#90556=CARTESIAN_POINT('Ctrl Pts',(-6.80257303895417,-7.81027817659755,
4.4569097067742));
#90557=CARTESIAN_POINT('Ctrl Pts',(-2.27877064542789,-10.1035977177542,
4.53564652005118));
#90558=CARTESIAN_POINT('Ctrl Pts',(2.79146869119749,-9.97412460187197,4.61438333332815));
#90559=CARTESIAN_POINT('Ctrl Pts',(7.19232868879842,-7.45291073539475,4.69312014660512));
#90560=CARTESIAN_POINT('Ctrl Pts',(9.8685061716992,-3.14452735022185,4.7718569598821));
#90561=CARTESIAN_POINT('Ctrl Pts',(10.1782679982284,1.91789664855303,4.85059377315908));
#90562=CARTESIAN_POINT('Ctrl Pts',(8.04733486999838,6.5204193848677,4.92933058643604));
#90563=CARTESIAN_POINT('Ctrl Pts',(3.98669332722565,9.5593798530638,5.00806739971302));
#90564=CARTESIAN_POINT('Ctrl Pts',(-1.02993623540529,10.3060515540929,5.08680421298999));
#90565=CARTESIAN_POINT('Ctrl Pts',(-5.79959252323165,8.58138646284841,5.16554102626697));
#90566=CARTESIAN_POINT('Ctrl Pts',(-9.17853713906726,4.79895021206766,5.24427783954394));
#90567=CARTESIAN_POINT('Ctrl Pts',(-10.3565169985255,-0.134248976023967,
5.32301465282091));
#90568=CARTESIAN_POINT('Ctrl Pts',(-9.05105875032658,-5.03525596400226,
5.40175146609789));
#90569=CARTESIAN_POINT('Ctrl Pts',(-5.57520439089005,-8.72883515332142,
5.48048827937486));
#90570=CARTESIAN_POINT('Ctrl Pts',(-0.762445448074686,-10.3292857480735,
5.55922509265183));
#90571=CARTESIAN_POINT('Ctrl Pts',(4.2331438885583,-9.4528281455708,5.63796190592881));
#90572=CARTESIAN_POINT('Ctrl Pts',(8.21364766592046,-6.30963225149706,5.71669871920578));
#90573=CARTESIAN_POINT('Ctrl Pts',(10.2245620898643,-1.65341984992491,5.79543553248275));
#90574=CARTESIAN_POINT('Ctrl Pts',(9.78368049639725,3.39927390393817,5.87417234575973));
#90575=CARTESIAN_POINT('Ctrl Pts',(6.99672396438769,7.63683971912566,5.95290915903669));
#90576=CARTESIAN_POINT('Ctrl Pts',(2.53198995887729,10.0431316817874,6.03164597231369));
#90577=CARTESIAN_POINT('Ctrl Pts',(-2.53990187331711,10.0411336811845,6.11038278559064));
#90578=CARTESIAN_POINT('Ctrl Pts',(-7.00273864350857,7.63132482733166,6.18911959886763));
#90579=CARTESIAN_POINT('Ctrl Pts',(-9.78635565189662,3.39156456286966,6.26785641214459));
#90580=CARTESIAN_POINT('Ctrl Pts',(-10.2232562335718,-1.66147498093125,
6.34659322542156));
#90581=CARTESIAN_POINT('Ctrl Pts',(-8.20867393528745,-6.3161015946277,6.42533003869855));
#90582=CARTESIAN_POINT('Ctrl Pts',(-4.22569495792512,-9.45616038633497,
6.50406685197551));
#90583=CARTESIAN_POINT('Ctrl Pts',(0.770583364441047,-10.3286818330304,
6.5828036652525));
#90584=CARTESIAN_POINT('Ctrl Pts',(5.58207986364352,-8.72443989751954,6.66154047852946));
#90585=CARTESIAN_POINT('Ctrl Pts',(9.05502307731348,-5.02812332772831,6.74027729180644));
#90586=CARTESIAN_POINT('Ctrl Pts',(10.3566195552168,-0.126089325581968,
6.8190141050834));
#90587=CARTESIAN_POINT('Ctrl Pts',(9.17475333260671,4.80618023125926,6.89775091836039));
#90588=CARTESIAN_POINT('Ctrl Pts',(5.79282969102316,8.58595313872173,6.97648773163736));
#90589=CARTESIAN_POINT('Ctrl Pts',(1.02181606777311,10.3068598056424,7.05522454491433));
#90590=CARTESIAN_POINT('Ctrl Pts',(-3.99422365473359,9.55623589733384,7.13396135819131));
#90591=CARTESIAN_POINT('Ctrl Pts',(-8.05246962888899,6.514077064738,7.21269817146827));
#90592=CARTESIAN_POINT('Ctrl Pts',(-10.1797758920949,1.9098769374614,7.29143498474526));
#90593=CARTESIAN_POINT('Ctrl Pts',(-9.86602563171077,-3.15230159787276,
7.37017179802222));
#90594=CARTESIAN_POINT('Ctrl Pts',(-7.186454504003,-7.45857484989058,7.44890861129921));
#90595=CARTESIAN_POINT('Ctrl Pts',(-2.78360952091465,-9.9763212240083,7.52764542457617));
#90596=CARTESIAN_POINT('Ctrl Pts',(2.28673033162688,-10.1017984299799,7.60638223785315));
#90597=CARTESIAN_POINT('Ctrl Pts',(6.80872432146195,-7.80491769616169,7.68511905113011));
#90598=CARTESIAN_POINT('Ctrl Pts',(9.69802215978954,-3.63645889812552,7.7638558644071));
#90599=CARTESIAN_POINT('Ctrl Pts',(10.261785476531,1.40400354813729,7.84259267768406));
#90600=CARTESIAN_POINT('Ctrl Pts',(8.36482680423332,6.10779335478084,7.92132949096105));
#90601=CARTESIAN_POINT('Ctrl Pts',(4.46202681915855,9.34696655576745,8.000066304238));
#90602=CARTESIAN_POINT('Ctrl Pts',(-0.510743643733886,10.3447865159176,
8.07880311751499));
#90603=CARTESIAN_POINT('Ctrl Pts',(-5.36104047688882,8.86198127591595,8.15753993079196));
#90604=CARTESIAN_POINT('Ctrl Pts',(-8.92578810266849,5.25411970512538,8.23627674406893));
#90605=CARTESIAN_POINT('Ctrl Pts',(-10.3501788574171,0.38634796363252,8.31501355734591));
#90606=CARTESIAN_POINT('Ctrl Pts',(-9.29265135698636,-4.57406798014904,
8.39375037062287));
#90607=CARTESIAN_POINT('Ctrl Pts',(-6.00679511367681,-8.43764656713195,
8.47248718389986));
#90608=CARTESIAN_POINT('Ctrl Pts',(-1.28054110979408,-10.2779220465838,
8.55122399717681));
#90609=CARTESIAN_POINT('Ctrl Pts',(3.75277989270658,-9.65360607267681,8.62996081045381));
#90610=CARTESIAN_POINT('Ctrl Pts',(7.88620408649619,-6.71440632041701,8.70869762373077));
#90611=CARTESIAN_POINT('Ctrl Pts',(10.1285581687469,-2.16512737542992,8.78743443700775));
#90612=CARTESIAN_POINT('Ctrl Pts',(9.9421374671065,2.90333768526539,8.86617125028472));
#90613=CARTESIAN_POINT('Ctrl Pts',(7.37164468178136,7.27559769469767,8.9449080635617));
#90614=CARTESIAN_POINT('Ctrl Pts',(3.03347041399593,9.90320778217525,9.02364487683867));
#90615=CARTESIAN_POINT('Ctrl Pts',(-2.03211404647875,10.156080918919,9.10238169011564));
#90616=CARTESIAN_POINT('Ctrl Pts',(-6.61040828539873,7.97357946156285,9.18111850339261));
#90617=CARTESIAN_POINT('Ctrl Pts',(-9.603561511421,3.8790557389497,9.25985531666959));
#90618=CARTESIAN_POINT('Ctrl Pts',(-10.2938313807125,-1.14564507373933,
9.33859212994656));
#90619=CARTESIAN_POINT('Ctrl Pts',(-8.51569482230081,-5.89562624518926,
9.41732894322354));
#90620=CARTESIAN_POINT('Ctrl Pts',(-4.69553959675684,-9.23186736390931,
9.4960657565005));
#90621=CARTESIAN_POINT('Ctrl Pts',(0.250581238043845,-10.3543554204337,
9.57480256977749));
#90622=CARTESIAN_POINT('Ctrl Pts',(5.13661401468883,-8.99392370401415,9.65353938305445));
#90623=CARTESIAN_POINT('Ctrl Pts',(8.7909138649284,-5.47679655902376,9.73227619633144));
#90624=CARTESIAN_POINT('Ctrl Pts',(10.3371989743949,-0.646362509196422,
9.8110130096084));
#90625=CARTESIAN_POINT('Ctrl Pts',(9.40467833611481,4.33906585842369,9.88974982288538));
#90626=CARTESIAN_POINT('Ctrl Pts',(6.21696547671049,8.28400913754416,9.96848663616235));
#90627=CARTESIAN_POINT('Ctrl Pts',(1.53845711309042,10.2424907537526,10.0472234494393));
#90628=CARTESIAN_POINT('Ctrl Pts',(-3.50896514529322,9.74487715359423,10.1259602627163));
#90629=CARTESIAN_POINT('Ctrl Pts',(-7.71495608438624,6.91049345166589,10.2046970759932));
#90630=CARTESIAN_POINT('Ctrl Pts',(-10.0709412788904,2.41900989800939,10.2834338892702));
#90631=CARTESIAN_POINT('Ctrl Pts',(-10.0119679155524,-2.65253946011637,
10.3621707025472));
#90632=CARTESIAN_POINT('Ctrl Pts',(-7.5521774956019,-7.0880238574972,10.4409075158241));
#90633=CARTESIAN_POINT('Ctrl Pts',(-3.28141477740401,-9.82383754895001,
10.5196443291011));
#90634=CARTESIAN_POINT('Ctrl Pts',(1.77621388302032,-10.2039468526297,10.5983811423781));
#90635=CARTESIAN_POINT('Ctrl Pts',(6.40791583028337,-8.13720356397264,10.6771179556551));
#90636=CARTESIAN_POINT('Ctrl Pts',(9.50303338650133,-4.11920181401277,10.755854768932));
#90637=CARTESIAN_POINT('Ctrl Pts',(10.3193736996929,0.886562787179303,10.834591582209));
#90638=CARTESIAN_POINT('Ctrl Pts',(8.66118267191835,5.67973431184827,10.913328395486));
#90639=CARTESIAN_POINT('Ctrl Pts',(4.9260857586507,9.11093552978749,10.992065208763));
#90640=CARTESIAN_POINT('Ctrl Pts',(0.0097394834735438,10.3573825009983,
11.0708020220399));
#90641=CARTESIAN_POINT('Ctrl Pts',(-4.90894226842936,9.1201838213247,11.1495388353169));
#90642=CARTESIAN_POINT('Ctrl Pts',(-8.65048557688362,5.69601320343043,11.2282756485939));
#90643=CARTESIAN_POINT('Ctrl Pts',(-10.3176881067681,0.905968686535361,
11.3070124618708));
#90644=CARTESIAN_POINT('Ctrl Pts',(-9.51076349197205,-4.10132233911171,
11.3857492751478));
#90645=CARTESIAN_POINT('Ctrl Pts',(-6.42320799566222,-8.12513791722861,
11.4644860884248));
#90646=CARTESIAN_POINT('Ctrl Pts',(-1.79540112777125,-10.2005883124418,
11.5432229017018));
#90647=CARTESIAN_POINT('Ctrl Pts',(3.26293345328981,-9.8299914755267,11.6219597149788));
#90648=CARTESIAN_POINT('Ctrl Pts',(7.5388338160908,-7.10221457172981,11.7006965282557));
#90649=CARTESIAN_POINT('Ctrl Pts',(10.0069616245548,-2.67136410363949,11.7794333415327));
#90650=CARTESIAN_POINT('Ctrl Pts',(10.075472858561,2.40006537534412,11.8581701548097));
#90651=CARTESIAN_POINT('Ctrl Pts',(7.72793888584071,6.89597184639239,11.9369069680867));
#90652=CARTESIAN_POINT('Ctrl Pts',(3.52728596127422,9.7382606700028,12.0156437813636));
#90653=CARTESIAN_POINT('Ctrl Pts',(-1.51919151754623,10.2453659896824,12.0943805946406));
#90654=CARTESIAN_POINT('Ctrl Pts',(-6.2013748897185,8.29568662659662,12.1731174079176));
#90655=CARTESIAN_POINT('Ctrl Pts',(-9.39650129813868,4.35674540036522,12.2518542211946));
#90656=CARTESIAN_POINT('Ctrl Pts',(-10.3383962959777,-0.626920375199499,
12.3305910344715));
#90657=CARTESIAN_POINT('Ctrl Pts',(-8.80119843467484,-5.46025395407599,
12.4093278477485));
#90658=CARTESIAN_POINT('Ctrl Pts',(-5.15351964706217,-8.98424745745961,
12.4880646610255));
#90659=CARTESIAN_POINT('Ctrl Pts',(-0.270054051639655,-10.3538658451188,
12.5668014743024));
#90660=CARTESIAN_POINT('Ctrl Pts',(4.67816907984897,-9.24068185741022,12.6455382875794));
#90661=CARTESIAN_POINT('Ctrl Pts',(8.50459196034266,-5.91163113849298,12.7242751008564));
#90662=CARTESIAN_POINT('Ctrl Pts',(10.2916585813938,-1.16500247791564,12.8030119141334));
#90663=CARTESIAN_POINT('Ctrl Pts',(9.61083980054881,3.86098762724155,12.8817487274103));
#90664=CARTESIAN_POINT('Ctrl Pts',(6.62539236765973,7.96113328013551,12.9604855406873));
#90665=CARTESIAN_POINT('Ctrl Pts',(2.05121081804228,10.1522411963798,13.0392223539643));
#90666=CARTESIAN_POINT('Ctrl Pts',(-3.01484025814591,9.90889526372077,13.1179591672413));
#90667=CARTESIAN_POINT('Ctrl Pts',(-7.35794855467586,7.28944855227533,13.1966959805182));
#90668=CARTESIAN_POINT('Ctrl Pts',(-9.93665962772858,2.92203055634167,13.2754327937952));
#90669=CARTESIAN_POINT('Ctrl Pts',(-10.1326121740638,-2.14607494266621,
13.3541696070722));
#90670=CARTESIAN_POINT('Ctrl Pts',(-7.89881780743255,-6.69956299877176,
13.4329064203492));
#90671=CARTESIAN_POINT('Ctrl Pts',(-3.77092862556512,-9.64653121232802,
13.5116432336261));
#90672=CARTESIAN_POINT('Ctrl Pts',(1.26120933535224,-10.2803121616975,13.5903800469031));
#90673=CARTESIAN_POINT('Ctrl Pts',(5.99091595511748,-8.4489285207205,13.6691168601801));
#90674=CARTESIAN_POINT('Ctrl Pts',(9.28403255271173,-4.59153641929518,13.747853673457));
#90675=CARTESIAN_POINT('Ctrl Pts',(10.3508871511966,0.36688187842646,13.826590486734));
#90676=CARTESIAN_POINT('Ctrl Pts',(8.93565364939284,5.23732383833744,13.905327300011));
#90677=CARTESIAN_POINT('Ctrl Pts',(5.37769757053005,8.85188318774262,13.984064113288));
#90678=CARTESIAN_POINT('Ctrl Pts',(0.530198001163546,10.3438076745988,14.0628009265649));
#90679=CARTESIAN_POINT('Ctrl Pts',(-4.44444025015958,9.35534168228432,14.1415377398419));
#90680=CARTESIAN_POINT('Ctrl Pts',(-8.3533251900779,6.12351413800404,14.2202745531189));
#90681=CARTESIAN_POINT('Ctrl Pts',(-10.2591268435809,1.42330022723409,14.2990113663959));
#90682=CARTESIAN_POINT('Ctrl Pts',(-9.70484403419201,-3.6182135649424,14.3777481796728));
#90683=CARTESIAN_POINT('Ctrl Pts',(-6.82339085374557,-7.79209884347897,
14.4564849929498));
#90684=CARTESIAN_POINT('Ctrl Pts',(-2.30572456476937,-10.0974799510048,
14.5352218062268));
#90685=CARTESIAN_POINT('Ctrl Pts',(2.76484230375725,-9.98153866720356,14.6139586195037));
#90686=CARTESIAN_POINT('Ctrl Pts',(7.1724145824397,-7.47207709991883,14.6926954327807));
#90687=CARTESIAN_POINT('Ctrl Pts',(9.86007970482085,-3.17085088645072,14.7714322460577));
#90688=CARTESIAN_POINT('Ctrl Pts',(10.1833497617602,1.8907286318198,14.8501690593347));
#90689=CARTESIAN_POINT('Ctrl Pts',(8.06470630002883,6.49892140464869,14.9289058726116));
#90690=CARTESIAN_POINT('Ctrl Pts',(4.01218883820157,9.54870713008499,15.0076426858886));
#90691=CARTESIAN_POINT('Ctrl Pts',(-1.00243032814087,10.3087632898786,15.0863794991656));
#90692=CARTESIAN_POINT('Ctrl Pts',(-5.77667199326021,8.596832428971,15.1651163124426));
#90693=CARTESIAN_POINT('Ctrl Pts',(-9.16569820734604,4.82342653114775,15.2438531257195));
#90694=CARTESIAN_POINT('Ctrl Pts',(-10.3568383736971,-0.106611587730943,
15.3225899389965));
#90695=CARTESIAN_POINT('Ctrl Pts',(-9.06446336801841,-5.01108481063476,
15.4013267522735));
#90696=CARTESIAN_POINT('Ctrl Pts',(-5.59847789469375,-8.71392634764388,
15.4800635655504));
#90697=CARTESIAN_POINT('Ctrl Pts',(-0.790006974550176,-10.3272143441326,
15.5588003788274));
#90698=CARTESIAN_POINT('Ctrl Pts',(4.20790344793164,-9.46409085451224,15.6375371921044));
#90699=CARTESIAN_POINT('Ctrl Pts',(8.19678083559,-6.33152833546188,15.7162740053814));
#90700=CARTESIAN_POINT('Ctrl Pts',(10.2201134467006,-1.68069874342431,15.7950108186583));
#90701=CARTESIAN_POINT('Ctrl Pts',(9.79271680154967,3.3731535355307,15.8737476319353));
#90702=CARTESIAN_POINT('Ctrl Pts',(7.01707835958532,7.6181414022353,15.9524844452123));
#90703=CARTESIAN_POINT('Ctrl Pts',(2.55878156758079,10.0363391742379,16.0312212584893));
#90704=CARTESIAN_POINT('Ctrl Pts',(-2.51309753742156,10.0478757901385,16.1099580717662));
#90705=CARTESIAN_POINT('Ctrl Pts',(-6.98234911873795,7.64998483123455,16.1886948850432));
#90706=CARTESIAN_POINT('Ctrl Pts',(-9.77727023854604,3.41766789014466,16.2674316983202));
#90707=CARTESIAN_POINT('Ctrl Pts',(-10.2276535660293,-1.63418776815829,
16.3461685115972));
#90708=CARTESIAN_POINT('Ctrl Pts',(-8.22549955600462,-6.29417383024248,
16.4249053248741));
#90709=CARTESIAN_POINT('Ctrl Pts',(-4.25091417271837,-9.44485022414144,
16.5036421381511));
#90710=CARTESIAN_POINT('Ctrl Pts',(0.743017991801421,-10.3307014064138,
16.5823789514281));
#90711=CARTESIAN_POINT('Ctrl Pts',(5.55877836081692,-8.73930489202781,16.6611157647051));
#90712=CARTESIAN_POINT('Ctrl Pts',(9.04157302787004,-5.05226925709063,16.739852577982));
#90713=CARTESIAN_POINT('Ctrl Pts',(10.3562461980019,-0.1537260051618,16.818589391259));
#90714=CARTESIAN_POINT('Ctrl Pts',(9.18754622001517,4.78167970197118,16.897326204536));
#90715=CARTESIAN_POINT('Ctrl Pts',(5.81572111097091,8.57046430229322,16.976063017813));
#90716=CARTESIAN_POINT('Ctrl Pts',(1.04931686630384,10.3040959400471,17.0547998310899));
#90717=CARTESIAN_POINT('Ctrl Pts',(-3.96870819410001,9.56686143762709,17.1335366443669));
#90718=CARTESIAN_POINT('Ctrl Pts',(-8.03505764881968,6.5355408136042,17.2122734576439));
#90719=CARTESIAN_POINT('Ctrl Pts',(-10.1746433338992,1.93703830392091,17.2910102709208));
#90720=CARTESIAN_POINT('Ctrl Pts',(-9.87440201338592,-3.12596799325867,
17.3697470841978));
#90721=CARTESIAN_POINT('Ctrl Pts',(-7.2063336236016,-7.43935994600553,17.4484838974748));
#90722=CARTESIAN_POINT('Ctrl Pts',(-2.8102197948658,-9.96887867130796,17.5272207107518));
#90723=CARTESIAN_POINT('Ctrl Pts',(2.25976083640424,-10.1078236336547,17.6059575240287));
#90724=CARTESIAN_POINT('Ctrl Pts',(6.787880338596,-7.82313910163977,17.6846943373057));
#90725=CARTESIAN_POINT('Ctrl Pts',(9.68826788900902,-3.66217042766011,17.7634311505827));
#90726=CARTESIAN_POINT('Ctrl Pts',(10.265525559982,1.37630858348745,17.8421679638596));
#90727=CARTESIAN_POINT('Ctrl Pts',(8.38104198679141,6.0860905800779,17.9209047771366));
#90728=CARTESIAN_POINT('Ctrl Pts',(5.7850274219278,8.25090580895841,17.9733959859879));
#90729=CARTESIAN_POINT('Ctrl Pts',(4.30727168806404,8.96120073717495,17.9996415904136));
#90730=CARTESIAN_POINT('Ctrl Pts',(5.66080476763815,-7.94023422788095,3.77985954388849));
#90731=CARTESIAN_POINT('Ctrl Pts',(6.97048919982341,-7.00652936557954,3.80611096059054));
#90732=CARTESIAN_POINT('Ctrl Pts',(9.11754829327675,-4.47995572025153,3.85860798171824));
#90733=CARTESIAN_POINT('Ctrl Pts',(10.1509147771437,0.3872203397439,3.93735060727159));
#90734=CARTESIAN_POINT('Ctrl Pts',(8.75017416132892,5.15987357781277,4.01608742054857));
#90735=CARTESIAN_POINT('Ctrl Pts',(5.25114117670495,8.69586401537322,4.09482423382554));
#90736=CARTESIAN_POINT('Ctrl Pts',(0.492935646717676,10.1463010928695,4.17356104710252));
#90737=CARTESIAN_POINT('Ctrl Pts',(-4.38348523304028,9.16387910691155,4.25229786037949));
#90738=CARTESIAN_POINT('Ctrl Pts',(-8.20876332281697,5.98391948609178,4.33103467365646));
#90739=CARTESIAN_POINT('Ctrl Pts',(-10.0656264785274,1.36909281366648,4.40977148693343));
#90740=CARTESIAN_POINT('Ctrl Pts',(-9.5088038985219,-3.57405841537725,4.48850830021041));
#90741=CARTESIAN_POINT('Ctrl Pts',(-6.6718211819854,-7.66015727834556,4.56724511348738));
#90742=CARTESIAN_POINT('Ctrl Pts',(-2.23497052865009,-9.90939705925389,
4.64598192676436));
#90743=CARTESIAN_POINT('Ctrl Pts',(2.73781403538504,-9.78241253852996,4.72471874004133));
#90744=CARTESIAN_POINT('Ctrl Pts',(7.05408536136851,-7.30965877574727,4.8034555533183));
#90745=CARTESIAN_POINT('Ctrl Pts',(9.67882419400217,-3.08408657465411,4.88219236659527));
#90746=CARTESIAN_POINT('Ctrl Pts',(9.9826321066513,1.88103286968048,4.96092917987225));
#90747=CARTESIAN_POINT('Ctrl Pts',(7.89265751896129,6.39509078671749,5.03966599314922));
#90748=CARTESIAN_POINT('Ctrl Pts',(3.91006532886167,9.37563957418694,5.1184028064262));
#90749=CARTESIAN_POINT('Ctrl Pts',(-1.01013989149727,10.1079595422914,5.19713961970317));
#90750=CARTESIAN_POINT('Ctrl Pts',(-5.68811889586561,8.41644413750198,5.27587643298014));
#90751=CARTESIAN_POINT('Ctrl Pts',(-9.00211701563495,4.70670987181179,5.35461324625711));
#90752=CARTESIAN_POINT('Ctrl Pts',(-10.1574549933796,-0.131668584338251,
5.43335005953409));
#90753=CARTESIAN_POINT('Ctrl Pts',(-8.87708888151934,-4.93847360476317,
5.51208687281107));
#90754=CARTESIAN_POINT('Ctrl Pts',(-5.46804371464078,-8.56105872535287,
5.59082368608803));
#90755=CARTESIAN_POINT('Ctrl Pts',(-0.747790528884207,-10.1307471531937,
5.66956049936502));
#90756=CARTESIAN_POINT('Ctrl Pts',(4.15177887842533,-9.27113589080745,5.74829731264197));
#90757=CARTESIAN_POINT('Ctrl Pts',(8.05577362639801,-6.18835518046099,5.82703412591897));
#90758=CARTESIAN_POINT('Ctrl Pts',(10.02803638227,-1.62163956407002,5.90577093919592));
#90759=CARTESIAN_POINT('Ctrl Pts',(9.59562894802464,3.33393665981891,5.98450775247291));
#90760=CARTESIAN_POINT('Ctrl Pts',(6.86224034388074,7.49005247128131,6.06324456574988));
#90761=CARTESIAN_POINT('Ctrl Pts',(2.48332272854344,9.85009323741409,6.14198137902686));
#90762=CARTESIAN_POINT('Ctrl Pts',(-2.49108256854038,9.84813364026348,6.22071819230382));
#90763=CARTESIAN_POINT('Ctrl Pts',(-6.86813941520742,7.48464358089862,6.29945500558081));
#90764=CARTESIAN_POINT('Ctrl Pts',(-9.59825268451726,3.3263754995424,6.37819181885778));
#90765=CARTESIAN_POINT('Ctrl Pts',(-10.0267556257647,-1.62953986787626,
6.45692863213474));
#90766=CARTESIAN_POINT('Ctrl Pts',(-8.05089549554946,-6.1947001767272,6.53566544541173));
#90767=CARTESIAN_POINT('Ctrl Pts',(-4.14447312325044,-9.27440408276756,
6.6144022586887));
#90768=CARTESIAN_POINT('Ctrl Pts',(0.755772026837927,-10.1301548459661,
6.69313907196567));
#90769=CARTESIAN_POINT('Ctrl Pts',(5.47478703433619,-8.55674795050467,6.77187588524263));
#90770=CARTESIAN_POINT('Ctrl Pts',(8.88097701040999,-4.93147806447222,6.85061269851962));
#90771=CARTESIAN_POINT('Ctrl Pts',(10.1575555788348,-0.123665770058277,
6.92934951179658));
#90772=CARTESIAN_POINT('Ctrl Pts',(8.99840593749619,4.71380092322904,7.00808632507357));
#90773=CARTESIAN_POINT('Ctrl Pts',(5.68148605165791,8.42092303756649,7.08682313835054));
#90774=CARTESIAN_POINT('Ctrl Pts',(1.00217580113035,10.1087522584852,7.16555995162751));
#90775=CARTESIAN_POINT('Ctrl Pts',(-3.91745091638676,9.37255604824544,7.2442967649045));
#90776=CARTESIAN_POINT('Ctrl Pts',(-7.89769358295277,6.38887037195061,7.32303357818146));
#90777=CARTESIAN_POINT('Ctrl Pts',(-9.98411101737842,1.87316730498484,7.40177039145844));
#90778=CARTESIAN_POINT('Ctrl Pts',(-9.67639133232721,-3.09171139394741,
7.4805072047354));
#90779=CARTESIAN_POINT('Ctrl Pts',(-7.04832408393412,-7.31521402063096,
7.55924401801238));
#90780=CARTESIAN_POINT('Ctrl Pts',(-2.73010592575272,-9.7845669395212,7.63798083128934));
#90781=CARTESIAN_POINT('Ctrl Pts',(2.24277722218803,-9.90763235548413,7.71671764456634));
#90782=CARTESIAN_POINT('Ctrl Pts',(6.6778542310533,-7.6548998313894,7.7954544578433));
#90783=CARTESIAN_POINT('Ctrl Pts',(9.51161704527546,-3.56656273515928,7.87419127112028));
#90784=CARTESIAN_POINT('Ctrl Pts',(10.0645443004072,1.37701727837461,7.95292808439723));
#90785=CARTESIAN_POINT('Ctrl Pts',(8.20404695936982,5.99039581732761,8.03166489767423));
#90786=CARTESIAN_POINT('Ctrl Pts',(4.37626246365533,9.16730906040605,8.11040171095119));
#90787=CARTESIAN_POINT('Ctrl Pts',(-0.500926670145997,10.1459499816891,
8.18913852422817));
#90788=CARTESIAN_POINT('Ctrl Pts',(-5.25799623265597,8.69164565414265,8.26787533750514));
#90789=CARTESIAN_POINT('Ctrl Pts',(-8.75422605362463,5.15313057876873,8.34661215078212));
#90790=CARTESIAN_POINT('Ctrl Pts',(-10.1512386773093,0.378921992107938,
8.42534896405908));
#90791=CARTESIAN_POINT('Ctrl Pts',(-9.11403785087162,-4.48615008806894,
8.50408577733605));
#90792=CARTESIAN_POINT('Ctrl Pts',(-5.89133885748571,-8.27546705788142,
8.58282259061303));
#90793=CARTESIAN_POINT('Ctrl Pts',(-1.25592790430966,-10.0803707103944,
8.66155940389002));
#90794=CARTESIAN_POINT('Ctrl Pts',(3.68064793073329,-9.46805467716523,8.74029621716696));
#90795=CARTESIAN_POINT('Ctrl Pts',(7.73462382078804,-6.58534911076854,8.81903303044396));
#90796=CARTESIAN_POINT('Ctrl Pts',(9.93387774688354,-2.12351158927219,8.89776984372092));
#90797=CARTESIAN_POINT('Ctrl Pts',(9.75104022660372,2.84753280208635,8.97650665699791));
#90798=CARTESIAN_POINT('Ctrl Pts',(7.22995473217883,7.13575385859452,9.05524347027487));
#90799=CARTESIAN_POINT('Ctrl Pts',(2.97516425727868,9.71285880686077,9.13398028355186));
#90800=CARTESIAN_POINT('Ctrl Pts',(-1.99305490170695,9.96087148389051,9.21271709682881));
#90801=CARTESIAN_POINT('Ctrl Pts',(-6.48335001587512,7.82031975890077,9.2914539101058));
#90802=CARTESIAN_POINT('Ctrl Pts',(-9.41897201948297,3.80449663635003,9.37019072338278));
#90803=CARTESIAN_POINT('Ctrl Pts',(-10.095974252146,-1.12362469704354,9.44892753665973));
#90804=CARTESIAN_POINT('Ctrl Pts',(-8.35201515212025,-5.7823067592921,9.52766434993672));
#90805=CARTESIAN_POINT('Ctrl Pts',(-4.6052869058661,-9.05442218335658,9.60640116321369));
#90806=CARTESIAN_POINT('Ctrl Pts',(0.245764830780288,-10.1553349628534,
9.68513797649068));
#90807=CARTESIAN_POINT('Ctrl Pts',(5.03788345830874,-8.82105202457739,9.76387478976763));
#90808=CARTESIAN_POINT('Ctrl Pts',(8.621944225689,-5.3715273739328,9.84261160304463));
#90809=CARTESIAN_POINT('Ctrl Pts',(10.1385082798565,-0.633938813358303,
9.92134841632157));
#90810=CARTESIAN_POINT('Ctrl Pts',(9.2239115660119,4.25566492832712,10.0000852295986));
#90811=CARTESIAN_POINT('Ctrl Pts',(6.09746954831168,8.12478268430691,10.0788220428756));
#90812=CARTESIAN_POINT('Ctrl Pts',(1.50888651925018,10.0456204403623,10.1575588561525));
#90813=CARTESIAN_POINT('Ctrl Pts',(-3.44151953226439,9.55757144199531,10.2362956694295));
#90814=CARTESIAN_POINT('Ctrl Pts',(-7.5666673664718,6.77766726278093,10.3150324827065));
#90815=CARTESIAN_POINT('Ctrl Pts',(-9.87736830788399,2.37251425079188,10.3937692959835));
#90816=CARTESIAN_POINT('Ctrl Pts',(-9.81952846810011,-2.60155515489731,
10.4725061092604));
#90817=CARTESIAN_POINT('Ctrl Pts',(-7.40701753538492,-6.95178536710547,
10.5512429225374));
#90818=CARTESIAN_POINT('Ctrl Pts',(-3.21834289663573,-9.63501414422814,
10.6299797358144));
#90819=CARTESIAN_POINT('Ctrl Pts',(1.74207338026517,-10.0078173892998,10.7087165490914));
#90820=CARTESIAN_POINT('Ctrl Pts',(6.2847496563502,-7.98079885204531,10.7874533623683));
#90821=CARTESIAN_POINT('Ctrl Pts',(9.32037613974987,-4.0400268778045,10.8661901756453));
#90822=CARTESIAN_POINT('Ctrl Pts',(10.121025623713,0.869522215901469,10.9449269889223));
#90823=CARTESIAN_POINT('Ctrl Pts',(8.49470658832261,5.57056447212576,11.0236638021992));
#90824=CARTESIAN_POINT('Ctrl Pts',(4.83140175351872,8.93581477291791,11.1024006154762));
#90825=CARTESIAN_POINT('Ctrl Pts',(0.00955228143353725,10.1583038600802,
11.1811374287532));
#90826=CARTESIAN_POINT('Ctrl Pts',(-4.81458777731637,8.94488530358647,11.2598742420302));
#90827=CARTESIAN_POINT('Ctrl Pts',(-8.48421510152349,5.58653046808861,11.3386110553071));
#90828=CARTESIAN_POINT('Ctrl Pts',(-10.1193724294707,0.888555115605388,
11.4173478685841));
#90829=CARTESIAN_POINT('Ctrl Pts',(-9.32795766531719,-4.02249106324075,
11.4960846818611));
#90830=CARTESIAN_POINT('Ctrl Pts',(-6.29974789191615,-7.96896511838893,
11.5748214951381));
#90831=CARTESIAN_POINT('Ctrl Pts',(-1.7608918281113,-10.0045234034157,11.653558308415));
#90832=CARTESIAN_POINT('Ctrl Pts',(3.20021680096722,-9.64104978654342,11.732295121692));
#90833=CARTESIAN_POINT('Ctrl Pts',(7.39393033395425,-6.965703322453,11.811031934969));
#90834=CARTESIAN_POINT('Ctrl Pts',(9.81461840272779,-2.62001797105254,11.8897687482459));
#90835=CARTESIAN_POINT('Ctrl Pts',(9.88181278632787,2.35393385968446,11.9685055615229));
#90836=CARTESIAN_POINT('Ctrl Pts',(7.57940062626177,6.76342477642978,12.0472423747999));
#90837=CARTESIAN_POINT('Ctrl Pts',(3.4594882049171,9.55108213344652,12.1259791880769));
#90838=CARTESIAN_POINT('Ctrl Pts',(-1.48999122658679,10.0484404115512,12.2047160013539));
#90839=CARTESIAN_POINT('Ctrl Pts',(-6.08217862707687,8.13623572102791,12.2834528146308));
#90840=CARTESIAN_POINT('Ctrl Pts',(-9.21589169840261,4.27300465283104,12.3621896279078));
#90841=CARTESIAN_POINT('Ctrl Pts',(-10.1396825877914,-0.614870375477425,
12.4409264411848));
#90842=CARTESIAN_POINT('Ctrl Pts',(-8.63203111632417,-5.35530273342346,
12.5196632544618));
#90843=CARTESIAN_POINT('Ctrl Pts',(-5.05446414851482,-8.81156176458976,
12.5984000677387));
#90844=CARTESIAN_POINT('Ctrl Pts',(-0.264863358569285,-10.1548547976369,
12.6771368810157));
#90845=CARTESIAN_POINT('Ctrl Pts',(4.58825026664382,-9.06306725399544,12.7558736942927));
#90846=CARTESIAN_POINT('Ctrl Pts',(8.34112569761994,-5.79800402348134,12.8346105075696));
#90847=CARTESIAN_POINT('Ctrl Pts',(10.0938432160754,-1.14261003369072,12.9133473208466));
#90848=CARTESIAN_POINT('Ctrl Pts',(9.42611041304279,3.78677581075619,12.9920841341236));
#90849=CARTESIAN_POINT('Ctrl Pts',(6.49804608997074,7.80811280479587,13.0708209474006));
#90850=CARTESIAN_POINT('Ctrl Pts',(2.0117846153455,9.95710556443289,13.1495577606775));
#90851=CARTESIAN_POINT('Ctrl Pts',(-2.95689219056041,9.71843696965745,13.2282945739545));
#90852=CARTESIAN_POINT('Ctrl Pts',(-7.2165218575283,7.14933848965189,13.3070313872315));
#90853=CARTESIAN_POINT('Ctrl Pts',(-9.74566767645484,2.8658663785852,13.3857682005084));
#90854=CARTESIAN_POINT('Ctrl Pts',(-9.93785383040227,-2.1048253622,13.4645050137854));
#90855=CARTESIAN_POINT('Ctrl Pts',(-7.74699509413485,-6.57079109173712,
13.5432418270624));
#90856=CARTESIAN_POINT('Ctrl Pts',(-3.69844782786315,-9.46111580229183,
13.6219786403394));
#90857=CARTESIAN_POINT('Ctrl Pts',(1.23696770476934,-10.0827148852459,13.7007154536163));
#90858=CARTESIAN_POINT('Ctrl Pts',(5.8757649113007,-8.28653216170243,13.7794522668933));
#90859=CARTESIAN_POINT('Ctrl Pts',(9.10558470812793,-4.5032827673719,13.8581890801703));
#90860=CARTESIAN_POINT('Ctrl Pts',(10.1519333570157,0.359830063382712,13.9369258934473));
#90861=CARTESIAN_POINT('Ctrl Pts',(8.76390197525464,5.13665754435015,14.0156627067242));
#90862=CARTESIAN_POINT('Ctrl Pts',(5.27433316127832,8.68174166072924,14.0943995200012));
#90863=CARTESIAN_POINT('Ctrl Pts',(0.520007096513734,10.1449899546218,14.1731363332782));
#90864=CARTESIAN_POINT('Ctrl Pts',(-4.35901392506651,9.1755232091079,14.2518731465552));
#90865=CARTESIAN_POINT('Ctrl Pts',(-8.19276641706479,6.00581443229949,14.3306099598321));
#90866=CARTESIAN_POINT('Ctrl Pts',(-10.0619367688849,1.39594305713547,14.4093467731091));
#90867=CARTESIAN_POINT('Ctrl Pts',(-9.51830779683059,-3.54866809445402,
14.4880835863861));
#90868=CARTESIAN_POINT('Ctrl Pts',(-6.69223885878102,-7.64232736912144,
14.566820399663));
#90869=CARTESIAN_POINT('Ctrl Pts',(-2.26140636829051,-9.90339688173995,
14.64555721294));
#90870=CARTESIAN_POINT('Ctrl Pts',(2.71169943217442,-9.78968409854713,14.724294026217));
#90871=CARTESIAN_POINT('Ctrl Pts',(7.03455402287886,-7.32845674470418,14.803030839494));
#90872=CARTESIAN_POINT('Ctrl Pts',(9.67055969174893,-3.1099041477387,14.881767652771));
#90873=CARTESIAN_POINT('Ctrl Pts',(9.98761619390468,1.8543870478017,14.9605044660479));
#90874=CARTESIAN_POINT('Ctrl Pts',(7.90969505375507,6.37400601791403,15.0392412793249));
#90875=CARTESIAN_POINT('Ctrl Pts',(3.93507079211811,9.36517199098984,15.1179780926019));
#90876=CARTESIAN_POINT('Ctrl Pts',(-0.983162673661375,10.1106191559627,
15.1967149058789));
#90877=CARTESIAN_POINT('Ctrl Pts',(-5.66563892005498,8.43159321761664,15.2754517191558));
#90878=CARTESIAN_POINT('Ctrl Pts',(-8.9895248602665,4.73071573299997,15.3541885324328));
#90879=CARTESIAN_POINT('Ctrl Pts',(-10.157770191418,-0.104562412662874,
15.4329253457097));
#90880=CARTESIAN_POINT('Ctrl Pts',(-8.89023584984156,-4.91476704371533,
15.5116621589867));
#90881=CARTESIAN_POINT('Ctrl Pts',(-5.49086987979438,-8.54643648095388,
15.5903989722637));
#90882=CARTESIAN_POINT('Ctrl Pts',(-0.774822296877582,-10.1287155635864,
15.6691357855407));
#90883=CARTESIAN_POINT('Ctrl Pts',(4.12702358282595,-9.28218211988161,15.7478725988177));
#90884=CARTESIAN_POINT('Ctrl Pts',(8.039230992423,-6.20983040108157,15.8266094120946));
#90885=CARTESIAN_POINT('Ctrl Pts',(10.0236732462154,-1.64839413155914,15.9053462253716));
#90886=CARTESIAN_POINT('Ctrl Pts',(9.60449156688632,3.30831834947895,15.9840830386486));
#90887=CARTESIAN_POINT('Ctrl Pts',(6.88220350844336,7.47171355364201,16.0628198519255));
#90888=CARTESIAN_POINT('Ctrl Pts',(2.50959937730913,9.84343128825342,16.1415566652025));
#90889=CARTESIAN_POINT('Ctrl Pts',(-2.46479343721129,9.85474615953707,16.2202934784795));
#90890=CARTESIAN_POINT('Ctrl Pts',(-6.84814179629524,7.50294492196215,16.2990302917565));
#90891=CARTESIAN_POINT('Ctrl Pts',(-9.58934190136322,3.35197709629649,16.3777671050334));
#90892=CARTESIAN_POINT('Ctrl Pts',(-10.0310684373532,-1.60277714101786,
16.4565039183104));
#90893=CARTESIAN_POINT('Ctrl Pts',(-8.06739771199873,-6.17319388461373,
16.5352407315874));
#90894=CARTESIAN_POINT('Ctrl Pts',(-4.16920760099691,-9.26331131253746,
16.6139775448644));
#90895=CARTESIAN_POINT('Ctrl Pts',(0.728736486607317,-10.1321356012481,
16.6927143581413));
#90896=CARTESIAN_POINT('Ctrl Pts',(5.45193340832726,-8.5713272258263,16.7714511714183));
#90897=CARTESIAN_POINT('Ctrl Pts',(8.8677854835772,-4.95515988634399,16.8501879846953));
#90898=CARTESIAN_POINT('Ctrl Pts',(10.1571893978969,-0.150771246642594,
16.9289247979723));
#90899=CARTESIAN_POINT('Ctrl Pts',(9.01095293356691,4.68977131717587,17.0076616112492));
#90900=CARTESIAN_POINT('Ctrl Pts',(5.7039374769669,8.40573191115353,17.0863984245262));
#90901=CARTESIAN_POINT('Ctrl Pts',(1.02914800842723,10.1060415169882,17.1651352378032));
#90902=CARTESIAN_POINT('Ctrl Pts',(-3.89242588692388,9.38297735565258,17.2438720510802));
#90903=CARTESIAN_POINT('Ctrl Pts',(-7.88061627753002,6.40992156736009,17.3226088643571));
#90904=CARTESIAN_POINT('Ctrl Pts',(-9.9790771117823,1.89980660441441,17.4013456776341));
#90905=CARTESIAN_POINT('Ctrl Pts',(-9.684606712062,-3.06588394600143,17.4800824909111));
#90906=CARTESIAN_POINT('Ctrl Pts',(-7.06782110814213,-7.29636844528527,
17.5588193041881));
#90907=CARTESIAN_POINT('Ctrl Pts',(-2.75620472519069,-9.77726743968932,
17.637556117465));
#90908=CARTESIAN_POINT('Ctrl Pts',(2.21632610604956,-9.91354174907297,17.716292930742));
#90909=CARTESIAN_POINT('Ctrl Pts',(6.65741088915815,-7.67277100430263,17.795029744019));
#90910=CARTESIAN_POINT('Ctrl Pts',(9.50205026076092,-3.59178006489433,17.8737665572959));
#90911=CARTESIAN_POINT('Ctrl Pts',(10.0682124959338,1.34985463701419,17.9525033705729));
#90912=CARTESIAN_POINT('Ctrl Pts',(8.21995047085605,5.96911019038295,18.0312401838499));
#90913=CARTESIAN_POINT('Ctrl Pts',(5.67383374951871,8.09231563285626,18.0837313927012));
#90914=CARTESIAN_POINT('Ctrl Pts',(4.22448187184914,8.7889580239625,18.1099769971269));
#90915=CARTESIAN_POINT('Ctrl Pts',(5.54986643234452,-7.78462448629111,3.89019495060166));
#90916=CARTESIAN_POINT('Ctrl Pts',(6.83388415871134,-6.86921802277418,3.91644636730371));
#90917=CARTESIAN_POINT('Ctrl Pts',(8.93886599082429,-4.39215922307585,3.96894338843142));
#90918=CARTESIAN_POINT('Ctrl Pts',(9.95198094471023,0.379631740305084,4.04768601398477));
#90919=CARTESIAN_POINT('Ctrl Pts',(8.57869151975529,5.05875230468204,4.12642282726174));
#90920=CARTESIAN_POINT('Ctrl Pts',(5.14823127529553,8.52544572373377,4.20515964053872));
#90921=CARTESIAN_POINT('Ctrl Pts',(0.48327527821911,9.94745767769539,4.28389645381569));
#90922=CARTESIAN_POINT('Ctrl Pts',(-4.29757932840324,8.9842888304963,4.36263326709267));
#90923=CARTESIAN_POINT('Ctrl Pts',(-8.04789104842608,5.86664886935661,4.44137008036965));
#90924=CARTESIAN_POINT('Ctrl Pts',(-9.86836409428141,1.34226184460021,4.52010689364661));
#90925=CARTESIAN_POINT('Ctrl Pts',(-9.32245391500608,-3.50401535487271,
4.59884370692359));
#90926=CARTESIAN_POINT('Ctrl Pts',(-6.54106932501662,-7.51003638009355,
4.67758052020056));
#90927=CARTESIAN_POINT('Ctrl Pts',(-2.1911704118723,-9.71519640075353,4.75631733347753));
#90928=CARTESIAN_POINT('Ctrl Pts',(2.6841593795726,-9.59070047518796,4.83505414675451));
#90929=CARTESIAN_POINT('Ctrl Pts',(6.9158420339386,-7.16640681609978,4.91379096003148));
#90930=CARTESIAN_POINT('Ctrl Pts',(9.48914221630516,-3.02364579908635,4.99252777330845));
#90931=CARTESIAN_POINT('Ctrl Pts',(9.7869962150742,1.84416909080794,5.07126458658543));
#90932=CARTESIAN_POINT('Ctrl Pts',(7.73798016792419,6.26976218856729,5.15000139986241));
#90933=CARTESIAN_POINT('Ctrl Pts',(3.83343733049769,9.19189929531005,5.22873821313939));
#90934=CARTESIAN_POINT('Ctrl Pts',(-0.990343547589242,9.90986753048978,
5.30747502641634));
#90935=CARTESIAN_POINT('Ctrl Pts',(-5.5766452684996,8.25150181215553,5.38621183969333));
#90936=CARTESIAN_POINT('Ctrl Pts',(-8.82569689220261,4.61446953155593,5.46494865297029));
#90937=CARTESIAN_POINT('Ctrl Pts',(-9.95839298823366,-0.12908819265254,
5.54368546624728));
#90938=CARTESIAN_POINT('Ctrl Pts',(-8.70311901271208,-4.84169124552408,
5.62242227952423));
#90939=CARTESIAN_POINT('Ctrl Pts',(-5.36088303839152,-8.39328229738432,
5.70115909280123));
#90940=CARTESIAN_POINT('Ctrl Pts',(-0.73313560969372,-9.93220855831381,
5.77989590607818));
#90941=CARTESIAN_POINT('Ctrl Pts',(4.07041386829234,-9.08944363604411,5.85863271935516));
#90942=CARTESIAN_POINT('Ctrl Pts',(7.89789958687557,-6.06707810942492,5.93736953263214));
#90943=CARTESIAN_POINT('Ctrl Pts',(9.83151067467579,-1.58985927821512,6.0161063459091));
#90944=CARTESIAN_POINT('Ctrl Pts',(9.40757739965206,3.26859941569965,6.0948431591861));
#90945=CARTESIAN_POINT('Ctrl Pts',(6.72775672337378,7.34326522343693,6.17357997246305));
#90946=CARTESIAN_POINT('Ctrl Pts',(2.4346554982096,9.6570547930408,6.25231678574004));
#90947=CARTESIAN_POINT('Ctrl Pts',(-2.44226326376367,9.65513359934245,6.331053599017));
#90948=CARTESIAN_POINT('Ctrl Pts',(-6.73354018690624,7.33796233446559,6.40979041229398));
#90949=CARTESIAN_POINT('Ctrl Pts',(-9.41014971713789,3.26118643621514,6.48852722557094));
#90950=CARTESIAN_POINT('Ctrl Pts',(-9.83025501795751,-1.59760475482128,
6.56726403884793));
#90951=CARTESIAN_POINT('Ctrl Pts',(-7.89311705581146,-6.07329875882669,
6.64600085212489));
#90952=CARTESIAN_POINT('Ctrl Pts',(-4.06325128857577,-9.09264777920014,
6.72473766540188));
#90953=CARTESIAN_POINT('Ctrl Pts',(0.740960689234815,-9.93162785890187,
6.80347447867885));
#90954=CARTESIAN_POINT('Ctrl Pts',(5.36749420502885,-8.3890560034898,6.88221129195582));
#90955=CARTESIAN_POINT('Ctrl Pts',(8.70693094350651,-4.83483280121613,6.9609481052328));
#90956=CARTESIAN_POINT('Ctrl Pts',(9.95849160245273,-0.121242214534584,
7.03968491850977));
#90957=CARTESIAN_POINT('Ctrl Pts',(8.82205854238565,4.62142161519883,7.11842173178673));
#90958=CARTESIAN_POINT('Ctrl Pts',(5.57014241229265,8.25589293641125,7.19715854506373));
#90959=CARTESIAN_POINT('Ctrl Pts',(0.982535534487584,9.91064471132812,7.27589535834069));
#90960=CARTESIAN_POINT('Ctrl Pts',(-3.84067817803991,9.18887619915703,7.35463217161766));
#90961=CARTESIAN_POINT('Ctrl Pts',(-7.74291753701654,6.26366367916321,7.43336898489463));
#90962=CARTESIAN_POINT('Ctrl Pts',(-9.78844614266187,1.83645767250828,7.51210579817161));
#90963=CARTESIAN_POINT('Ctrl Pts',(-9.48675703294365,-3.03112119002206,
7.59084261144859));
#90964=CARTESIAN_POINT('Ctrl Pts',(-6.91019366386524,-7.17185319137134,
7.66957942472556));
#90965=CARTESIAN_POINT('Ctrl Pts',(-2.67660233059081,-9.5928126550341,7.74831623800253));
#90966=CARTESIAN_POINT('Ctrl Pts',(2.19882411274918,-9.71346628098845,7.8270530512795));
#90967=CARTESIAN_POINT('Ctrl Pts',(6.54698414064464,-7.50488196661709,7.90578986455649));
#90968=CARTESIAN_POINT('Ctrl Pts',(9.32521193076139,-3.49666657219303,7.98452667783345));
#90969=CARTESIAN_POINT('Ctrl Pts',(9.86730312428339,1.35003100861192,8.06326349111042));
#90970=CARTESIAN_POINT('Ctrl Pts',(8.04326711450635,5.87299827987438,8.14200030438739));
#90971=CARTESIAN_POINT('Ctrl Pts',(4.29049810815211,8.98765156504466,8.22073711766438));
#90972=CARTESIAN_POINT('Ctrl Pts',(-0.491109696558105,9.94711344746069,
8.29947393094134));
#90973=CARTESIAN_POINT('Ctrl Pts',(-5.15495198842312,8.52131003236937,8.37821074421831));
#90974=CARTESIAN_POINT('Ctrl Pts',(-8.58266400458077,5.05214145241206,8.4569475574953));
#90975=CARTESIAN_POINT('Ctrl Pts',(-9.95229849720142,0.371496020583359,
8.53568437077227));
#90976=CARTESIAN_POINT('Ctrl Pts',(-8.93542434475686,-4.39823219598886,
8.61442118404923));
#90977=CARTESIAN_POINT('Ctrl Pts',(-5.7758826012946,-8.11328754863087,8.69315799732622));
#90978=CARTESIAN_POINT('Ctrl Pts',(-1.23131469882525,-9.88281937420509,
8.77189481060318));
#90979=CARTESIAN_POINT('Ctrl Pts',(3.60851596876001,-9.28250328165365,8.85063162388015));
#90980=CARTESIAN_POINT('Ctrl Pts',(7.58304355507985,-6.45629190112006,8.92936843715714));
#90981=CARTESIAN_POINT('Ctrl Pts',(9.73919732502021,-2.08189580311446,9.0081052504341));
#90982=CARTESIAN_POINT('Ctrl Pts',(9.55994298610092,2.79172791890731,9.08684206371107));
#90983=CARTESIAN_POINT('Ctrl Pts',(7.08826478257631,6.99591002249136,9.16557887698806));
#90984=CARTESIAN_POINT('Ctrl Pts',(2.91685810056142,9.52250983154629,9.24431569026502));
#90985=CARTESIAN_POINT('Ctrl Pts',(-1.95399575693514,9.76566204886213,9.32305250354201));
#90986=CARTESIAN_POINT('Ctrl Pts',(-6.35629174635151,7.66706005623865,9.40178931681896));
#90987=CARTESIAN_POINT('Ctrl Pts',(-9.23438252754493,3.72993753375037,9.48052613009595));
#90988=CARTESIAN_POINT('Ctrl Pts',(-9.8981171235795,-1.10160432034774,9.55926294337291));
#90989=CARTESIAN_POINT('Ctrl Pts',(-8.1883354819397,-5.66898727339496,9.6379997566499));
#90990=CARTESIAN_POINT('Ctrl Pts',(-4.51503421497537,-8.87697700280384,
9.71673656992686));
#90991=CARTESIAN_POINT('Ctrl Pts',(0.240948423516744,-9.95631450527311,
9.79547338320386));
#90992=CARTESIAN_POINT('Ctrl Pts',(4.93915290192862,-8.64818034514063,9.87421019648081));
#90993=CARTESIAN_POINT('Ctrl Pts',(8.45297458644962,-5.26625818884181,9.9529470097578));
#90994=CARTESIAN_POINT('Ctrl Pts',(9.93981758531818,-0.621515117520195,
10.0316838230348));
#90995=CARTESIAN_POINT('Ctrl Pts',(9.04314479590899,4.17226399823058,10.1104206363118));
#90996=CARTESIAN_POINT('Ctrl Pts',(5.97797361991285,7.96555623106965,10.1891574495887));
#90997=CARTESIAN_POINT('Ctrl Pts',(1.47931592540995,9.84875012697221,10.2678942628657));
#90998=CARTESIAN_POINT('Ctrl Pts',(-3.37407391923556,9.37026573039639,10.3466310761427));
#90999=CARTESIAN_POINT('Ctrl Pts',(-7.41837864855737,6.64484107389598,10.4253678894196));
#91000=CARTESIAN_POINT('Ctrl Pts',(-9.68379533687761,2.32601860357435,10.5041047026966));
#91001=CARTESIAN_POINT('Ctrl Pts',(-9.62708902064784,-2.55057084967824,
10.5828415159736));
#91002=CARTESIAN_POINT('Ctrl Pts',(-7.26185757516794,-6.81554687671376,
10.6615783292506));
#91003=CARTESIAN_POINT('Ctrl Pts',(-3.15527101586746,-9.44619073950626,
10.7403151425275));
#91004=CARTESIAN_POINT('Ctrl Pts',(1.70793287751002,-9.81168792597006,10.8190519558045));
#91005=CARTESIAN_POINT('Ctrl Pts',(6.16158348241702,-7.82439414011797,10.8977887690815));
#91006=CARTESIAN_POINT('Ctrl Pts',(9.1377188929984,-3.96085194159623,10.9765255823584));
#91007=CARTESIAN_POINT('Ctrl Pts',(9.92267754773311,0.852481644623632,11.0552623956354));
#91008=CARTESIAN_POINT('Ctrl Pts',(8.32823050472688,5.46139463240326,11.1339992089124));
#91009=CARTESIAN_POINT('Ctrl Pts',(4.73671774838673,8.76069401604832,11.2127360221894));
#91010=CARTESIAN_POINT('Ctrl Pts',(0.00936507939353068,9.9592252191621,
11.2914728354663));
#91011=CARTESIAN_POINT('Ctrl Pts',(-4.72023328620338,8.76958678584825,11.3702096487433));
#91012=CARTESIAN_POINT('Ctrl Pts',(-8.31794462616336,5.4770477327468,11.4489464620203));
#91013=CARTESIAN_POINT('Ctrl Pts',(-9.92105675217349,0.87114154467542,11.5276832752972));
#91014=CARTESIAN_POINT('Ctrl Pts',(-9.14515183866235,-3.94365978736978,
11.6064200885743));
#91015=CARTESIAN_POINT('Ctrl Pts',(-6.17628778817008,-7.81279231954925,
11.6851569018512));
#91016=CARTESIAN_POINT('Ctrl Pts',(-1.72638252845134,-9.80845849438966,
11.7638937151282));
#91017=CARTESIAN_POINT('Ctrl Pts',(3.13750014864465,-9.45210809756012,11.8426305284052));
#91018=CARTESIAN_POINT('Ctrl Pts',(7.24902685181769,-6.8291920731762,11.9213673416821));
#91019=CARTESIAN_POINT('Ctrl Pts',(9.62227518090085,-2.56867183846557,12.0001041549591));
#91020=CARTESIAN_POINT('Ctrl Pts',(9.68815271409469,2.30780234402479,12.0788409682361));
#91021=CARTESIAN_POINT('Ctrl Pts',(7.43086236668286,6.63087770646717,12.1575777815131));
#91022=CARTESIAN_POINT('Ctrl Pts',(3.39169044855997,9.36390359689024,12.23631459479));
#91023=CARTESIAN_POINT('Ctrl Pts',(-1.46079093562736,9.85151483342006,12.315051408067));
#91024=CARTESIAN_POINT('Ctrl Pts',(-5.96298236443524,7.97678481545922,12.393788221344));
#91025=CARTESIAN_POINT('Ctrl Pts',(-9.03528209866653,4.18926390529685,12.472525034621));
#91026=CARTESIAN_POINT('Ctrl Pts',(-9.94096887960528,-0.602820375755343,
12.5512618478979));
#91027=CARTESIAN_POINT('Ctrl Pts',(-8.46286379797352,-5.25035151277091,
12.6299986611749));
#91028=CARTESIAN_POINT('Ctrl Pts',(-4.95540864996746,-8.63887607171988,
12.7087354744519));
#91029=CARTESIAN_POINT('Ctrl Pts',(-0.259672665498926,-9.95584375015496,
12.7874722877288));
#91030=CARTESIAN_POINT('Ctrl Pts',(4.49833145343869,-8.88545265058065,12.8662091010058));
#91031=CARTESIAN_POINT('Ctrl Pts',(8.17765943489719,-5.6843769084697,12.9449459142828));
#91032=CARTESIAN_POINT('Ctrl Pts',(9.89602785075699,-1.12021758946579,13.0236827275598));
#91033=CARTESIAN_POINT('Ctrl Pts',(9.24138102553675,3.71256399427083,13.1024195408367));
#91034=CARTESIAN_POINT('Ctrl Pts',(6.37069981228177,7.65509232945621,13.1811563541137));
#91035=CARTESIAN_POINT('Ctrl Pts',(1.9723584126487,9.761969932486,13.2598931673907));
#91036=CARTESIAN_POINT('Ctrl Pts',(-2.89894412297489,9.5279786755941,13.3386299806676));
#91037=CARTESIAN_POINT('Ctrl Pts',(-7.07509516038074,7.00922842702848,13.4173667939446));
#91038=CARTESIAN_POINT('Ctrl Pts',(-9.55467572518108,2.80970220082872,13.4961036072216));
#91039=CARTESIAN_POINT('Ctrl Pts',(-9.74309548674077,-2.06357578173378,
13.5748404204986));
#91040=CARTESIAN_POINT('Ctrl Pts',(-7.59517238083715,-6.44201918470249,
13.6535772337755));
#91041=CARTESIAN_POINT('Ctrl Pts',(-3.62596703016116,-9.27570039225563,
13.7323140470525));
#91042=CARTESIAN_POINT('Ctrl Pts',(1.21272607418644,-9.88511760879428,13.8110508603295));
#91043=CARTESIAN_POINT('Ctrl Pts',(5.76061386748395,-8.12413580268438,13.8897876736065));
#91044=CARTESIAN_POINT('Ctrl Pts',(8.9271368635441,-4.41502911544861,13.9685244868834));
#91045=CARTESIAN_POINT('Ctrl Pts',(9.95297956283469,0.352778248338951,14.0472613001604));
#91046=CARTESIAN_POINT('Ctrl Pts',(8.59215030111643,5.03599125036287,14.1259981134374));
#91047=CARTESIAN_POINT('Ctrl Pts',(5.17096875202658,8.51160013371584,14.2047349267144));
#91048=CARTESIAN_POINT('Ctrl Pts',(0.509816191863926,9.94617223464483,14.2834717399913));
#91049=CARTESIAN_POINT('Ctrl Pts',(-4.27358759997346,8.99570473593146,14.3622085532683));
#91050=CARTESIAN_POINT('Ctrl Pts',(-8.0322076440517,5.88811472659494,14.4409453665453));
#91051=CARTESIAN_POINT('Ctrl Pts',(-9.86474669418887,1.36858588703684,14.5196821798223));
#91052=CARTESIAN_POINT('Ctrl Pts',(-9.33177155946915,-3.47912262396562,
14.5984189930992));
#91053=CARTESIAN_POINT('Ctrl Pts',(-6.56108686381646,-7.49255589476393,
14.6771558063762));
#91054=CARTESIAN_POINT('Ctrl Pts',(-2.21708817181164,-9.70931381247509,
14.7558926196532));
#91055=CARTESIAN_POINT('Ctrl Pts',(2.65855656059159,-9.59782952989072,14.8346294329302));
#91056=CARTESIAN_POINT('Ctrl Pts',(6.89669346331803,-7.18483638948953,14.9133662462071));
#91057=CARTESIAN_POINT('Ctrl Pts',(9.48103967867699,-3.04895740902669,14.9921030594841));
#91058=CARTESIAN_POINT('Ctrl Pts',(9.79188262604912,1.81804546378362,15.0708398727611));
#91059=CARTESIAN_POINT('Ctrl Pts',(7.75468380748131,6.24909063117937,15.1495766860381));
#91060=CARTESIAN_POINT('Ctrl Pts',(3.85795274603463,9.18163685189467,15.228313499315));
#91061=CARTESIAN_POINT('Ctrl Pts',(-0.963895019181878,9.91247502204688,
15.307050312592));
#91062=CARTESIAN_POINT('Ctrl Pts',(-5.55460584684975,8.26635400626227,15.385787125869));
#91063=CARTESIAN_POINT('Ctrl Pts',(-8.81335151318695,4.63800493485218,15.464523939146));
#91064=CARTESIAN_POINT('Ctrl Pts',(-9.95870200913874,-0.102513237594813,
15.5432607524229));
#91065=CARTESIAN_POINT('Ctrl Pts',(-8.71600833166472,-4.81844927679591,
15.6219975656999));
#91066=CARTESIAN_POINT('Ctrl Pts',(-5.38326186489501,-8.37894661426389,
15.7007343789769));
#91067=CARTESIAN_POINT('Ctrl Pts',(-0.759637619204987,-9.93021678304004,
15.7794711922538));
#91068=CARTESIAN_POINT('Ctrl Pts',(4.04614371772026,-9.10027338525098,15.8582080055308));
#91069=CARTESIAN_POINT('Ctrl Pts',(7.881681149256,-6.08813246670124,15.9369448188078));
#91070=CARTESIAN_POINT('Ctrl Pts',(9.82723304573019,-1.61608951969397,16.0156816320848));
#91071=CARTESIAN_POINT('Ctrl Pts',(9.41626633222295,3.24348316342719,16.0944184453617));
#91072=CARTESIAN_POINT('Ctrl Pts',(6.74732865730142,7.32528570504871,16.1731552586387));
#91073=CARTESIAN_POINT('Ctrl Pts',(2.46041718703747,9.65052340226892,16.2518920719157));
#91074=CARTESIAN_POINT('Ctrl Pts',(-2.41648933700102,9.66161652893571,16.3306288851926));
#91075=CARTESIAN_POINT('Ctrl Pts',(-6.71393447385249,7.35590501268973,16.4093656984696));
#91076=CARTESIAN_POINT('Ctrl Pts',(-9.40141356418044,3.28628630244833,16.4881025117466));
#91077=CARTESIAN_POINT('Ctrl Pts',(-9.83448330867708,-1.57136651387741,
16.5668393250236));
#91078=CARTESIAN_POINT('Ctrl Pts',(-7.90929586799285,-6.05221393898498,
16.6455761383005));
#91079=CARTESIAN_POINT('Ctrl Pts',(-4.08750102927544,-9.0817724009335,16.7243129515775));
#91080=CARTESIAN_POINT('Ctrl Pts',(0.714454981413205,-9.93356979608242,
16.8030497648545));
#91081=CARTESIAN_POINT('Ctrl Pts',(5.3450884558376,-8.40334955962479,16.8817865781315));
#91082=CARTESIAN_POINT('Ctrl Pts',(8.69399793928435,-4.85805051559736,16.9605233914084));
#91083=CARTESIAN_POINT('Ctrl Pts',(9.95813259779199,-0.147816488123383,
17.0392602046854));
#91084=CARTESIAN_POINT('Ctrl Pts',(8.83435964711863,4.59786293238055,17.1179970179624));
#91085=CARTESIAN_POINT('Ctrl Pts',(5.5921538429629,8.24099952001386,17.1967338312394));
#91086=CARTESIAN_POINT('Ctrl Pts',(1.00897915055061,9.90798709392943,17.2754706445163));
#91087=CARTESIAN_POINT('Ctrl Pts',(-3.81614357974774,9.19909327367808,17.3542074577933));
#91088=CARTESIAN_POINT('Ctrl Pts',(-7.72617490624037,6.28430232111598,17.4329442710703));
#91089=CARTESIAN_POINT('Ctrl Pts',(-9.78351088966547,1.8625749049079,17.5116810843473));
#91090=CARTESIAN_POINT('Ctrl Pts',(-9.49481141073808,-3.00579989874418,
17.5904178976242));
#91091=CARTESIAN_POINT('Ctrl Pts',(-6.92930859268264,-7.15337694456503,
17.6691547109012));
#91092=CARTESIAN_POINT('Ctrl Pts',(-2.70218965551557,-9.58565620807068,
17.7478915241782));
#91093=CARTESIAN_POINT('Ctrl Pts',(2.17289137569487,-9.71925986449121,17.8266283374551));
#91094=CARTESIAN_POINT('Ctrl Pts',(6.52694143972031,-7.52240290696552,17.9053651507321));
#91095=CARTESIAN_POINT('Ctrl Pts',(9.31583263251279,-3.52138970212855,17.9841019640091));
#91096=CARTESIAN_POINT('Ctrl Pts',(9.87089943188555,1.32340069054093,18.0628387772861));
#91097=CARTESIAN_POINT('Ctrl Pts',(8.05885895492069,5.85212980068802,18.141575590563));
#91098=CARTESIAN_POINT('Ctrl Pts',(5.56264007710963,7.93372545675409,18.1940667994144));
#91099=CARTESIAN_POINT('Ctrl Pts',(4.14169205563424,8.61671531075004,18.22031240384));
#91100=CARTESIAN_POINT('Ctrl Pts',(5.43892809705089,-7.62901474470127,4.00053035731484));
#91101=CARTESIAN_POINT('Ctrl Pts',(6.69727911759927,-6.7319066799688,4.02678177401689));
#91102=CARTESIAN_POINT('Ctrl Pts',(8.76018368837185,-4.30436272590017,4.07927879514459));
#91103=CARTESIAN_POINT('Ctrl Pts',(9.75304711227676,0.372043140866268,4.15802142069795));
#91104=CARTESIAN_POINT('Ctrl Pts',(8.40720887818163,4.9576310315513,4.23675823397493));
#91105=CARTESIAN_POINT('Ctrl Pts',(5.04532137388612,8.35502743209433,4.3154950472519));
#91106=CARTESIAN_POINT('Ctrl Pts',(0.473614909720539,9.7486142625213,4.39423186052886));
#91107=CARTESIAN_POINT('Ctrl Pts',(-4.21167342376619,8.80469855408104,4.47296867380585));
#91108=CARTESIAN_POINT('Ctrl Pts',(-7.8870187740352,5.74937825262146,4.55170548708282));
#91109=CARTESIAN_POINT('Ctrl Pts',(-9.67110171003543,1.31543087553393,4.6304423003598));
#91110=CARTESIAN_POINT('Ctrl Pts',(-9.13610393149024,-3.43397229436816,
4.70917911363676));
#91111=CARTESIAN_POINT('Ctrl Pts',(-6.41031746804786,-7.35991548184156,
4.78791592691374));
#91112=CARTESIAN_POINT('Ctrl Pts',(-2.14737029509449,-9.52099574225318,
4.86665274019072));
#91113=CARTESIAN_POINT('Ctrl Pts',(2.63050472376014,-9.39898841184597,4.94538955346768));
#91114=CARTESIAN_POINT('Ctrl Pts',(6.7775987065087,-7.02315485645229,5.02412636674467));
#91115=CARTESIAN_POINT('Ctrl Pts',(9.29946023860813,-2.96320502351861,5.10286318002163));
#91116=CARTESIAN_POINT('Ctrl Pts',(9.59136032349711,1.80730531193538,5.18159999329862));
#91117=CARTESIAN_POINT('Ctrl Pts',(7.5833028168871,6.14443359041709,5.26033680657558));
#91118=CARTESIAN_POINT('Ctrl Pts',(3.75680933213372,9.00815901643317,5.33907361985255));
#91119=CARTESIAN_POINT('Ctrl Pts',(-0.970547203681225,9.71177551868821,
5.41781043312952));
#91120=CARTESIAN_POINT('Ctrl Pts',(-5.46517164113355,8.08655948680911,5.4965472464065));
#91121=CARTESIAN_POINT('Ctrl Pts',(-8.64927676877029,4.52222919130004,5.57528405968347));
#91122=CARTESIAN_POINT('Ctrl Pts',(-9.75933098308775,-0.126507800966816,
5.65402087296046));
#91123=CARTESIAN_POINT('Ctrl Pts',(-8.52914914390484,-4.74490888628499,
5.73275768623743));
#91124=CARTESIAN_POINT('Ctrl Pts',(-5.25372236214226,-8.22550586941576,
5.81149449951439));
#91125=CARTESIAN_POINT('Ctrl Pts',(-0.718480690503233,-9.73366996343397,
5.89023131279138));
#91126=CARTESIAN_POINT('Ctrl Pts',(3.98904885815936,-8.90775138128075,5.96896812606833));
#91127=CARTESIAN_POINT('Ctrl Pts',(7.74002554735313,-5.94580103838886,6.04770493934533));
#91128=CARTESIAN_POINT('Ctrl Pts',(9.63498496708154,-1.55807899236021,6.12644175262228));
#91129=CARTESIAN_POINT('Ctrl Pts',(9.21952585127947,3.20326217158038,6.20517856589926));
#91130=CARTESIAN_POINT('Ctrl Pts',(6.5932731028668,7.19647797559256,6.28391537917623));
#91131=CARTESIAN_POINT('Ctrl Pts',(2.38598826787577,9.4640163486675,6.36265219245321));
#91132=CARTESIAN_POINT('Ctrl Pts',(-2.39344395898697,9.46213355842142,6.44138900573019));
#91133=CARTESIAN_POINT('Ctrl Pts',(-6.59894095860507,7.19128108803257,6.52012581900716));
#91134=CARTESIAN_POINT('Ctrl Pts',(-9.22204674975853,3.19599737288787,6.59886263228413));
#91135=CARTESIAN_POINT('Ctrl Pts',(-9.63375441015036,-1.5656696417663,6.67759944556111));
#91136=CARTESIAN_POINT('Ctrl Pts',(-7.73533861607347,-5.95189734092617,
6.75633625883808));
#91137=CARTESIAN_POINT('Ctrl Pts',(-3.98202945390109,-8.91089147563272,
6.83507307211505));
#91138=CARTESIAN_POINT('Ctrl Pts',(0.726149351631704,-9.7331008718376,6.91380988539203));
#91139=CARTESIAN_POINT('Ctrl Pts',(5.2602013757215,-8.22136405647494,6.99254669866899));
#91140=CARTESIAN_POINT('Ctrl Pts',(8.53288487660304,-4.73818753796005,7.07128351194597));
#91141=CARTESIAN_POINT('Ctrl Pts',(9.75942762607066,-0.118818659010883,
7.15002032522295));
#91142=CARTESIAN_POINT('Ctrl Pts',(8.64571114727513,4.5290423071686,7.22875713849992));
#91143=CARTESIAN_POINT('Ctrl Pts',(5.45879877292739,8.09086283525602,7.30749395177689));
#91144=CARTESIAN_POINT('Ctrl Pts',(0.962895267844818,9.71253716417098,7.38623076505386));
#91145=CARTESIAN_POINT('Ctrl Pts',(-3.76390543969308,9.00519635006864,7.46496757833085));
#91146=CARTESIAN_POINT('Ctrl Pts',(-7.58814149108033,6.13845698637581,7.54370439160781));
#91147=CARTESIAN_POINT('Ctrl Pts',(-9.5927812679453,1.79974804003172,7.62244120488479));
#91148=CARTESIAN_POINT('Ctrl Pts',(-9.2971227335601,-2.9705309860967,7.70117801816176));
#91149=CARTESIAN_POINT('Ctrl Pts',(-6.77206324379635,-7.02849236211172,
7.77991483143874));
#91150=CARTESIAN_POINT('Ctrl Pts',(-2.62309873542888,-9.40105837054699,
7.85865164471571));
#91151=CARTESIAN_POINT('Ctrl Pts',(2.15487100331034,-9.51930020649275,7.93738845799269));
#91152=CARTESIAN_POINT('Ctrl Pts',(6.41611405023598,-7.35486410184478,8.01612527126965));
#91153=CARTESIAN_POINT('Ctrl Pts',(9.13880681624731,-3.42677040922677,8.09486208454663));
#91154=CARTESIAN_POINT('Ctrl Pts',(9.67006194815957,1.32304473884924,8.1735988978236));
#91155=CARTESIAN_POINT('Ctrl Pts',(7.88248726964285,5.75560074242115,8.25233571110058));
#91156=CARTESIAN_POINT('Ctrl Pts',(4.20473375264889,8.80799406968328,8.33107252437755));
#91157=CARTESIAN_POINT('Ctrl Pts',(-0.481292722970219,9.74827691323223,
8.40980933765452));
#91158=CARTESIAN_POINT('Ctrl Pts',(-5.05190774419027,8.35097441059609,8.48854615093149));
#91159=CARTESIAN_POINT('Ctrl Pts',(-8.4111019555369,4.95115232605539,8.56728296420848));
#91160=CARTESIAN_POINT('Ctrl Pts',(-9.75335831709361,0.364070049058778,
8.64601977748544));
#91161=CARTESIAN_POINT('Ctrl Pts',(-8.75681083864211,-4.31031430390876,
8.72475659076242));
#91162=CARTESIAN_POINT('Ctrl Pts',(-5.6604263451035,-7.95110803938034,8.80349340403939));
#91163=CARTESIAN_POINT('Ctrl Pts',(-1.20670149334083,-9.68526803801576,
8.88223021731637));
#91164=CARTESIAN_POINT('Ctrl Pts',(3.53638400678673,-9.09695188614206,8.96096703059333));
#91165=CARTESIAN_POINT('Ctrl Pts',(7.43146328937169,-6.3272346914716,9.03970384387032));
#91166=CARTESIAN_POINT('Ctrl Pts',(9.54451690315688,-2.04028001695672,9.11844065714729));
#91167=CARTESIAN_POINT('Ctrl Pts',(9.36884574559812,2.73592303572826,9.19717747042426));
#91168=CARTESIAN_POINT('Ctrl Pts',(6.94657483297379,6.8560661863882,9.27591428370123));
#91169=CARTESIAN_POINT('Ctrl Pts',(2.85855194384417,9.33216085623181,9.35465109697821));
#91170=CARTESIAN_POINT('Ctrl Pts',(-1.91493661216333,9.57045261383372,9.43338791025518));
#91171=CARTESIAN_POINT('Ctrl Pts',(-6.2292334768279,7.51380035357655,9.51212472353215));
#91172=CARTESIAN_POINT('Ctrl Pts',(-9.04979303560688,3.65537843115071,9.59086153680913));
#91173=CARTESIAN_POINT('Ctrl Pts',(-9.70025999501298,-1.07958394365195,
9.6695983500861));
#91174=CARTESIAN_POINT('Ctrl Pts',(-8.02465581175916,-5.55566778749779,
9.74833516336308));
#91175=CARTESIAN_POINT('Ctrl Pts',(-4.42478152408464,-8.69953182225111,
9.82707197664002));
#91176=CARTESIAN_POINT('Ctrl Pts',(0.236132016253185,-9.75729404769278,
9.90580878991702));
#91177=CARTESIAN_POINT('Ctrl Pts',(4.84042234554853,-8.47530866570387,9.98454560319398));
#91178=CARTESIAN_POINT('Ctrl Pts',(8.28400494721021,-5.16098900375083,10.063282416471));
#91179=CARTESIAN_POINT('Ctrl Pts',(9.74112689077983,-0.609091421682083,
10.1420192297479));
#91180=CARTESIAN_POINT('Ctrl Pts',(8.86237802580607,4.08886306813402,10.2207560430249));
#91181=CARTESIAN_POINT('Ctrl Pts',(5.85847769151402,7.80632977783241,10.2994928563019));
#91182=CARTESIAN_POINT('Ctrl Pts',(1.44974533156971,9.65187981358203,10.3782296695789));
#91183=CARTESIAN_POINT('Ctrl Pts',(-3.30662830620673,9.18296001879747,10.4569664828558));
#91184=CARTESIAN_POINT('Ctrl Pts',(-7.27008993064292,6.51201488501103,10.5357032961328));
#91185=CARTESIAN_POINT('Ctrl Pts',(-9.49022236587123,2.27952295635682,10.6144401094098));
#91186=CARTESIAN_POINT('Ctrl Pts',(-9.43464957319556,-2.49958654445917,
10.6931769226868));
#91187=CARTESIAN_POINT('Ctrl Pts',(-7.11669761495095,-6.67930838632205,
10.7719137359637));
#91188=CARTESIAN_POINT('Ctrl Pts',(-3.09219913509919,-9.25736733478436,
10.8506505492407));
#91189=CARTESIAN_POINT('Ctrl Pts',(1.67379237475489,-9.61555846264028,10.9293873625177));
#91190=CARTESIAN_POINT('Ctrl Pts',(6.03841730848384,-7.66798942819062,11.0081241757946));
#91191=CARTESIAN_POINT('Ctrl Pts',(8.95506164624695,-3.88167700538795,11.0868609890716));
#91192=CARTESIAN_POINT('Ctrl Pts',(9.72432947175317,0.835441073345797,11.1655978023486));
#91193=CARTESIAN_POINT('Ctrl Pts',(8.16175442113116,5.35222479268075,11.2443346156255));
#91194=CARTESIAN_POINT('Ctrl Pts',(4.64203374325474,8.58557325917873,11.3230714289025));
#91195=CARTESIAN_POINT('Ctrl Pts',(0.00917787735352807,9.76014657824398,
11.4018082421795));
#91196=CARTESIAN_POINT('Ctrl Pts',(-4.62587879509039,8.59428826811001,11.4805450554565));
#91197=CARTESIAN_POINT('Ctrl Pts',(-8.15167415080322,5.36756499740499,11.5592818687334));
#91198=CARTESIAN_POINT('Ctrl Pts',(-9.72274107487621,0.853727973745442,
11.6380186820104));
#91199=CARTESIAN_POINT('Ctrl Pts',(-8.96234601200748,-3.8648285114988,11.7167554952874));
#91200=CARTESIAN_POINT('Ctrl Pts',(-6.05282768442402,-7.65661952070957,
11.7954923085644));
#91201=CARTESIAN_POINT('Ctrl Pts',(-1.69187322879139,-9.61239358536361,
11.8742291218413));
#91202=CARTESIAN_POINT('Ctrl Pts',(3.07478349632207,-9.26316640857683,11.9529659351183));
#91203=CARTESIAN_POINT('Ctrl Pts',(7.10412336968115,-6.6926808238994,12.0317027483953));
#91204=CARTESIAN_POINT('Ctrl Pts',(9.4299319590739,-2.51732570587861,12.1104395616723));
#91205=CARTESIAN_POINT('Ctrl Pts',(9.49449264186152,2.26167082836512,12.1891763749493));
#91206=CARTESIAN_POINT('Ctrl Pts',(7.28232410710392,6.49833063650456,12.2679131882262));
#91207=CARTESIAN_POINT('Ctrl Pts',(3.32389269220285,9.17672506033395,12.3466500015032));
#91208=CARTESIAN_POINT('Ctrl Pts',(-1.43159064466794,9.65458925528889,12.4253868147802));
#91209=CARTESIAN_POINT('Ctrl Pts',(-5.84378610179361,7.81733390989052,12.5041236280571));
#91210=CARTESIAN_POINT('Ctrl Pts',(-8.85467249893046,4.10552315776266,12.5828604413341));
#91211=CARTESIAN_POINT('Ctrl Pts',(-9.74225517141907,-0.590770376033278,
12.6615972546111));
#91212=CARTESIAN_POINT('Ctrl Pts',(-8.29369647962288,-5.14540029211835,
12.7403340678881));
#91213=CARTESIAN_POINT('Ctrl Pts',(-4.85635315142008,-8.46619037885003,
12.819070881165));
#91214=CARTESIAN_POINT('Ctrl Pts',(-0.254481972428574,-9.75683270267301,
12.897807694442));
#91215=CARTESIAN_POINT('Ctrl Pts',(4.40841264023357,-8.70783804716588,12.976544507719));
#91216=CARTESIAN_POINT('Ctrl Pts',(8.01419317217444,-5.57074979345805,13.0552813209959));
#91217=CARTESIAN_POINT('Ctrl Pts',(9.6982124854386,-1.09782514524086,13.1340181342729));
#91218=CARTESIAN_POINT('Ctrl Pts',(9.05665163803072,3.63835217778546,13.2127549475499));
#91219=CARTESIAN_POINT('Ctrl Pts',(6.24335353459279,7.50207185411658,13.2914917608269));
#91220=CARTESIAN_POINT('Ctrl Pts',(1.93293220995191,9.56683430053906,13.3702285741039));
#91221=CARTESIAN_POINT('Ctrl Pts',(-2.84099605538939,9.33752038153078,13.4489653873808));
#91222=CARTESIAN_POINT('Ctrl Pts',(-6.93366846323316,6.86911836440503,13.5277022006578));
#91223=CARTESIAN_POINT('Ctrl Pts',(-9.36368377390736,2.75353802307226,13.6064390139348));
#91224=CARTESIAN_POINT('Ctrl Pts',(-9.54833714307926,-2.02232620126758,
13.6851758272117));
#91225=CARTESIAN_POINT('Ctrl Pts',(-7.44334966753948,-6.31324727766785,
13.7639126404887));
#91226=CARTESIAN_POINT('Ctrl Pts',(-3.55348623245917,-9.0902849822194,13.8426494537657));
#91227=CARTESIAN_POINT('Ctrl Pts',(1.18848444360352,-9.68752033234268,13.9213862670427));
#91228=CARTESIAN_POINT('Ctrl Pts',(5.6454628236672,-7.96173944366632,14.0001230803196));
#91229=CARTESIAN_POINT('Ctrl Pts',(8.74868901896026,-4.32677546352531,14.0788598935966));
#91230=CARTESIAN_POINT('Ctrl Pts',(9.75402576865375,0.345726433295193,14.1575967068736));
#91231=CARTESIAN_POINT('Ctrl Pts',(8.42039862697821,4.93532495637561,14.2363335201505));
#91232=CARTESIAN_POINT('Ctrl Pts',(5.06760434277485,8.34145860670244,14.3150703334275));
#91233=CARTESIAN_POINT('Ctrl Pts',(0.499625287214116,9.7473545146679,14.3938071467045));
#91234=CARTESIAN_POINT('Ctrl Pts',(-4.1881612748804,8.81588626275501,14.4725439599815));
#91235=CARTESIAN_POINT('Ctrl Pts',(-7.87164887103858,5.77041502089042,14.5512807732584));
#91236=CARTESIAN_POINT('Ctrl Pts',(-9.6675566194929,1.34122871693821,14.6300175865354));
#91237=CARTESIAN_POINT('Ctrl Pts',(-9.14523532210772,-3.40957715347724,
14.7087543998124));
#91238=CARTESIAN_POINT('Ctrl Pts',(-6.4299348688519,-7.3427844204064,14.7874912130894));
#91239=CARTESIAN_POINT('Ctrl Pts',(-2.17276997533279,-9.51523074321021,
14.8662280263663));
#91240=CARTESIAN_POINT('Ctrl Pts',(2.60541368900876,-9.4059749612343,14.9449648396433));
#91241=CARTESIAN_POINT('Ctrl Pts',(6.75883290375718,-7.04121603427487,15.0237016529203));
#91242=CARTESIAN_POINT('Ctrl Pts',(9.29151966560509,-2.98801067031467,15.1024384661973));
#91243=CARTESIAN_POINT('Ctrl Pts',(9.59614905819356,1.78170387976553,15.1811752794742));
#91244=CARTESIAN_POINT('Ctrl Pts',(7.59967256120758,6.12417524444471,15.2599120927512));
#91245=CARTESIAN_POINT('Ctrl Pts',(3.78083469995116,8.99810171279953,15.3386489060282));
#91246=CARTESIAN_POINT('Ctrl Pts',(-0.944627364702379,9.71433088813101,
15.4173857193052));
#91247=CARTESIAN_POINT('Ctrl Pts',(-5.44357277364452,8.10111479490791,15.4961225325821));
#91248=CARTESIAN_POINT('Ctrl Pts',(-8.63717816610739,4.54529413670439,15.5748593458591));
#91249=CARTESIAN_POINT('Ctrl Pts',(-9.75963382685953,-0.100464062526747,
15.6535961591361));
#91250=CARTESIAN_POINT('Ctrl Pts',(-8.54178081348788,-4.7221315098765,15.7323329724131));
#91251=CARTESIAN_POINT('Ctrl Pts',(-5.27565384999563,-8.21145674757389,
15.81106978569));
#91252=CARTESIAN_POINT('Ctrl Pts',(-0.744452941532393,-9.7317180024937,
15.889806598967));
#91253=CARTESIAN_POINT('Ctrl Pts',(3.96526385261457,-8.91836465062037,15.968543412244));
#91254=CARTESIAN_POINT('Ctrl Pts',(7.72413130608901,-5.96643453232091,16.0472802255209));
#91255=CARTESIAN_POINT('Ctrl Pts',(9.63079284524497,-1.5837849078288,16.1260170387979));
#91256=CARTESIAN_POINT('Ctrl Pts',(9.22804109755958,3.17864797737543,16.2047538520749));
#91257=CARTESIAN_POINT('Ctrl Pts',(6.61245380615948,7.17885785645543,16.2834906653519));
#91258=CARTESIAN_POINT('Ctrl Pts',(2.41123499676581,9.45761551628439,16.3622274786288));
#91259=CARTESIAN_POINT('Ctrl Pts',(-2.36818523679073,9.46848689833435,16.4409642919058));
#91260=CARTESIAN_POINT('Ctrl Pts',(-6.57972715140979,7.2088651034173,16.5197011051828));
#91261=CARTESIAN_POINT('Ctrl Pts',(-9.21348522699762,3.22059550860017,16.5984379184598));
#91262=CARTESIAN_POINT('Ctrl Pts',(-9.63789818000097,-1.53995588673697,
16.6771747317367));
#91263=CARTESIAN_POINT('Ctrl Pts',(-7.75119402398696,-5.93123399335623,
16.7559115450137));
#91264=CARTESIAN_POINT('Ctrl Pts',(-4.00579445755397,-8.90023348932953,
16.8346483582907));
#91265=CARTESIAN_POINT('Ctrl Pts',(0.700173476219099,-9.73500399091671,
16.9133851715676));
#91266=CARTESIAN_POINT('Ctrl Pts',(5.23824350334795,-8.23537189342328,16.9921219848446));
#91267=CARTESIAN_POINT('Ctrl Pts',(8.52021039499149,-4.76094114485073,17.0708587981216));
#91268=CARTESIAN_POINT('Ctrl Pts',(9.75907579768703,-0.144861729604177,
17.1495956113986));
#91269=CARTESIAN_POINT('Ctrl Pts',(8.65776636067038,4.50595454758523,17.2283324246755));
#91270=CARTESIAN_POINT('Ctrl Pts',(5.48037020895889,8.07626712887417,17.3070692379525));
#91271=CARTESIAN_POINT('Ctrl Pts',(0.988810292674002,9.70993267087064,17.3858060512295));
#91272=CARTESIAN_POINT('Ctrl Pts',(-3.7398612725716,9.01520919170358,17.4645428645065));
#91273=CARTESIAN_POINT('Ctrl Pts',(-7.5717335349507,6.15868307487187,17.5432796777834));
#91274=CARTESIAN_POINT('Ctrl Pts',(-9.58794466754864,1.8253432054014,17.6220164910604));
#91275=CARTESIAN_POINT('Ctrl Pts',(-9.30501610941416,-2.94571585148694,
17.7007533043374));
#91276=CARTESIAN_POINT('Ctrl Pts',(-6.79079607722315,-7.01038544384477,
17.7794901176143));
#91277=CARTESIAN_POINT('Ctrl Pts',(-2.64817458584047,-9.39404497645205,
17.8582269308913));
#91278=CARTESIAN_POINT('Ctrl Pts',(2.12945664534019,-9.52497797990943,17.9369637441683));
#91279=CARTESIAN_POINT('Ctrl Pts',(6.39647199028245,-7.37203480962839,18.0157005574453));
#91280=CARTESIAN_POINT('Ctrl Pts',(9.12961500426467,-3.45099933936275,18.0944373707222));
#91281=CARTESIAN_POINT('Ctrl Pts',(9.6735863678373,1.29694674406767,18.1731741839992));
#91282=CARTESIAN_POINT('Ctrl Pts',(7.89776743898533,5.73514941099307,18.2519109972762));
#91283=CARTESIAN_POINT('Ctrl Pts',(5.45144640470055,7.77513528065193,18.3044022061275));
#91284=CARTESIAN_POINT('Ctrl Pts',(4.05890223941934,8.44447259753758,18.3306478105532));
#91285=CARTESIAN_POINT('',(5.44054447803332,-7.62915214953083,18.0000585632373));
#91286=CARTESIAN_POINT('Ctrl Pts',(5.44060438077288,-7.62923406419748,18.));
#91287=CARTESIAN_POINT('Ctrl Pts',(5.63908049858948,-7.49661732771331,18.));
#91288=CARTESIAN_POINT('Ctrl Pts',(5.83209798667451,-7.356661156938,18.));
#91289=CARTESIAN_POINT('Ctrl Pts',(6.01921567302457,-7.20964694412941,18.));
#91290=CARTESIAN_POINT('Ctrl Pts',(6.06606615359304,-7.17283756146319,18.));
#91291=CARTESIAN_POINT('Ctrl Pts',(6.11254669610509,-7.1355854670293,18.));
#91292=CARTESIAN_POINT('Ctrl Pts',(6.15865019795423,-7.09789459962803,18.));
#91293=CARTESIAN_POINT('Ctrl Pts',(6.34251836556963,-6.94757736889825,18.));
#91294=CARTESIAN_POINT('Ctrl Pts',(6.52039177856815,-6.79028495952252,18.));
#91295=CARTESIAN_POINT('Ctrl Pts',(6.69202469675709,-6.62649321917725,18.));
#91296=CARTESIAN_POINT('Ctrl Pts',(6.86398651234873,-6.46238760735236,18.));
#91297=CARTESIAN_POINT('Ctrl Pts',(7.0296843088185,-6.29175722463819,18.));
#91298=CARTESIAN_POINT('Ctrl Pts',(7.1888389091338,-6.11503780430435,18.));
#91299=CARTESIAN_POINT('Ctrl Pts',(7.34753690632627,-5.93882537930102,18.));
#91300=CARTESIAN_POINT('Ctrl Pts',(7.49972959262976,-5.75655827630888,18.));
#91301=CARTESIAN_POINT('Ctrl Pts',(7.64510234867658,-5.56863371957282,18.));
#91302=CARTESIAN_POINT('Ctrl Pts',(7.71778872669999,-5.47467144120479,18.));
#91303=CARTESIAN_POINT('Ctrl Pts',(7.7887694932955,-5.37929430472954,18.));
#91304=CARTESIAN_POINT('Ctrl Pts',(7.85800127979533,-5.28254931711788,18.));
#91305=CARTESIAN_POINT('Ctrl Pts',(7.89298282651811,-5.23366585656554,18.));
#91306=CARTESIAN_POINT('Ctrl Pts',(7.92751779717385,-5.18443314532346,18.));
#91307=CARTESIAN_POINT('Ctrl Pts',(7.96160031305259,-5.13485710286307,18.));
#91308=CARTESIAN_POINT('Ctrl Pts',(7.97841946488067,-5.11039215467253,18.));
#91309=CARTESIAN_POINT('Ctrl Pts',(7.99512842932023,-5.08584359508419,18.));
#91310=CARTESIAN_POINT('Ctrl Pts',(8.01172648209115,-5.06121212757392,18.));
#91311=CARTESIAN_POINT('Ctrl Pts',(8.02805976181813,-5.03697358257809,18.));
#91312=CARTESIAN_POINT('Ctrl Pts',(8.04428165797018,-5.01266061493114,18.));
#91313=CARTESIAN_POINT('Ctrl Pts',(8.06038683280492,-4.9882814087714,18.));
#91314=CARTESIAN_POINT('Ctrl Pts',(8.19275521184893,-4.78790879345619,18.));
#91315=CARTESIAN_POINT('Ctrl Pts',(8.31734444140616,-4.58291260001262,18.));
#91316=CARTESIAN_POINT('Ctrl Pts',(8.43390799998684,-4.37375983102443,18.));
#91317=CARTESIAN_POINT('Ctrl Pts',(8.55097522304311,-4.16370332487345,18.));
#91318=CARTESIAN_POINT('Ctrl Pts',(8.65994769799928,-3.94945372966206,18.));
#91319=CARTESIAN_POINT('Ctrl Pts',(8.76053783217777,-3.73144799113718,18.));
#91320=CARTESIAN_POINT('Ctrl Pts',(8.8154658148089,-3.61240435413465,18.));
#91321=CARTESIAN_POINT('Ctrl Pts',(8.8678936654753,-3.49224013192352,18.));
#91322=CARTESIAN_POINT('Ctrl Pts',(8.91776911684323,-3.3710227923076,18.));
#91323=CARTESIAN_POINT('Ctrl Pts',(9.00877320867449,-3.14984636977119,18.));
#91324=CARTESIAN_POINT('Ctrl Pts',(9.09128260143624,-2.92516487707576,18.));
#91325=CARTESIAN_POINT('Ctrl Pts',(9.16525623050192,-2.69748761681311,18.));
#91326=CARTESIAN_POINT('Ctrl Pts',(9.23941857399464,-2.4692295281625,18.));
#91327=CARTESIAN_POINT('Ctrl Pts',(9.3050016942559,-2.23795972868455,18.));
#91328=CARTESIAN_POINT('Ctrl Pts',(9.36191409108156,-2.00417709010597,18.));
#91329=CARTESIAN_POINT('Ctrl Pts',(9.38858160860227,-1.89463324802476,18.));
#91330=CARTESIAN_POINT('Ctrl Pts',(9.41334466163771,-1.78453754436346,18.));
#91331=CARTESIAN_POINT('Ctrl Pts',(9.43618992040111,-1.67394083647048,18.));
#91332=CARTESIAN_POINT('Ctrl Pts',(9.4414550134228,-1.64845187348782,18.));
#91333=CARTESIAN_POINT('Ctrl Pts',(9.44661801742425,-1.62293716459345,18.));
#91334=CARTESIAN_POINT('Ctrl Pts',(9.4516763764568,-1.59740995483373,18.));
#91335=CARTESIAN_POINT('Ctrl Pts',(9.49875085486108,-1.35984672991766,18.));
#91336=CARTESIAN_POINT('Ctrl Pts',(9.53682634772605,-1.12091537343081,18.));
#91337=CARTESIAN_POINT('Ctrl Pts',(9.56592491913746,-0.881154213382847,
18.));
#91338=CARTESIAN_POINT('Ctrl Pts',(9.59514317894571,-0.640406866471459,
18.));
#91339=CARTESIAN_POINT('Ctrl Pts',(9.61531064791162,-0.39882222764125,18.));
#91340=CARTESIAN_POINT('Ctrl Pts',(9.62640020763537,-0.156925741005529,
18.));
#91341=CARTESIAN_POINT('Ctrl Pts',(9.637454051899,0.0841916845548948,18.));
#91342=CARTESIAN_POINT('Ctrl Pts',(9.63948844587604,0.325619611769683,18.));
#91343=CARTESIAN_POINT('Ctrl Pts',(9.63242601287159,0.566847217814661,18.));
#91344=CARTESIAN_POINT('Ctrl Pts',(9.62540501294608,0.806659617168582,18.));
#91345=CARTESIAN_POINT('Ctrl Pts',(9.60939367539977,1.04627467889501,18.));
#91346=CARTESIAN_POINT('Ctrl Pts',(9.58426491595667,1.28519029797862,18.));
#91347=CARTESIAN_POINT('Ctrl Pts',(9.55893834752381,1.5259866170369,18.));
#91348=CARTESIAN_POINT('Ctrl Pts',(9.52435004681638,1.76607306295997,18.));
#91349=CARTESIAN_POINT('Ctrl Pts',(9.48065298058511,2.00496676972802,18.));
#91350=CARTESIAN_POINT('Ctrl Pts',(9.47776845394166,2.02073659872469,18.));
#91351=CARTESIAN_POINT('Ctrl Pts',(9.47484421719539,2.03650122469258,18.));
#91352=CARTESIAN_POINT('Ctrl Pts',(9.47188030676458,2.05226050618878,18.));
#91353=CARTESIAN_POINT('Ctrl Pts',(9.46699294616702,2.07824688237274,18.));
#91354=CARTESIAN_POINT('Ctrl Pts',(9.46199776850117,2.10421821966082,18.));
#91355=CARTESIAN_POINT('Ctrl Pts',(9.45689766603046,2.13016061400735,18.));
#91356=CARTESIAN_POINT('Ctrl Pts',(9.41044452583058,2.36645109809496,18.));
#91357=CARTESIAN_POINT('Ctrl Pts',(9.35523815544362,2.6006253577108,18.));
#91358=CARTESIAN_POINT('Ctrl Pts',(9.29156327949617,2.83223149451236,18.));
#91359=CARTESIAN_POINT('Ctrl Pts',(9.22550315875267,3.07251353879421,18.));
#91360=CARTESIAN_POINT('Ctrl Pts',(9.15032830215148,3.31003211717532,18.));
#91361=CARTESIAN_POINT('Ctrl Pts',(9.06629873032425,3.5442816002362,18.));
#91362=CARTESIAN_POINT('Ctrl Pts',(8.98378308036435,3.77431071888128,18.));
#91363=CARTESIAN_POINT('Ctrl Pts',(8.89272851982826,4.00118809602247,18.));
#91364=CARTESIAN_POINT('Ctrl Pts',(8.79332932928383,4.22442436011723,18.));
#91365=CARTESIAN_POINT('Ctrl Pts',(8.69119461023845,4.45380422718833,18.));
#91366=CARTESIAN_POINT('Ctrl Pts',(8.58024964935816,4.67934061636778,18.));
#91367=CARTESIAN_POINT('Ctrl Pts',(8.46065218408456,4.90048044154929,18.));
#91368=CARTESIAN_POINT('Ctrl Pts',(8.34105471881097,5.12162026673081,18.));
#91369=CARTESIAN_POINT('Ctrl Pts',(8.21280451965211,5.33836427804101,18.));
#91370=CARTESIAN_POINT('Ctrl Pts',(8.07600905803291,5.55012586177464,18.));
#91371=CARTESIAN_POINT('Ctrl Pts',(8.06012001225815,5.57472236123051,18.));
#91372=CARTESIAN_POINT('Ctrl Pts',(8.04411564478489,5.59925148901493,18.));
#91373=CARTESIAN_POINT('Ctrl Pts',(8.02800402746578,5.62370047380093,18.));
#91374=CARTESIAN_POINT('Ctrl Pts',(7.99747825883122,5.67002258027512,18.));
#91375=CARTESIAN_POINT('Ctrl Pts',(7.96656056320155,5.71606781954641,18.));
#91376=CARTESIAN_POINT('Ctrl Pts',(7.93525343239553,5.76183067239227,18.));
#91377=CARTESIAN_POINT('Ctrl Pts',(7.79770776576771,5.96288653217314,18.));
#91378=CARTESIAN_POINT('Ctrl Pts',(7.65264895522489,6.15849356205626,18.));
#91379=CARTESIAN_POINT('Ctrl Pts',(7.50052757437793,6.34837497204547,18.));
#91380=CARTESIAN_POINT('Ctrl Pts',(7.34701857641731,6.53998843766418,18.));
#91381=CARTESIAN_POINT('Ctrl Pts',(7.18631717033013,6.72577182484101,18.));
#91382=CARTESIAN_POINT('Ctrl Pts',(7.01884082387205,6.90541294124557,18.));
#91383=CARTESIAN_POINT('Ctrl Pts',(6.92175824280081,7.00954718835513,18.));
#91384=CARTESIAN_POINT('Ctrl Pts',(6.82239827758366,7.11161690764809,18.));
#91385=CARTESIAN_POINT('Ctrl Pts',(6.72083616319641,7.21155611066385,18.));
#91386=CARTESIAN_POINT('Ctrl Pts',(6.66929208915534,7.26227653639473,18.));
#91387=CARTESIAN_POINT('Ctrl Pts',(6.617180742554,7.31244814185575,18.));
#91388=CARTESIAN_POINT('Ctrl Pts',(6.56451156701509,7.36206188025258,18.));
#91389=CARTESIAN_POINT('Ctrl Pts',(6.52219163648823,7.40192675264994,18.));
#91390=CARTESIAN_POINT('Ctrl Pts',(6.47951155539951,7.44143144973857,18.));
#91391=CARTESIAN_POINT('Ctrl Pts',(6.43647610849305,7.48057113719609,18.));
#91392=CARTESIAN_POINT('Ctrl Pts',(6.40510030277937,7.50910666587389,18.));
#91393=CARTESIAN_POINT('Ctrl Pts',(6.37353721864763,7.53744658432229,18.));
#91394=CARTESIAN_POINT('Ctrl Pts',(6.34180463558981,7.56557530387894,18.));
#91395=CARTESIAN_POINT('Ctrl Pts',(6.28236444622681,7.61826488209385,18.));
#91396=CARTESIAN_POINT('Ctrl Pts',(6.22231565827699,7.67022618764865,18.));
#91397=CARTESIAN_POINT('Ctrl Pts',(6.16167255213736,7.72144997951763,18.));
#91398=CARTESIAN_POINT('Ctrl Pts',(5.97233596776844,7.88137809679721,18.));
#91399=CARTESIAN_POINT('Ctrl Pts',(5.77721063648874,8.03411825327571,18.));
#91400=CARTESIAN_POINT('Ctrl Pts',(5.57671927434662,8.17935389220667,18.));
#91401=CARTESIAN_POINT('Ctrl Pts',(5.37540325211635,8.32518691365587,18.));
#91402=CARTESIAN_POINT('Ctrl Pts',(5.16867649244539,8.46345403723429,18.));
#91403=CARTESIAN_POINT('Ctrl Pts',(4.95693127547179,8.59379583228999,18.));
#91404=CARTESIAN_POINT('Ctrl Pts',(4.7451860584982,8.7241376273457,18.));
#91405=CARTESIAN_POINT('Ctrl Pts',(4.52842188794294,8.84655456454867,18.));
#91406=CARTESIAN_POINT('Ctrl Pts',(4.30700275658802,8.96064123010977,18.));
#91407=CARTESIAN_POINT('Ctrl Pts',(5.43505795426094,-7.63293718671423,18.));
#91408=CARTESIAN_POINT('Ctrl Pts',(5.43686761498028,-7.63164861186465,18.0000195210791));
#91409=CARTESIAN_POINT('Ctrl Pts',(5.43867681744549,-7.63035939344787,18.0000390421582));
#91410=CARTESIAN_POINT('Ctrl Pts',(5.44048556119893,-7.62906953178997,18.0000585632373));
#91411=CARTESIAN_POINT('Ctrl Pts',(4.30729780905827,8.96073832123217,4.));
#91412=CARTESIAN_POINT('Ctrl Pts',(4.52735866241683,8.84762889800062,3.99999999999999));
#91413=CARTESIAN_POINT('Ctrl Pts',(4.74289519135029,8.72644163152856,3.99999999999999));
#91414=CARTESIAN_POINT('Ctrl Pts',(4.95341780643153,8.59733634854351,3.99999999999999));
#91415=CARTESIAN_POINT('Ctrl Pts',(5.01139145305849,8.5617833793266,3.99999999999999));
#91416=CARTESIAN_POINT('Ctrl Pts',(5.06898473711946,8.52562968458252,4.));
#91417=CARTESIAN_POINT('Ctrl Pts',(5.12618709348549,8.48887799458869,4.));
#91418=CARTESIAN_POINT('Ctrl Pts',(5.33414451424221,8.35526834727518,3.99999999999999));
#91419=CARTESIAN_POINT('Ctrl Pts',(5.53693773709606,8.21375835063172,4.));
#91420=CARTESIAN_POINT('Ctrl Pts',(5.73421561007242,8.06474571286238,3.99999999999999));
#91421=CARTESIAN_POINT('Ctrl Pts',(5.93164891033915,7.91561567403752,3.99999999999999));
#91422=CARTESIAN_POINT('Ctrl Pts',(6.12355862014355,7.75897067554847,4.));
#91423=CARTESIAN_POINT('Ctrl Pts',(6.30955580572295,7.5951727274196,4.));
#91424=CARTESIAN_POINT('Ctrl Pts',(6.34223834170209,7.56639093528467,4.));
#91425=CARTESIAN_POINT('Ctrl Pts',(6.37473822150666,7.53738820927742,4.));
#91426=CARTESIAN_POINT('Ctrl Pts',(6.40705320087122,7.50816641433773,4.));
#91427=CARTESIAN_POINT('Ctrl Pts',(6.43174166095423,7.48584112952835,4.));
#91428=CARTESIAN_POINT('Ctrl Pts',(6.45631548500609,7.46339403274824,4.));
#91429=CARTESIAN_POINT('Ctrl Pts',(6.48077183163878,7.44082803617405,4.));
#91430=CARTESIAN_POINT('Ctrl Pts',(6.63832117297785,7.2954564502082,4.));
#91431=CARTESIAN_POINT('Ctrl Pts',(6.79102402996194,7.14512773488293,4.));
#91432=CARTESIAN_POINT('Ctrl Pts',(6.93866063600344,6.99010918328356,4.));
#91433=CARTESIAN_POINT('Ctrl Pts',(7.10847998508006,6.81179873417987,4.));
#91434=CARTESIAN_POINT('Ctrl Pts',(7.27159731884034,6.62728364575909,4.));
#91435=CARTESIAN_POINT('Ctrl Pts',(7.42764239363171,6.43693772257308,4.00000000000001));
#91436=CARTESIAN_POINT('Ctrl Pts',(7.58218650243463,6.24842269829321,4.00000000000001));
#91437=CARTESIAN_POINT('Ctrl Pts',(7.72979410893354,6.05418794787021,4.00000000000001));
#91438=CARTESIAN_POINT('Ctrl Pts',(7.87006275526019,5.85456913669398,4.00000000000001));
#91439=CARTESIAN_POINT('Ctrl Pts',(7.92865109023734,5.77119103272556,4.00000000000001));
#91440=CARTESIAN_POINT('Ctrl Pts',(7.98595850701148,5.6868733272343,4.00000000000001));
#91441=CARTESIAN_POINT('Ctrl Pts',(8.04195320620857,5.60163937017,4.00000000000001));
#91442=CARTESIAN_POINT('Ctrl Pts',(8.05864268878731,5.5762349897208,4.));
#91443=CARTESIAN_POINT('Ctrl Pts',(8.07521588798848,5.55074859303754,4.00000000000001));
#91444=CARTESIAN_POINT('Ctrl Pts',(8.09166333406113,5.525194394489,4.00000000000001));
#91445=CARTESIAN_POINT('Ctrl Pts',(8.20895789598644,5.34295524861398,4.00000000000001));
#91446=CARTESIAN_POINT('Ctrl Pts',(8.31996633523362,5.15710734281305,4.));
#91447=CARTESIAN_POINT('Ctrl Pts',(8.42446245528993,4.96791812226087,4.00000000000001));
#91448=CARTESIAN_POINT('Ctrl Pts',(8.5415709437287,4.75589433002977,4.00000000000001));
#91449=CARTESIAN_POINT('Ctrl Pts',(8.65050135921717,4.53967410763202,4.));
#91450=CARTESIAN_POINT('Ctrl Pts',(8.75117985411016,4.31977266478955,4.));
#91451=CARTESIAN_POINT('Ctrl Pts',(8.85287322430194,4.09765453661874,4.));
#91452=CARTESIAN_POINT('Ctrl Pts',(8.94614769538898,3.87177998411824,4.));
#91453=CARTESIAN_POINT('Ctrl Pts',(9.03087895681104,3.64265834953363,4.));
#91454=CARTESIAN_POINT('Ctrl Pts',(9.11548314304982,3.41388033869804,4.));
#91455=CARTESIAN_POINT('Ctrl Pts',(9.19156986905553,3.18186432688568,4.));
#91456=CARTESIAN_POINT('Ctrl Pts',(9.25896493253069,2.94710551021159,4.));
#91457=CARTESIAN_POINT('Ctrl Pts',(9.32561355021895,2.71494680578028,4.));
#91458=CARTESIAN_POINT('Ctrl Pts',(9.38376203708655,2.48010509232614,4.00000000000001));
#91459=CARTESIAN_POINT('Ctrl Pts',(9.43319110917098,2.24305718438921,4.));
#91460=CARTESIAN_POINT('Ctrl Pts',(9.44421566232366,2.19018653255259,4.));
#91461=CARTESIAN_POINT('Ctrl Pts',(9.45480625606057,2.13720614422637,4.));
#91462=CARTESIAN_POINT('Ctrl Pts',(9.46496010189184,2.08412134345432,4.));
#91463=CARTESIAN_POINT('Ctrl Pts',(9.47020198198243,2.05671653891976,4.));
#91464=CARTESIAN_POINT('Ctrl Pts',(9.47532601316739,2.0292913927946,4.));
#91465=CARTESIAN_POINT('Ctrl Pts',(9.48033096475668,2.00185258817826,4.));
#91466=CARTESIAN_POINT('Ctrl Pts',(9.52392327882317,1.76286506410242,4.));
#91467=CARTESIAN_POINT('Ctrl Pts',(9.55851334216252,1.52270096690633,4.00000000000001));
#91468=CARTESIAN_POINT('Ctrl Pts',(9.58400922469124,1.28186074651651,4.));
#91469=CARTESIAN_POINT('Ctrl Pts',(9.60946255717459,1.04142246405902,4.));
#91470=CARTESIAN_POINT('Ctrl Pts',(9.62585215468648,0.800309667757621,4.00000000000001));
#91471=CARTESIAN_POINT('Ctrl Pts',(9.63303576261776,0.559010656769312,4.00000000000001));
#91472=CARTESIAN_POINT('Ctrl Pts',(9.63493699332233,0.495147888497155,4.00000000000001));
#91473=CARTESIAN_POINT('Ctrl Pts',(9.63619309821743,0.431272053532241,4.));
#91474=CARTESIAN_POINT('Ctrl Pts',(9.63680082693735,0.367392178681336,4.));
#91475=CARTESIAN_POINT('Ctrl Pts',(9.63910369572888,0.125331921562864,4.00000000000001));
#91476=CARTESIAN_POINT('Ctrl Pts',(9.63210067711924,-0.116786870509174,
4.00000000000001));
#91477=CARTESIAN_POINT('Ctrl Pts',(9.61592042259555,-0.358453301654759,
4.00000000000001));
#91478=CARTESIAN_POINT('Ctrl Pts',(9.59976867571333,-0.599693945927636,
4.00000000000001));
#91479=CARTESIAN_POINT('Ctrl Pts',(9.57447182128881,-0.840484470113809,
4.));
#91480=CARTESIAN_POINT('Ctrl Pts',(9.54010755134981,-1.08030443174907,4.00000000000001));
#91481=CARTESIAN_POINT('Ctrl Pts',(9.52066457166946,-1.21599230317178,4.));
#91482=CARTESIAN_POINT('Ctrl Pts',(9.49831804338267,-1.35136920346387,4.00000000000001));
#91483=CARTESIAN_POINT('Ctrl Pts',(9.47307521435284,-1.4863379289703,4.00000000000001));
#91484=CARTESIAN_POINT('Ctrl Pts',(9.4649303911865,-1.52988678797252,4.00000000000001));
#91485=CARTESIAN_POINT('Ctrl Pts',(9.45648402016263,-1.57339303349641,4.00000000000001));
#91486=CARTESIAN_POINT('Ctrl Pts',(9.44773617789971,-1.61685363980245,4.00000000000001));
#91487=CARTESIAN_POINT('Ctrl Pts',(9.44045759216671,-1.653014756967,4.00000000000001));
#91488=CARTESIAN_POINT('Ctrl Pts',(9.4329703892861,-1.68914330368502,4.00000000000001));
#91489=CARTESIAN_POINT('Ctrl Pts',(9.42528051679276,-1.72521129584486,4.00000000000001));
#91490=CARTESIAN_POINT('Ctrl Pts',(9.37504487203195,-1.96083273728565,4.));
#91491=CARTESIAN_POINT('Ctrl Pts',(9.31610795885698,-2.19415568001356,4.));
#91492=CARTESIAN_POINT('Ctrl Pts',(9.24864539615387,-2.42469127009468,4.));
#91493=CARTESIAN_POINT('Ctrl Pts',(9.18110633204538,-2.65548828363685,4.));
#91494=CARTESIAN_POINT('Ctrl Pts',(9.10502208698088,-2.88349226619126,4.));
#91495=CARTESIAN_POINT('Ctrl Pts',(9.02051769106837,-3.10820223924067,4.));
#91496=CARTESIAN_POINT('Ctrl Pts',(8.93678495719486,-3.33086024618686,4.));
#91497=CARTESIAN_POINT('Ctrl Pts',(8.84478490227422,-3.55028471986832,4.));
#91498=CARTESIAN_POINT('Ctrl Pts',(8.7445922820912,-3.7659688277657,4.));
#91499=CARTESIAN_POINT('Ctrl Pts',(8.67781695430482,-3.90971571228528,4.));
#91500=CARTESIAN_POINT('Ctrl Pts',(8.60740168442632,-4.05180078366608,4.));
#91501=CARTESIAN_POINT('Ctrl Pts',(8.53335765314134,-4.19206717736045,4.));
#91502=CARTESIAN_POINT('Ctrl Pts',(8.44331101733595,-4.36264833899545,4.));
#91503=CARTESIAN_POINT('Ctrl Pts',(8.34789785964412,-4.53054022772032,4.));
#91504=CARTESIAN_POINT('Ctrl Pts',(8.24728117878015,-4.69552960580368,4.));
#91505=CARTESIAN_POINT('Ctrl Pts',(8.20326138090216,-4.76771245871515,4.));
#91506=CARTESIAN_POINT('Ctrl Pts',(8.15824539656185,-4.83933955682702,4.));
#91507=CARTESIAN_POINT('Ctrl Pts',(8.11224599398009,-4.91039207263641,4.));
#91508=CARTESIAN_POINT('Ctrl Pts',(8.08753260385713,-4.94856536280674,4.));
#91509=CARTESIAN_POINT('Ctrl Pts',(8.06253567255053,-4.9865723101471,4.));
#91510=CARTESIAN_POINT('Ctrl Pts',(8.03725606161742,-5.02441150090253,4.));
#91511=CARTESIAN_POINT('Ctrl Pts',(8.01764312895937,-5.05376865762798,4.));
#91512=CARTESIAN_POINT('Ctrl Pts',(7.9978615337744,-5.08302244104312,4.));
#91513=CARTESIAN_POINT('Ctrl Pts',(7.97792532987057,-5.11215275381745,4.));
#91514=CARTESIAN_POINT('Ctrl Pts',(7.8440295483756,-5.30779812406573,4.));
#91515=CARTESIAN_POINT('Ctrl Pts',(7.70302251457516,-5.49808894505449,4.));
#91516=CARTESIAN_POINT('Ctrl Pts',(7.55529935414448,-5.68269963489007,4.));
#91517=CARTESIAN_POINT('Ctrl Pts',(7.40624743847603,-5.86897087964711,4.));
#91518=CARTESIAN_POINT('Ctrl Pts',(7.25035761889544,-6.04945986263983,4.));
#91519=CARTESIAN_POINT('Ctrl Pts',(7.08799183256734,-6.22380270966777,4.));
#91520=CARTESIAN_POINT('Ctrl Pts',(6.92609832025987,-6.39763844495009,4.));
#91521=CARTESIAN_POINT('Ctrl Pts',(6.75776597786644,-6.56536420217669,4.));
#91522=CARTESIAN_POINT('Ctrl Pts',(6.58331694003355,-6.72658296228736,4.));
#91523=CARTESIAN_POINT('Ctrl Pts',(6.40972058594001,-6.88701370649991,4.));
#91524=CARTESIAN_POINT('Ctrl Pts',(6.23006671722395,-7.0410013431429,4.));
#91525=CARTESIAN_POINT('Ctrl Pts',(6.04464352038724,-7.18811202239736,4.));
#91526=CARTESIAN_POINT('Ctrl Pts',(5.85922032355054,-7.33522270165183,4.));
#91527=CARTESIAN_POINT('Ctrl Pts',(5.66802736285917,-7.47545689991215,4.));
#91528=CARTESIAN_POINT('Ctrl Pts',(5.47133023013366,-7.60833117514228,4.));
#91529=CARTESIAN_POINT('Ctrl Pts',(5.46100689439012,-7.61530486985696,4.));
#91530=CARTESIAN_POINT('Ctrl Pts',(5.45066839308308,-7.62225827926665,4.));
#91531=CARTESIAN_POINT('Ctrl Pts',(5.44031476324456,-7.62919132931685,4.));
#91532=CARTESIAN_POINT('Origin',(0.,0.,4.));
#91533=CARTESIAN_POINT('',(-14.,-1.71450551880629E-15,4.));
#91534=CARTESIAN_POINT('Origin',(0.,0.,4.));
#91535=CARTESIAN_POINT('Origin',(0.,0.,0.));
#91536=CARTESIAN_POINT('',(-14.,-1.71450551880629E-15,0.));
#91537=CARTESIAN_POINT('',(-14.,-1.71450551880629E-15,0.));
#91538=CARTESIAN_POINT('Origin',(0.,0.,0.));
#91539=CARTESIAN_POINT('Origin',(0.,0.,0.));
#91540=CARTESIAN_POINT('',(-5.,-6.12323399573677E-16,0.));
#91541=CARTESIAN_POINT('Origin',(0.,0.,0.));
#91542=CARTESIAN_POINT('',(-5.,-6.12323399573677E-16,18.));
#91543=CARTESIAN_POINT('',(-5.,-6.12323399573677E-16,0.));
#91544=CARTESIAN_POINT('Origin',(0.,0.,18.));
#91545=CARTESIAN_POINT('Origin',(0.,0.,18.));
#91546=CARTESIAN_POINT('Origin',(0.,0.,0.));
#94391=UNCERTAINTY_MEASURE_WITH_UNIT(LENGTH_MEASURE(0.01),#94413,
'DISTANCE_ACCURACY_VALUE',
'Maximum model space distance between geometric entities at asserted c
onnectivities');
#94394=UNCERTAINTY_MEASURE_WITH_UNIT(LENGTH_MEASURE(0.01),#94413,
'DISTANCE_ACCURACY_VALUE',
'Maximum model space distance between geometric entities at asserted c
onnectivities');
#94409=(
GEOMETRIC_REPRESENTATION_CONTEXT(3)
GLOBAL_UNCERTAINTY_ASSIGNED_CONTEXT((#94391))
GLOBAL_UNIT_ASSIGNED_CONTEXT((#94413,#94415,#94416))
REPRESENTATION_CONTEXT('','3D')
);
#94412=(
GEOMETRIC_REPRESENTATION_CONTEXT(3)
GLOBAL_UNCERTAINTY_ASSIGNED_CONTEXT((#94394))
GLOBAL_UNIT_ASSIGNED_CONTEXT((#94413,#94415,#94416))
REPRESENTATION_CONTEXT('','3D')
);
#94413=(
LENGTH_UNIT()
NAMED_UNIT(*)
SI_UNIT(.MILLI.,.METRE.)
);
#94415=(
NAMED_UNIT(*)
PLANE_ANGLE_UNIT()
SI_UNIT($,.RADIAN.)
);
#94416=(
NAMED_UNIT(*)
SI_UNIT($,.STERADIAN.)
SOLID_ANGLE_UNIT()
);
#94431=SHAPE_DEFINITION_REPRESENTATION(#94465,#94500);
#94465=PRODUCT_DEFINITION_SHAPE('',$,#94518);
#94500=SHAPE_REPRESENTATION('',(#8845),#94409);
#94503=PRODUCT_DEFINITION_CONTEXT('part definition',#94556,'design');
#94518=PRODUCT_DEFINITION('Cable entry body','Cable entry body',#94535,
#94503);
#94535=PRODUCT_DEFINITION_FORMATION('',$,#94572);
#94556=APPLICATION_CONTEXT(
'Core Data for Automotive Mechanical Design Process');
#94557=PRODUCT_CONTEXT('part definition',#94556,'mechanical');
#94572=PRODUCT('Cable entry body','Cable entry body',$,(#94557));
#94577=PRESENTATION_STYLE_ASSIGNMENT((#94584));
#94584=SURFACE_STYLE_USAGE(.BOTH.,#94591);
#94591=SURFACE_SIDE_STYLE('',(#94598));
#94598=SURFACE_STYLE_FILL_AREA(#94605);
#94605=FILL_AREA_STYLE('Opaque(104,114,127)',(#94612));
#94612=FILL_AREA_STYLE_COLOUR('Opaque(104,114,127)',#94619);
#94619=COLOUR_RGB('Opaque(104,114,127)',0.407843137254902,0.447058823529412,
0.498039215686275);
ENDSEC;
END-ISO-10303-21;
